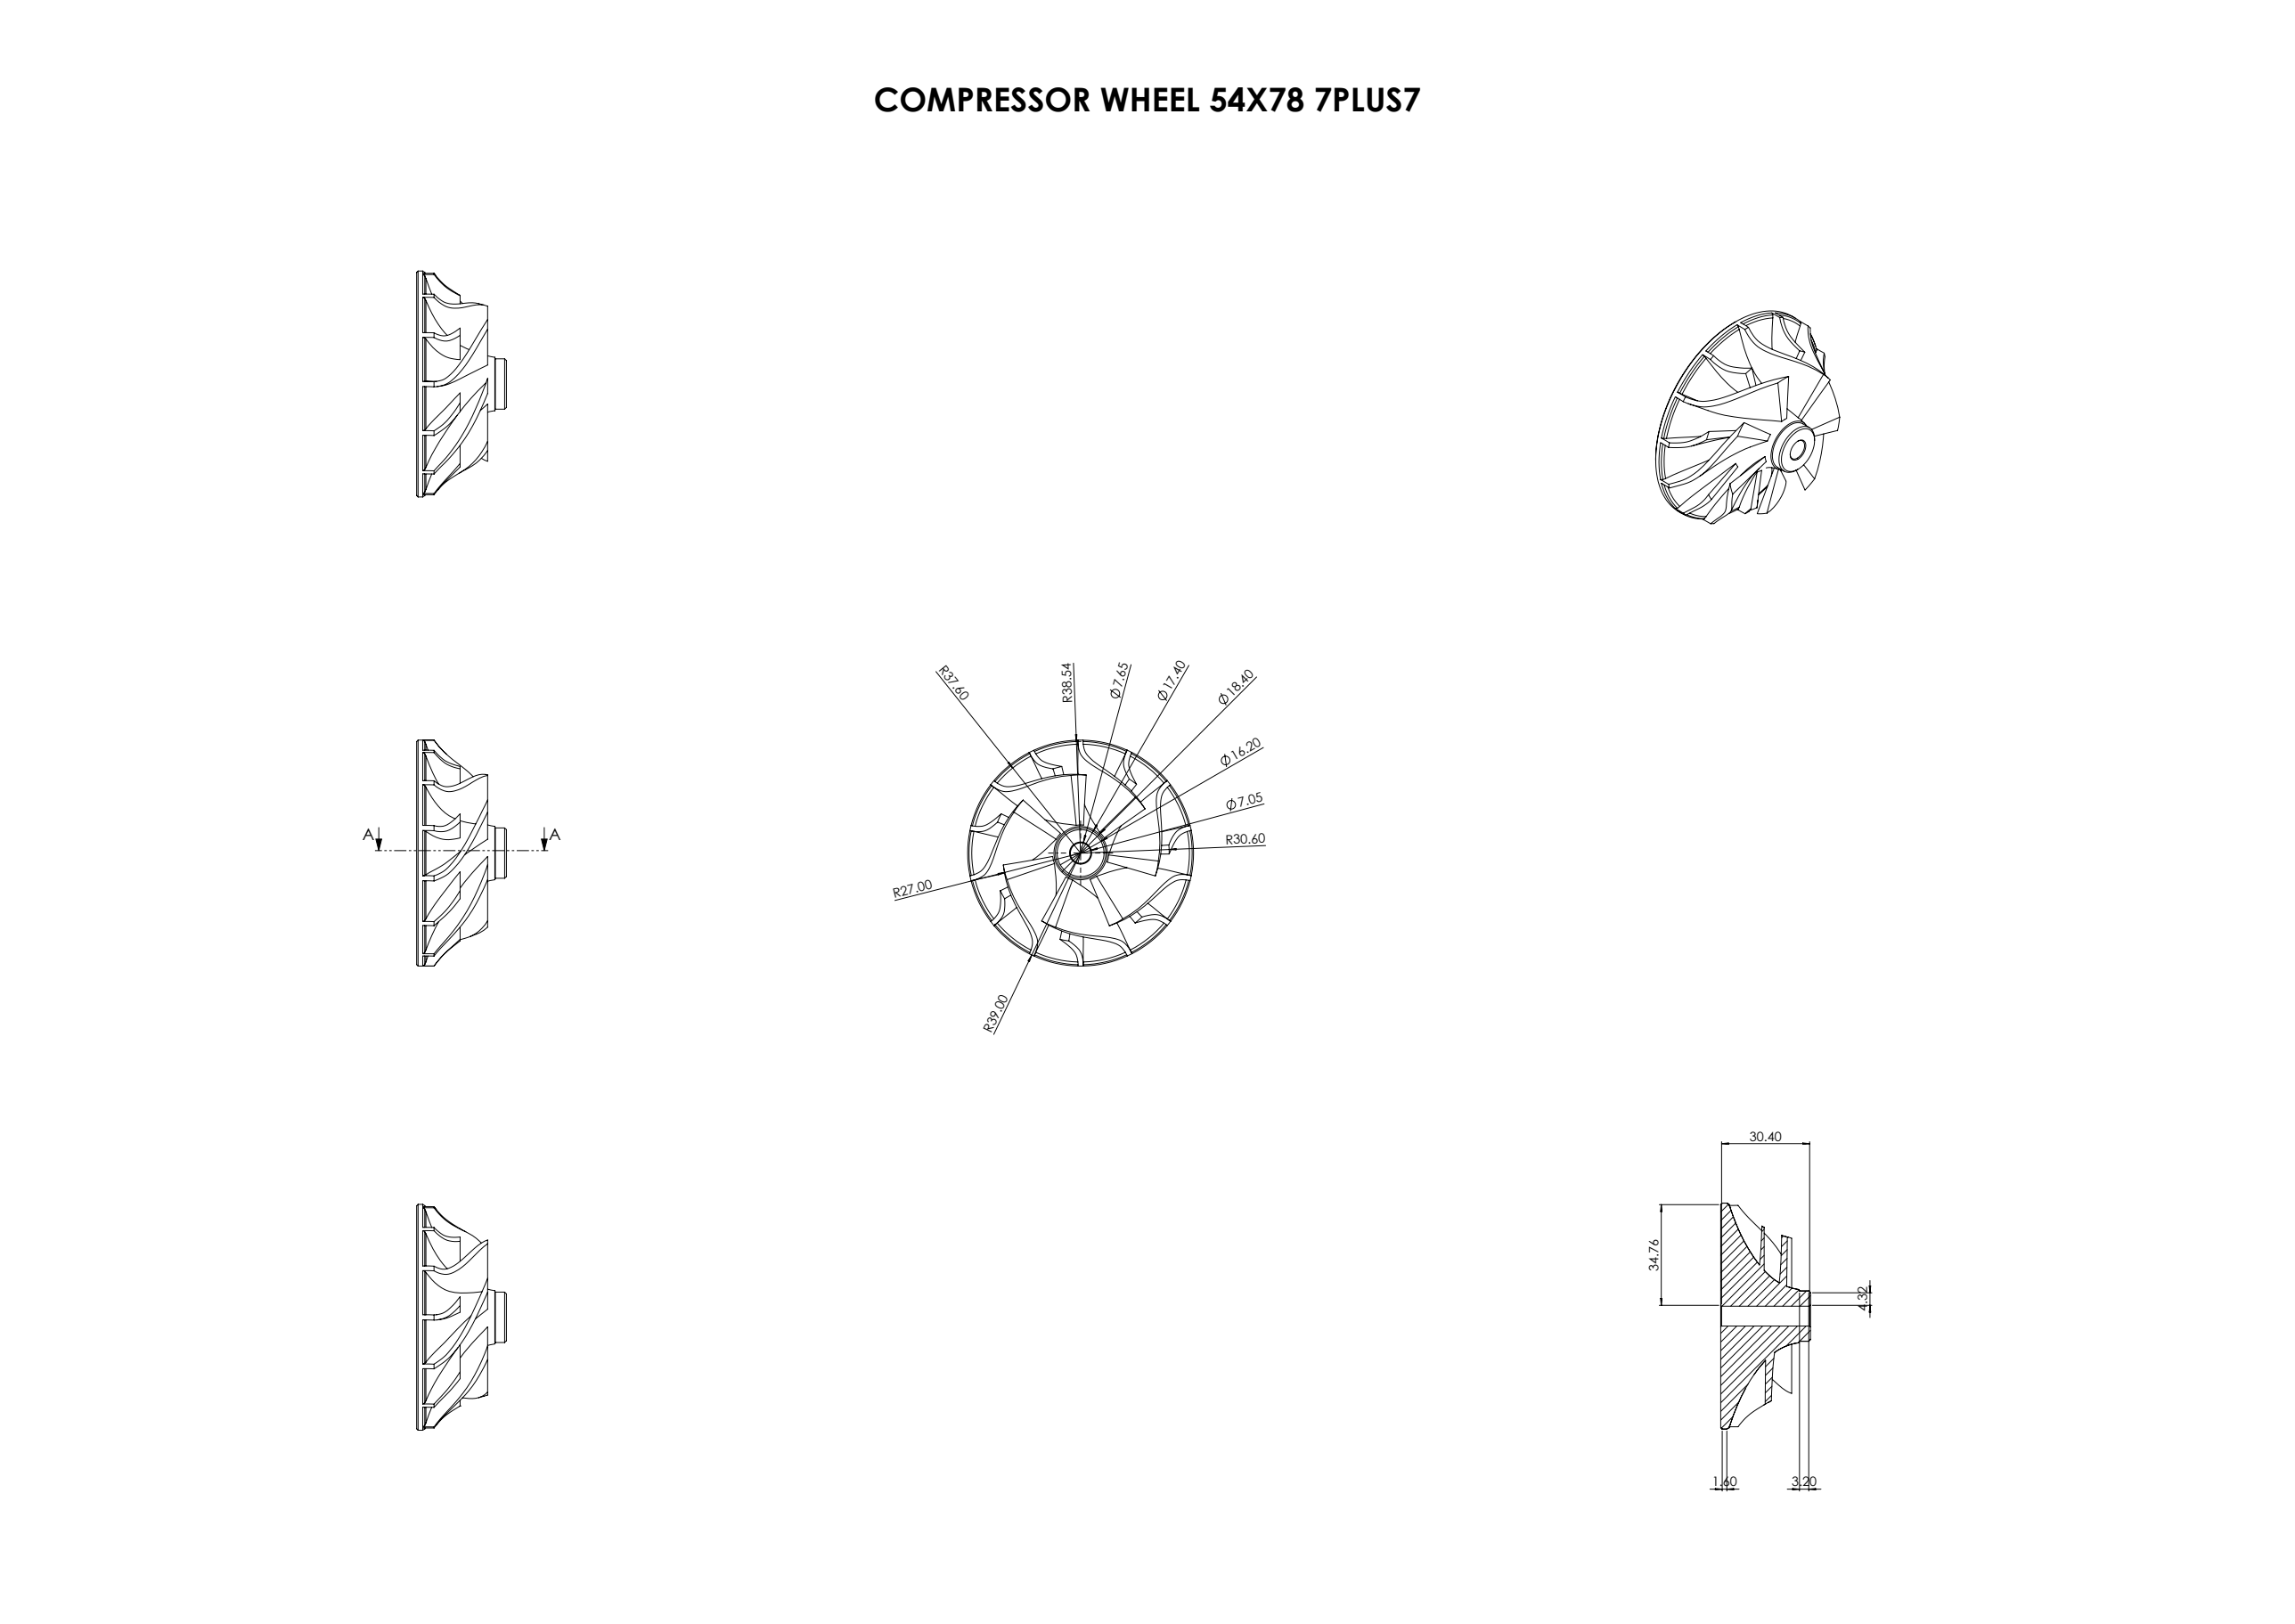
ISO-10303-21;
HEADER;
/* Generated by software containing ST-Developer
 * from STEP Tools, Inc. (www.steptools.com) 
 */

FILE_DESCRIPTION(
/* description */ (''),
/* implementation_level */ '2;1');

FILE_NAME(
/* name */ '09_Compressor_Wheel_54x78_7plus7.step',
/* time_stamp */ '2026-10-25T01:10:36-07:00',
/* author */ (''),
/* organization */ (''),
/* preprocessor_version */ 'ST-DEVELOPER v20.2',
/* originating_system */ 'Autodesk Translation Framework v15.15.0.0',
/* authorisation */ '');

FILE_SCHEMA (('AUTOMOTIVE_DESIGN { 1 0 10303 214 3 1 1 }'));
ENDSEC;

DATA;
#10=MECHANICAL_DESIGN_GEOMETRIC_PRESENTATION_REPRESENTATION('',(#1301),#60365);
#73=SHAPE_REPRESENTATION_RELATIONSHIP('SRR','None',#60413,#83);
#83=ADVANCED_BREP_SHAPE_REPRESENTATION('',(#93),#60361);
#93=MANIFOLD_SOLID_BREP('Body1',#18303);
#131=B_SPLINE_SURFACE_WITH_KNOTS('',3,3,((#48070,#48071,#48072,#48073,#48074,
#48075,#48076,#48077,#48078,#48079,#48080,#48081,#48082,#48083,#48084,#48085,
#48086,#48087,#48088,#48089,#48090,#48091,#48092,#48093,#48094,#48095,#48096),
(#48097,#48098,#48099,#48100,#48101,#48102,#48103,#48104,#48105,#48106,
#48107,#48108,#48109,#48110,#48111,#48112,#48113,#48114,#48115,#48116,#48117,
#48118,#48119,#48120,#48121,#48122,#48123),(#48124,#48125,#48126,#48127,
#48128,#48129,#48130,#48131,#48132,#48133,#48134,#48135,#48136,#48137,#48138,
#48139,#48140,#48141,#48142,#48143,#48144,#48145,#48146,#48147,#48148,#48149,
#48150),(#48151,#48152,#48153,#48154,#48155,#48156,#48157,#48158,#48159,
#48160,#48161,#48162,#48163,#48164,#48165,#48166,#48167,#48168,#48169,#48170,
#48171,#48172,#48173,#48174,#48175,#48176,#48177)),.UNSPECIFIED.,.F.,.F.,
 .F.,(4,4),(4,2,1,1,1,2,1,1,1,1,1,1,2,1,1,1,1,1,2,1,4),(0.266176291422809,
0.969386396335851),(0.0275328340336186,0.114720141806747,0.131928163077759,
0.149136184348771,0.183552226890795,0.252384311974843,0.26119115197838,
0.269997991981918,0.287611671988993,0.305225351996068,0.322839032003143,
0.358066392017293,0.393293752031443,0.516081621889917,0.536546266866329,
0.546778589354535,0.551894750598638,0.55445283122069,0.557010911842741,
0.604124367076873,0.651237822311005),.UNSPECIFIED.);
#132=B_SPLINE_SURFACE_WITH_KNOTS('',3,3,((#48414,#48415,#48416,#48417,#48418,
#48419,#48420,#48421,#48422,#48423,#48424,#48425,#48426,#48427,#48428,#48429,
#48430,#48431,#48432,#48433,#48434,#48435,#48436,#48437,#48438),(#48439,
#48440,#48441,#48442,#48443,#48444,#48445,#48446,#48447,#48448,#48449,#48450,
#48451,#48452,#48453,#48454,#48455,#48456,#48457,#48458,#48459,#48460,#48461,
#48462,#48463),(#48464,#48465,#48466,#48467,#48468,#48469,#48470,#48471,
#48472,#48473,#48474,#48475,#48476,#48477,#48478,#48479,#48480,#48481,#48482,
#48483,#48484,#48485,#48486,#48487,#48488),(#48489,#48490,#48491,#48492,
#48493,#48494,#48495,#48496,#48497,#48498,#48499,#48500,#48501,#48502,#48503,
#48504,#48505,#48506,#48507,#48508,#48509,#48510,#48511,#48512,#48513)),
 .UNSPECIFIED.,.F.,.F.,.F.,(4,4),(4,2,1,1,2,1,1,1,1,1,1,2,1,1,1,2,1,1,4),
(0.266100373933286,0.969385828517312),(0.0275328340336185,0.114720141806747,
0.149136184348771,0.183552226890795,0.252384311974843,0.26119115197838,
0.269997991981918,0.287611671988993,0.305225351996068,0.322839032003143,
0.340452712010218,0.393293752031443,0.475152331937092,0.516081621889917,
0.536546266866329,0.557010911842741,0.602472788890741,0.647934665938741,
0.738858420034741),.UNSPECIFIED.);
#133=B_SPLINE_SURFACE_WITH_KNOTS('',3,3,((#48540,#48541,#48542,#48543,#48544,
#48545,#48546,#48547,#48548,#48549,#48550,#48551,#48552,#48553,#48554,#48555,
#48556,#48557,#48558,#48559,#48560,#48561,#48562,#48563,#48564,#48565,#48566),
(#48567,#48568,#48569,#48570,#48571,#48572,#48573,#48574,#48575,#48576,
#48577,#48578,#48579,#48580,#48581,#48582,#48583,#48584,#48585,#48586,#48587,
#48588,#48589,#48590,#48591,#48592,#48593),(#48594,#48595,#48596,#48597,
#48598,#48599,#48600,#48601,#48602,#48603,#48604,#48605,#48606,#48607,#48608,
#48609,#48610,#48611,#48612,#48613,#48614,#48615,#48616,#48617,#48618,#48619,
#48620),(#48621,#48622,#48623,#48624,#48625,#48626,#48627,#48628,#48629,
#48630,#48631,#48632,#48633,#48634,#48635,#48636,#48637,#48638,#48639,#48640,
#48641,#48642,#48643,#48644,#48645,#48646,#48647)),.UNSPECIFIED.,.F.,.F.,
 .F.,(4,4),(4,2,1,1,1,2,1,1,1,1,1,1,2,1,1,1,1,1,2,1,4),(0.266176291422809,
0.969386396335851),(0.0275328340336186,0.114720141806747,0.131928163077759,
0.149136184348771,0.183552226890795,0.252384311974843,0.26119115197838,
0.269997991981918,0.287611671988993,0.305225351996068,0.322839032003143,
0.358066392017293,0.393293752031443,0.516081621889917,0.536546266866329,
0.546778589354535,0.551894750598638,0.55445283122069,0.557010911842741,
0.604124367076873,0.651237822311005),.UNSPECIFIED.);
#134=B_SPLINE_SURFACE_WITH_KNOTS('',3,3,((#48884,#48885,#48886,#48887,#48888,
#48889,#48890,#48891,#48892,#48893,#48894,#48895,#48896,#48897,#48898,#48899,
#48900,#48901,#48902,#48903,#48904,#48905,#48906,#48907,#48908),(#48909,
#48910,#48911,#48912,#48913,#48914,#48915,#48916,#48917,#48918,#48919,#48920,
#48921,#48922,#48923,#48924,#48925,#48926,#48927,#48928,#48929,#48930,#48931,
#48932,#48933),(#48934,#48935,#48936,#48937,#48938,#48939,#48940,#48941,
#48942,#48943,#48944,#48945,#48946,#48947,#48948,#48949,#48950,#48951,#48952,
#48953,#48954,#48955,#48956,#48957,#48958),(#48959,#48960,#48961,#48962,
#48963,#48964,#48965,#48966,#48967,#48968,#48969,#48970,#48971,#48972,#48973,
#48974,#48975,#48976,#48977,#48978,#48979,#48980,#48981,#48982,#48983)),
 .UNSPECIFIED.,.F.,.F.,.F.,(4,4),(4,2,1,1,2,1,1,1,1,1,1,2,1,1,1,2,1,1,4),
(0.266100373933286,0.969385828517312),(0.0275328340336192,0.114720141806747,
0.149136184348771,0.183552226890795,0.252384311974843,0.26119115197838,
0.269997991981918,0.287611671988993,0.305225351996068,0.322839032003143,
0.340452712010218,0.393293752031443,0.475152331937092,0.516081621889917,
0.536546266866329,0.557010911842741,0.602472788890741,0.647934665938741,
0.738858420034741),.UNSPECIFIED.);
#135=B_SPLINE_SURFACE_WITH_KNOTS('',3,3,((#49010,#49011,#49012,#49013,#49014,
#49015,#49016,#49017,#49018,#49019,#49020,#49021,#49022,#49023,#49024,#49025,
#49026,#49027,#49028,#49029,#49030,#49031,#49032,#49033,#49034,#49035,#49036),
(#49037,#49038,#49039,#49040,#49041,#49042,#49043,#49044,#49045,#49046,
#49047,#49048,#49049,#49050,#49051,#49052,#49053,#49054,#49055,#49056,#49057,
#49058,#49059,#49060,#49061,#49062,#49063),(#49064,#49065,#49066,#49067,
#49068,#49069,#49070,#49071,#49072,#49073,#49074,#49075,#49076,#49077,#49078,
#49079,#49080,#49081,#49082,#49083,#49084,#49085,#49086,#49087,#49088,#49089,
#49090),(#49091,#49092,#49093,#49094,#49095,#49096,#49097,#49098,#49099,
#49100,#49101,#49102,#49103,#49104,#49105,#49106,#49107,#49108,#49109,#49110,
#49111,#49112,#49113,#49114,#49115,#49116,#49117)),.UNSPECIFIED.,.F.,.F.,
 .F.,(4,4),(4,2,1,1,1,2,1,1,1,1,1,1,2,1,1,1,1,1,2,1,4),(0.266176291422809,
0.969386396335851),(0.0275328340336192,0.114720141806747,0.131928163077759,
0.149136184348771,0.183552226890795,0.252384311974843,0.26119115197838,
0.269997991981918,0.287611671988993,0.305225351996068,0.322839032003143,
0.358066392017293,0.393293752031443,0.516081621889917,0.536546266866329,
0.546778589354535,0.551894750598638,0.55445283122069,0.557010911842741,
0.604124367076873,0.651237822311005),.UNSPECIFIED.);
#136=B_SPLINE_SURFACE_WITH_KNOTS('',3,3,((#49354,#49355,#49356,#49357,#49358,
#49359,#49360,#49361,#49362,#49363,#49364,#49365,#49366,#49367,#49368,#49369,
#49370,#49371,#49372,#49373,#49374,#49375,#49376,#49377,#49378),(#49379,
#49380,#49381,#49382,#49383,#49384,#49385,#49386,#49387,#49388,#49389,#49390,
#49391,#49392,#49393,#49394,#49395,#49396,#49397,#49398,#49399,#49400,#49401,
#49402,#49403),(#49404,#49405,#49406,#49407,#49408,#49409,#49410,#49411,
#49412,#49413,#49414,#49415,#49416,#49417,#49418,#49419,#49420,#49421,#49422,
#49423,#49424,#49425,#49426,#49427,#49428),(#49429,#49430,#49431,#49432,
#49433,#49434,#49435,#49436,#49437,#49438,#49439,#49440,#49441,#49442,#49443,
#49444,#49445,#49446,#49447,#49448,#49449,#49450,#49451,#49452,#49453)),
 .UNSPECIFIED.,.F.,.F.,.F.,(4,4),(4,2,1,1,2,1,1,1,1,1,1,2,1,1,1,2,1,1,4),
(0.266100373933287,0.969385828517312),(0.0275328340336187,0.114720141806747,
0.149136184348771,0.183552226890795,0.252384311974843,0.26119115197838,
0.269997991981918,0.287611671988993,0.305225351996068,0.322839032003143,
0.340452712010218,0.393293752031443,0.475152331937092,0.516081621889917,
0.536546266866329,0.557010911842741,0.602472788890741,0.647934665938741,
0.738858420034741),.UNSPECIFIED.);
#137=B_SPLINE_SURFACE_WITH_KNOTS('',3,3,((#49480,#49481,#49482,#49483,#49484,
#49485,#49486,#49487,#49488,#49489,#49490,#49491,#49492,#49493,#49494,#49495,
#49496,#49497,#49498,#49499,#49500,#49501,#49502,#49503,#49504,#49505,#49506),
(#49507,#49508,#49509,#49510,#49511,#49512,#49513,#49514,#49515,#49516,
#49517,#49518,#49519,#49520,#49521,#49522,#49523,#49524,#49525,#49526,#49527,
#49528,#49529,#49530,#49531,#49532,#49533),(#49534,#49535,#49536,#49537,
#49538,#49539,#49540,#49541,#49542,#49543,#49544,#49545,#49546,#49547,#49548,
#49549,#49550,#49551,#49552,#49553,#49554,#49555,#49556,#49557,#49558,#49559,
#49560),(#49561,#49562,#49563,#49564,#49565,#49566,#49567,#49568,#49569,
#49570,#49571,#49572,#49573,#49574,#49575,#49576,#49577,#49578,#49579,#49580,
#49581,#49582,#49583,#49584,#49585,#49586,#49587)),.UNSPECIFIED.,.F.,.F.,
 .F.,(4,4),(4,2,1,1,1,2,1,1,1,1,1,1,2,1,1,1,1,1,2,1,4),(0.266176291422809,
0.969386396335851),(0.0275328340336192,0.114720141806747,0.131928163077759,
0.149136184348771,0.183552226890795,0.252384311974843,0.26119115197838,
0.269997991981918,0.287611671988993,0.305225351996068,0.322839032003143,
0.358066392017293,0.393293752031443,0.516081621889917,0.536546266866329,
0.546778589354535,0.551894750598638,0.55445283122069,0.557010911842741,
0.604124367076873,0.651237822311005),.UNSPECIFIED.);
#138=B_SPLINE_SURFACE_WITH_KNOTS('',3,3,((#49826,#49827,#49828,#49829,#49830,
#49831,#49832,#49833,#49834,#49835,#49836,#49837,#49838,#49839,#49840,#49841,
#49842,#49843,#49844,#49845,#49846,#49847,#49848,#49849,#49850),(#49851,
#49852,#49853,#49854,#49855,#49856,#49857,#49858,#49859,#49860,#49861,#49862,
#49863,#49864,#49865,#49866,#49867,#49868,#49869,#49870,#49871,#49872,#49873,
#49874,#49875),(#49876,#49877,#49878,#49879,#49880,#49881,#49882,#49883,
#49884,#49885,#49886,#49887,#49888,#49889,#49890,#49891,#49892,#49893,#49894,
#49895,#49896,#49897,#49898,#49899,#49900),(#49901,#49902,#49903,#49904,
#49905,#49906,#49907,#49908,#49909,#49910,#49911,#49912,#49913,#49914,#49915,
#49916,#49917,#49918,#49919,#49920,#49921,#49922,#49923,#49924,#49925)),
 .UNSPECIFIED.,.F.,.F.,.F.,(4,4),(4,2,1,1,2,1,1,1,1,1,1,2,1,1,1,2,1,1,4),
(0.266100373933287,0.969385828517312),(0.0275328340336186,0.114720141806747,
0.149136184348771,0.183552226890795,0.252384311974843,0.26119115197838,
0.269997991981918,0.287611671988993,0.305225351996068,0.322839032003143,
0.340452712010218,0.393293752031443,0.475152331937092,0.516081621889917,
0.536546266866329,0.557010911842741,0.602472788890741,0.647934665938741,
0.738858420034741),.UNSPECIFIED.);
#139=B_SPLINE_SURFACE_WITH_KNOTS('',3,3,((#49952,#49953,#49954,#49955,#49956,
#49957,#49958,#49959,#49960,#49961,#49962,#49963,#49964,#49965,#49966,#49967,
#49968,#49969,#49970,#49971,#49972,#49973,#49974,#49975,#49976,#49977,#49978),
(#49979,#49980,#49981,#49982,#49983,#49984,#49985,#49986,#49987,#49988,
#49989,#49990,#49991,#49992,#49993,#49994,#49995,#49996,#49997,#49998,#49999,
#50000,#50001,#50002,#50003,#50004,#50005),(#50006,#50007,#50008,#50009,
#50010,#50011,#50012,#50013,#50014,#50015,#50016,#50017,#50018,#50019,#50020,
#50021,#50022,#50023,#50024,#50025,#50026,#50027,#50028,#50029,#50030,#50031,
#50032),(#50033,#50034,#50035,#50036,#50037,#50038,#50039,#50040,#50041,
#50042,#50043,#50044,#50045,#50046,#50047,#50048,#50049,#50050,#50051,#50052,
#50053,#50054,#50055,#50056,#50057,#50058,#50059)),.UNSPECIFIED.,.F.,.F.,
 .F.,(4,4),(4,2,1,1,1,2,1,1,1,1,1,1,2,1,1,1,1,1,2,1,4),(0.266176291422809,
0.969386396335851),(0.0275328340336195,0.114720141806747,0.131928163077759,
0.149136184348771,0.183552226890795,0.252384311974843,0.26119115197838,
0.269997991981918,0.287611671988993,0.305225351996068,0.322839032003143,
0.358066392017293,0.393293752031443,0.516081621889917,0.536546266866329,
0.546778589354535,0.551894750598638,0.55445283122069,0.557010911842741,
0.604124367076873,0.651237822311005),.UNSPECIFIED.);
#140=B_SPLINE_SURFACE_WITH_KNOTS('',3,3,((#50298,#50299,#50300,#50301,#50302,
#50303,#50304,#50305,#50306,#50307,#50308,#50309,#50310,#50311,#50312,#50313,
#50314,#50315,#50316,#50317,#50318,#50319,#50320,#50321,#50322),(#50323,
#50324,#50325,#50326,#50327,#50328,#50329,#50330,#50331,#50332,#50333,#50334,
#50335,#50336,#50337,#50338,#50339,#50340,#50341,#50342,#50343,#50344,#50345,
#50346,#50347),(#50348,#50349,#50350,#50351,#50352,#50353,#50354,#50355,
#50356,#50357,#50358,#50359,#50360,#50361,#50362,#50363,#50364,#50365,#50366,
#50367,#50368,#50369,#50370,#50371,#50372),(#50373,#50374,#50375,#50376,
#50377,#50378,#50379,#50380,#50381,#50382,#50383,#50384,#50385,#50386,#50387,
#50388,#50389,#50390,#50391,#50392,#50393,#50394,#50395,#50396,#50397)),
 .UNSPECIFIED.,.F.,.F.,.F.,(4,4),(4,2,1,1,2,1,1,1,1,1,1,2,1,1,1,2,1,1,4),
(0.266100373933287,0.969385828517312),(0.0275328340336187,0.114720141806747,
0.149136184348771,0.183552226890795,0.252384311974843,0.26119115197838,
0.269997991981918,0.287611671988993,0.305225351996068,0.322839032003143,
0.340452712010218,0.393293752031443,0.475152331937092,0.516081621889917,
0.536546266866329,0.557010911842741,0.602472788890741,0.647934665938741,
0.738858420034741),.UNSPECIFIED.);
#141=B_SPLINE_SURFACE_WITH_KNOTS('',3,3,((#50424,#50425,#50426,#50427,#50428,
#50429,#50430,#50431,#50432,#50433,#50434,#50435,#50436,#50437,#50438,#50439,
#50440,#50441,#50442,#50443,#50444,#50445,#50446,#50447,#50448,#50449,#50450),
(#50451,#50452,#50453,#50454,#50455,#50456,#50457,#50458,#50459,#50460,
#50461,#50462,#50463,#50464,#50465,#50466,#50467,#50468,#50469,#50470,#50471,
#50472,#50473,#50474,#50475,#50476,#50477),(#50478,#50479,#50480,#50481,
#50482,#50483,#50484,#50485,#50486,#50487,#50488,#50489,#50490,#50491,#50492,
#50493,#50494,#50495,#50496,#50497,#50498,#50499,#50500,#50501,#50502,#50503,
#50504),(#50505,#50506,#50507,#50508,#50509,#50510,#50511,#50512,#50513,
#50514,#50515,#50516,#50517,#50518,#50519,#50520,#50521,#50522,#50523,#50524,
#50525,#50526,#50527,#50528,#50529,#50530,#50531)),.UNSPECIFIED.,.F.,.F.,
 .F.,(4,4),(4,2,1,1,1,2,1,1,1,1,1,1,2,1,1,1,1,1,2,1,4),(0.266176291422809,
0.969386396335851),(0.0275328340336193,0.114720141806747,0.131928163077759,
0.149136184348771,0.183552226890795,0.252384311974843,0.26119115197838,
0.269997991981918,0.287611671988993,0.305225351996068,0.322839032003143,
0.358066392017293,0.393293752031443,0.516081621889917,0.536546266866329,
0.546778589354535,0.551894750598638,0.55445283122069,0.557010911842741,
0.604124367076873,0.651237822311005),.UNSPECIFIED.);
#142=B_SPLINE_SURFACE_WITH_KNOTS('',3,3,((#50768,#50769,#50770,#50771,#50772,
#50773,#50774,#50775,#50776,#50777,#50778,#50779,#50780,#50781,#50782,#50783,
#50784,#50785,#50786,#50787,#50788,#50789,#50790,#50791,#50792),(#50793,
#50794,#50795,#50796,#50797,#50798,#50799,#50800,#50801,#50802,#50803,#50804,
#50805,#50806,#50807,#50808,#50809,#50810,#50811,#50812,#50813,#50814,#50815,
#50816,#50817),(#50818,#50819,#50820,#50821,#50822,#50823,#50824,#50825,
#50826,#50827,#50828,#50829,#50830,#50831,#50832,#50833,#50834,#50835,#50836,
#50837,#50838,#50839,#50840,#50841,#50842),(#50843,#50844,#50845,#50846,
#50847,#50848,#50849,#50850,#50851,#50852,#50853,#50854,#50855,#50856,#50857,
#50858,#50859,#50860,#50861,#50862,#50863,#50864,#50865,#50866,#50867)),
 .UNSPECIFIED.,.F.,.F.,.F.,(4,4),(4,2,1,1,2,1,1,1,1,1,1,2,1,1,1,2,1,1,4),
(0.266100373933286,0.969385828517312),(0.0275328340336187,0.114720141806747,
0.149136184348771,0.183552226890795,0.252384311974843,0.26119115197838,
0.269997991981918,0.287611671988993,0.305225351996068,0.322839032003143,
0.340452712010218,0.393293752031443,0.475152331937092,0.516081621889917,
0.536546266866329,0.557010911842741,0.602472788890741,0.647934665938741,
0.738858420034741),.UNSPECIFIED.);
#143=B_SPLINE_SURFACE_WITH_KNOTS('',3,3,((#50894,#50895,#50896,#50897,#50898,
#50899,#50900,#50901,#50902,#50903,#50904,#50905,#50906,#50907,#50908,#50909,
#50910,#50911,#50912,#50913,#50914,#50915,#50916,#50917,#50918,#50919,#50920),
(#50921,#50922,#50923,#50924,#50925,#50926,#50927,#50928,#50929,#50930,
#50931,#50932,#50933,#50934,#50935,#50936,#50937,#50938,#50939,#50940,#50941,
#50942,#50943,#50944,#50945,#50946,#50947),(#50948,#50949,#50950,#50951,
#50952,#50953,#50954,#50955,#50956,#50957,#50958,#50959,#50960,#50961,#50962,
#50963,#50964,#50965,#50966,#50967,#50968,#50969,#50970,#50971,#50972,#50973,
#50974),(#50975,#50976,#50977,#50978,#50979,#50980,#50981,#50982,#50983,
#50984,#50985,#50986,#50987,#50988,#50989,#50990,#50991,#50992,#50993,#50994,
#50995,#50996,#50997,#50998,#50999,#51000,#51001)),.UNSPECIFIED.,.F.,.F.,
 .F.,(4,4),(4,2,1,1,1,2,1,1,1,1,1,1,2,1,1,1,1,1,2,1,4),(0.266176291422809,
0.969386396335851),(0.0275328340336186,0.114720141806747,0.131928163077759,
0.149136184348771,0.183552226890795,0.252384311974843,0.26119115197838,
0.269997991981918,0.287611671988993,0.305225351996068,0.322839032003143,
0.358066392017293,0.393293752031443,0.516081621889917,0.536546266866329,
0.546778589354535,0.551894750598638,0.55445283122069,0.557010911842741,
0.604124367076873,0.651237822311005),.UNSPECIFIED.);
#144=B_SPLINE_SURFACE_WITH_KNOTS('',3,3,((#51203,#51204,#51205,#51206,#51207,
#51208,#51209,#51210,#51211,#51212,#51213,#51214,#51215,#51216,#51217,#51218,
#51219,#51220,#51221,#51222,#51223,#51224,#51225,#51226,#51227),(#51228,
#51229,#51230,#51231,#51232,#51233,#51234,#51235,#51236,#51237,#51238,#51239,
#51240,#51241,#51242,#51243,#51244,#51245,#51246,#51247,#51248,#51249,#51250,
#51251,#51252),(#51253,#51254,#51255,#51256,#51257,#51258,#51259,#51260,
#51261,#51262,#51263,#51264,#51265,#51266,#51267,#51268,#51269,#51270,#51271,
#51272,#51273,#51274,#51275,#51276,#51277),(#51278,#51279,#51280,#51281,
#51282,#51283,#51284,#51285,#51286,#51287,#51288,#51289,#51290,#51291,#51292,
#51293,#51294,#51295,#51296,#51297,#51298,#51299,#51300,#51301,#51302)),
 .UNSPECIFIED.,.F.,.F.,.F.,(4,4),(4,2,1,1,2,1,1,1,1,1,1,2,1,1,1,2,1,1,4),
(0.266100373933287,0.969385828517312),(0.0275328340336187,0.114720141806747,
0.149136184348771,0.183552226890795,0.252384311974843,0.26119115197838,
0.269997991981918,0.287611671988993,0.305225351996068,0.322839032003143,
0.340452712010218,0.393293752031443,0.475152331937092,0.516081621889917,
0.536546266866329,0.557010911842741,0.602472788890741,0.647934665938741,
0.738858420034741),.UNSPECIFIED.);
#145=B_SPLINE_SURFACE_WITH_KNOTS('',3,3,((#51312,#51313,#51314,#51315,#51316,
#51317,#51318,#51319,#51320,#51321,#51322,#51323,#51324,#51325,#51326,#51327,
#51328,#51329,#51330,#51331,#51332,#51333,#51334,#51335,#51336,#51337,#51338,
#51339,#51340,#51341,#51342,#51343,#51344,#51345,#51346),(#51347,#51348,
#51349,#51350,#51351,#51352,#51353,#51354,#51355,#51356,#51357,#51358,#51359,
#51360,#51361,#51362,#51363,#51364,#51365,#51366,#51367,#51368,#51369,#51370,
#51371,#51372,#51373,#51374,#51375,#51376,#51377,#51378,#51379,#51380,#51381),
(#51382,#51383,#51384,#51385,#51386,#51387,#51388,#51389,#51390,#51391,
#51392,#51393,#51394,#51395,#51396,#51397,#51398,#51399,#51400,#51401,#51402,
#51403,#51404,#51405,#51406,#51407,#51408,#51409,#51410,#51411,#51412,#51413,
#51414,#51415,#51416),(#51417,#51418,#51419,#51420,#51421,#51422,#51423,
#51424,#51425,#51426,#51427,#51428,#51429,#51430,#51431,#51432,#51433,#51434,
#51435,#51436,#51437,#51438,#51439,#51440,#51441,#51442,#51443,#51444,#51445,
#51446,#51447,#51448,#51449,#51450,#51451),(#51452,#51453,#51454,#51455,
#51456,#51457,#51458,#51459,#51460,#51461,#51462,#51463,#51464,#51465,#51466,
#51467,#51468,#51469,#51470,#51471,#51472,#51473,#51474,#51475,#51476,#51477,
#51478,#51479,#51480,#51481,#51482,#51483,#51484,#51485,#51486)),
 .UNSPECIFIED.,.F.,.F.,.F.,(4,1,4),(4,2,1,1,1,2,1,1,1,1,1,1,1,2,1,2,1,1,
2,1,1,2,1,1,2,4),(0.081890721945263,0.462246010974744,0.969386396347385),
(0.0162979902041911,0.0679082925174644,0.0780945363950841,0.0882807802727037,
0.108653268027943,0.149398243538422,0.154611429799316,0.159824616060209,
0.165037802321103,0.170250988581997,0.191103733625573,0.211956478669149,
0.222382851190937,0.232809223712724,0.281265199287278,0.329721174861832,
0.35931187583389,0.388902576805948,0.448083978750065,0.484049840267495,
0.520015701784926,0.591947424819786,0.634833203943942,0.677718983068097,
0.763490541316409,0.884888589856318),.UNSPECIFIED.);
#146=B_SPLINE_SURFACE_WITH_KNOTS('',3,3,((#51895,#51896,#51897,#51898,#51899,
#51900,#51901,#51902,#51903,#51904,#51905,#51906,#51907,#51908,#51909,#51910,
#51911,#51912,#51913,#51914,#51915,#51916,#51917,#51918,#51919,#51920,#51921,
#51922,#51923,#51924,#51925,#51926,#51927,#51928,#51929,#51930),(#51931,
#51932,#51933,#51934,#51935,#51936,#51937,#51938,#51939,#51940,#51941,#51942,
#51943,#51944,#51945,#51946,#51947,#51948,#51949,#51950,#51951,#51952,#51953,
#51954,#51955,#51956,#51957,#51958,#51959,#51960,#51961,#51962,#51963,#51964,
#51965,#51966),(#51967,#51968,#51969,#51970,#51971,#51972,#51973,#51974,
#51975,#51976,#51977,#51978,#51979,#51980,#51981,#51982,#51983,#51984,#51985,
#51986,#51987,#51988,#51989,#51990,#51991,#51992,#51993,#51994,#51995,#51996,
#51997,#51998,#51999,#52000,#52001,#52002),(#52003,#52004,#52005,#52006,
#52007,#52008,#52009,#52010,#52011,#52012,#52013,#52014,#52015,#52016,#52017,
#52018,#52019,#52020,#52021,#52022,#52023,#52024,#52025,#52026,#52027,#52028,
#52029,#52030,#52031,#52032,#52033,#52034,#52035,#52036,#52037,#52038),
(#52039,#52040,#52041,#52042,#52043,#52044,#52045,#52046,#52047,#52048,
#52049,#52050,#52051,#52052,#52053,#52054,#52055,#52056,#52057,#52058,#52059,
#52060,#52061,#52062,#52063,#52064,#52065,#52066,#52067,#52068,#52069,#52070,
#52071,#52072,#52073,#52074)),.UNSPECIFIED.,.F.,.F.,.F.,(4,1,4),(4,2,1,
1,1,2,1,1,1,1,1,1,1,2,1,2,1,1,2,1,1,1,2,1,1,2,4),(0.081835747691657,0.462214353759979,
0.969385828517743),(0.0162979902041911,0.0679082925174644,0.0780945363950841,
0.0882807802727037,0.108653268027943,0.149398243538422,0.154611429799316,
0.159824616060209,0.165037802321103,0.170250988581997,0.191103733625573,
0.211956478669149,0.222382851190937,0.232809223712724,0.281265199287278,
0.329721174861832,0.35931187583389,0.388902576805948,0.448083978750065,
0.46606690950878,0.484049840267495,0.520015701784926,0.591947424819786,
0.634833203943942,0.677718983068097,0.763490541316409,0.988990749040375),
 .UNSPECIFIED.);
#147=B_SPLINE_SURFACE_WITH_KNOTS('',3,3,((#52134,#52135,#52136,#52137,#52138,
#52139,#52140,#52141,#52142,#52143,#52144,#52145,#52146,#52147,#52148,#52149,
#52150,#52151,#52152,#52153,#52154,#52155,#52156,#52157,#52158,#52159,#52160,
#52161,#52162,#52163,#52164,#52165,#52166,#52167,#52168),(#52169,#52170,
#52171,#52172,#52173,#52174,#52175,#52176,#52177,#52178,#52179,#52180,#52181,
#52182,#52183,#52184,#52185,#52186,#52187,#52188,#52189,#52190,#52191,#52192,
#52193,#52194,#52195,#52196,#52197,#52198,#52199,#52200,#52201,#52202,#52203),
(#52204,#52205,#52206,#52207,#52208,#52209,#52210,#52211,#52212,#52213,
#52214,#52215,#52216,#52217,#52218,#52219,#52220,#52221,#52222,#52223,#52224,
#52225,#52226,#52227,#52228,#52229,#52230,#52231,#52232,#52233,#52234,#52235,
#52236,#52237,#52238),(#52239,#52240,#52241,#52242,#52243,#52244,#52245,
#52246,#52247,#52248,#52249,#52250,#52251,#52252,#52253,#52254,#52255,#52256,
#52257,#52258,#52259,#52260,#52261,#52262,#52263,#52264,#52265,#52266,#52267,
#52268,#52269,#52270,#52271,#52272,#52273),(#52274,#52275,#52276,#52277,
#52278,#52279,#52280,#52281,#52282,#52283,#52284,#52285,#52286,#52287,#52288,
#52289,#52290,#52291,#52292,#52293,#52294,#52295,#52296,#52297,#52298,#52299,
#52300,#52301,#52302,#52303,#52304,#52305,#52306,#52307,#52308)),
 .UNSPECIFIED.,.F.,.F.,.F.,(4,1,4),(4,2,1,1,1,2,1,1,1,1,1,1,1,2,1,2,1,1,
2,1,1,2,1,1,2,4),(0.0818907219452629,0.462246010974744,0.969386396347385),
(0.0162979902041915,0.0679082925174644,0.0780945363950841,0.0882807802727037,
0.108653268027943,0.149398243538422,0.154611429799316,0.159824616060209,
0.165037802321103,0.170250988581997,0.191103733625573,0.211956478669149,
0.222382851190937,0.232809223712724,0.281265199287278,0.329721174861832,
0.35931187583389,0.388902576805948,0.448083978750065,0.484049840267495,
0.520015701784926,0.591947424819786,0.634833203943942,0.677718983068097,
0.763490541316409,0.884888589856318),.UNSPECIFIED.);
#148=B_SPLINE_SURFACE_WITH_KNOTS('',3,3,((#52717,#52718,#52719,#52720,#52721,
#52722,#52723,#52724,#52725,#52726,#52727,#52728,#52729,#52730,#52731,#52732,
#52733,#52734,#52735,#52736,#52737,#52738,#52739,#52740,#52741,#52742,#52743,
#52744,#52745,#52746,#52747,#52748,#52749,#52750,#52751),(#52752,#52753,
#52754,#52755,#52756,#52757,#52758,#52759,#52760,#52761,#52762,#52763,#52764,
#52765,#52766,#52767,#52768,#52769,#52770,#52771,#52772,#52773,#52774,#52775,
#52776,#52777,#52778,#52779,#52780,#52781,#52782,#52783,#52784,#52785,#52786),
(#52787,#52788,#52789,#52790,#52791,#52792,#52793,#52794,#52795,#52796,
#52797,#52798,#52799,#52800,#52801,#52802,#52803,#52804,#52805,#52806,#52807,
#52808,#52809,#52810,#52811,#52812,#52813,#52814,#52815,#52816,#52817,#52818,
#52819,#52820,#52821),(#52822,#52823,#52824,#52825,#52826,#52827,#52828,
#52829,#52830,#52831,#52832,#52833,#52834,#52835,#52836,#52837,#52838,#52839,
#52840,#52841,#52842,#52843,#52844,#52845,#52846,#52847,#52848,#52849,#52850,
#52851,#52852,#52853,#52854,#52855,#52856),(#52857,#52858,#52859,#52860,
#52861,#52862,#52863,#52864,#52865,#52866,#52867,#52868,#52869,#52870,#52871,
#52872,#52873,#52874,#52875,#52876,#52877,#52878,#52879,#52880,#52881,#52882,
#52883,#52884,#52885,#52886,#52887,#52888,#52889,#52890,#52891),(#52892,
#52893,#52894,#52895,#52896,#52897,#52898,#52899,#52900,#52901,#52902,#52903,
#52904,#52905,#52906,#52907,#52908,#52909,#52910,#52911,#52912,#52913,#52914,
#52915,#52916,#52917,#52918,#52919,#52920,#52921,#52922,#52923,#52924,#52925,
#52926)),.UNSPECIFIED.,.F.,.F.,.F.,(4,1,1,4),(4,2,1,1,1,2,1,1,1,1,1,1,2,
1,1,2,1,1,2,1,1,2,1,1,2,4),(0.0818357476916571,0.335421485070539,0.58900722244942,
0.969385828517743),(0.016297990204191,0.0679082925174644,0.0780945363950841,
0.0882807802727037,0.108653268027943,0.149398243538422,0.154611429799316,
0.159824616060209,0.170250988581997,0.180677361103785,0.191103733625573,
0.211956478669149,0.232809223712724,0.281265199287278,0.305493187074555,
0.329721174861832,0.35931187583389,0.388902576805948,0.448083978750065,
0.484049840267495,0.520015701784926,0.591947424819786,0.634833203943942,
0.677718983068097,0.763490541316409,0.988990749040375),.UNSPECIFIED.);
#149=B_SPLINE_SURFACE_WITH_KNOTS('',3,3,((#52986,#52987,#52988,#52989,#52990,
#52991,#52992,#52993,#52994,#52995,#52996,#52997,#52998,#52999,#53000,#53001,
#53002,#53003,#53004,#53005,#53006,#53007,#53008,#53009,#53010,#53011,#53012,
#53013,#53014,#53015,#53016,#53017,#53018,#53019,#53020,#53021),(#53022,
#53023,#53024,#53025,#53026,#53027,#53028,#53029,#53030,#53031,#53032,#53033,
#53034,#53035,#53036,#53037,#53038,#53039,#53040,#53041,#53042,#53043,#53044,
#53045,#53046,#53047,#53048,#53049,#53050,#53051,#53052,#53053,#53054,#53055,
#53056,#53057),(#53058,#53059,#53060,#53061,#53062,#53063,#53064,#53065,
#53066,#53067,#53068,#53069,#53070,#53071,#53072,#53073,#53074,#53075,#53076,
#53077,#53078,#53079,#53080,#53081,#53082,#53083,#53084,#53085,#53086,#53087,
#53088,#53089,#53090,#53091,#53092,#53093),(#53094,#53095,#53096,#53097,
#53098,#53099,#53100,#53101,#53102,#53103,#53104,#53105,#53106,#53107,#53108,
#53109,#53110,#53111,#53112,#53113,#53114,#53115,#53116,#53117,#53118,#53119,
#53120,#53121,#53122,#53123,#53124,#53125,#53126,#53127,#53128,#53129),
(#53130,#53131,#53132,#53133,#53134,#53135,#53136,#53137,#53138,#53139,
#53140,#53141,#53142,#53143,#53144,#53145,#53146,#53147,#53148,#53149,#53150,
#53151,#53152,#53153,#53154,#53155,#53156,#53157,#53158,#53159,#53160,#53161,
#53162,#53163,#53164,#53165)),.UNSPECIFIED.,.F.,.F.,.F.,(4,1,4),(4,2,1,
1,1,2,1,1,1,1,1,1,1,2,1,2,1,1,2,1,1,1,2,1,1,2,4),(0.0818907219452629,0.462246010974744,
0.969386396347385),(0.0162979902041916,0.0679082925174644,0.0780945363950841,
0.0882807802727037,0.108653268027943,0.149398243538422,0.154611429799316,
0.159824616060209,0.165037802321103,0.170250988581997,0.191103733625573,
0.211956478669149,0.222382851190937,0.232809223712724,0.281265199287278,
0.329721174861832,0.35931187583389,0.388902576805948,0.448083978750065,
0.46606690950878,0.484049840267495,0.520015701784926,0.591947424819786,
0.634833203943942,0.677718983068097,0.763490541316409,0.884888589856318),
 .UNSPECIFIED.);
#150=B_SPLINE_SURFACE_WITH_KNOTS('',3,3,((#53574,#53575,#53576,#53577,#53578,
#53579,#53580,#53581,#53582,#53583,#53584,#53585,#53586,#53587,#53588,#53589,
#53590,#53591,#53592,#53593,#53594,#53595,#53596,#53597,#53598,#53599,#53600,
#53601,#53602,#53603,#53604,#53605,#53606,#53607,#53608),(#53609,#53610,
#53611,#53612,#53613,#53614,#53615,#53616,#53617,#53618,#53619,#53620,#53621,
#53622,#53623,#53624,#53625,#53626,#53627,#53628,#53629,#53630,#53631,#53632,
#53633,#53634,#53635,#53636,#53637,#53638,#53639,#53640,#53641,#53642,#53643),
(#53644,#53645,#53646,#53647,#53648,#53649,#53650,#53651,#53652,#53653,
#53654,#53655,#53656,#53657,#53658,#53659,#53660,#53661,#53662,#53663,#53664,
#53665,#53666,#53667,#53668,#53669,#53670,#53671,#53672,#53673,#53674,#53675,
#53676,#53677,#53678),(#53679,#53680,#53681,#53682,#53683,#53684,#53685,
#53686,#53687,#53688,#53689,#53690,#53691,#53692,#53693,#53694,#53695,#53696,
#53697,#53698,#53699,#53700,#53701,#53702,#53703,#53704,#53705,#53706,#53707,
#53708,#53709,#53710,#53711,#53712,#53713),(#53714,#53715,#53716,#53717,
#53718,#53719,#53720,#53721,#53722,#53723,#53724,#53725,#53726,#53727,#53728,
#53729,#53730,#53731,#53732,#53733,#53734,#53735,#53736,#53737,#53738,#53739,
#53740,#53741,#53742,#53743,#53744,#53745,#53746,#53747,#53748)),
 .UNSPECIFIED.,.F.,.F.,.F.,(4,1,4),(4,2,1,1,1,2,1,1,1,1,1,1,1,2,1,2,1,1,
2,1,1,2,1,1,2,4),(0.0818357476916571,0.462214353759979,0.969385828517743),
(0.0162979902041911,0.0679082925174644,0.0780945363950841,0.0882807802727037,
0.108653268027943,0.149398243538422,0.154611429799316,0.159824616060209,
0.165037802321103,0.170250988581997,0.191103733625573,0.211956478669149,
0.222382851190937,0.232809223712724,0.281265199287278,0.329721174861832,
0.35931187583389,0.388902576805948,0.448083978750065,0.484049840267495,
0.520015701784926,0.591947424819786,0.634833203943942,0.677718983068097,
0.763490541316409,0.988990749040375),.UNSPECIFIED.);
#151=B_SPLINE_SURFACE_WITH_KNOTS('',3,3,((#53808,#53809,#53810,#53811,#53812,
#53813,#53814,#53815,#53816,#53817,#53818,#53819,#53820,#53821,#53822,#53823,
#53824,#53825,#53826,#53827,#53828,#53829,#53830,#53831,#53832,#53833,#53834,
#53835,#53836,#53837,#53838,#53839,#53840,#53841,#53842),(#53843,#53844,
#53845,#53846,#53847,#53848,#53849,#53850,#53851,#53852,#53853,#53854,#53855,
#53856,#53857,#53858,#53859,#53860,#53861,#53862,#53863,#53864,#53865,#53866,
#53867,#53868,#53869,#53870,#53871,#53872,#53873,#53874,#53875,#53876,#53877),
(#53878,#53879,#53880,#53881,#53882,#53883,#53884,#53885,#53886,#53887,
#53888,#53889,#53890,#53891,#53892,#53893,#53894,#53895,#53896,#53897,#53898,
#53899,#53900,#53901,#53902,#53903,#53904,#53905,#53906,#53907,#53908,#53909,
#53910,#53911,#53912),(#53913,#53914,#53915,#53916,#53917,#53918,#53919,
#53920,#53921,#53922,#53923,#53924,#53925,#53926,#53927,#53928,#53929,#53930,
#53931,#53932,#53933,#53934,#53935,#53936,#53937,#53938,#53939,#53940,#53941,
#53942,#53943,#53944,#53945,#53946,#53947),(#53948,#53949,#53950,#53951,
#53952,#53953,#53954,#53955,#53956,#53957,#53958,#53959,#53960,#53961,#53962,
#53963,#53964,#53965,#53966,#53967,#53968,#53969,#53970,#53971,#53972,#53973,
#53974,#53975,#53976,#53977,#53978,#53979,#53980,#53981,#53982)),
 .UNSPECIFIED.,.F.,.F.,.F.,(4,1,4),(4,2,1,1,1,2,1,1,1,1,1,1,1,2,1,2,1,1,
2,1,1,2,1,1,2,4),(0.0818907219452629,0.462246010974744,0.969386396347385),
(0.0162979902041915,0.0679082925174644,0.0780945363950841,0.0882807802727037,
0.108653268027943,0.149398243538422,0.154611429799316,0.159824616060209,
0.165037802321103,0.170250988581997,0.191103733625573,0.211956478669149,
0.222382851190937,0.232809223712724,0.281265199287278,0.329721174861832,
0.35931187583389,0.388902576805948,0.448083978750065,0.484049840267495,
0.520015701784926,0.591947424819786,0.634833203943942,0.677718983068097,
0.763490541316409,0.884888589856318),.UNSPECIFIED.);
#152=B_SPLINE_SURFACE_WITH_KNOTS('',3,3,((#54391,#54392,#54393,#54394,#54395,
#54396,#54397,#54398,#54399,#54400,#54401,#54402,#54403,#54404,#54405,#54406,
#54407,#54408,#54409,#54410,#54411,#54412,#54413,#54414,#54415,#54416,#54417,
#54418,#54419,#54420,#54421,#54422,#54423,#54424,#54425),(#54426,#54427,
#54428,#54429,#54430,#54431,#54432,#54433,#54434,#54435,#54436,#54437,#54438,
#54439,#54440,#54441,#54442,#54443,#54444,#54445,#54446,#54447,#54448,#54449,
#54450,#54451,#54452,#54453,#54454,#54455,#54456,#54457,#54458,#54459,#54460),
(#54461,#54462,#54463,#54464,#54465,#54466,#54467,#54468,#54469,#54470,
#54471,#54472,#54473,#54474,#54475,#54476,#54477,#54478,#54479,#54480,#54481,
#54482,#54483,#54484,#54485,#54486,#54487,#54488,#54489,#54490,#54491,#54492,
#54493,#54494,#54495),(#54496,#54497,#54498,#54499,#54500,#54501,#54502,
#54503,#54504,#54505,#54506,#54507,#54508,#54509,#54510,#54511,#54512,#54513,
#54514,#54515,#54516,#54517,#54518,#54519,#54520,#54521,#54522,#54523,#54524,
#54525,#54526,#54527,#54528,#54529,#54530),(#54531,#54532,#54533,#54534,
#54535,#54536,#54537,#54538,#54539,#54540,#54541,#54542,#54543,#54544,#54545,
#54546,#54547,#54548,#54549,#54550,#54551,#54552,#54553,#54554,#54555,#54556,
#54557,#54558,#54559,#54560,#54561,#54562,#54563,#54564,#54565),(#54566,
#54567,#54568,#54569,#54570,#54571,#54572,#54573,#54574,#54575,#54576,#54577,
#54578,#54579,#54580,#54581,#54582,#54583,#54584,#54585,#54586,#54587,#54588,
#54589,#54590,#54591,#54592,#54593,#54594,#54595,#54596,#54597,#54598,#54599,
#54600)),.UNSPECIFIED.,.F.,.F.,.F.,(4,1,1,4),(4,2,1,1,1,2,1,1,1,1,1,1,2,
1,1,2,1,1,2,1,1,2,1,1,2,4),(0.0818357476916571,0.335421485070539,0.58900722244942,
0.969385828517743),(0.0162979902041912,0.0679082925174644,0.0780945363950841,
0.0882807802727037,0.108653268027943,0.149398243538422,0.154611429799316,
0.159824616060209,0.170250988581997,0.180677361103785,0.191103733625573,
0.211956478669149,0.232809223712724,0.281265199287278,0.305493187074555,
0.329721174861832,0.35931187583389,0.388902576805948,0.448083978750065,
0.484049840267495,0.520015701784926,0.591947424819786,0.634833203943942,
0.677718983068097,0.763490541316409,0.988990749040375),.UNSPECIFIED.);
#153=B_SPLINE_SURFACE_WITH_KNOTS('',3,3,((#54660,#54661,#54662,#54663,#54664,
#54665,#54666,#54667,#54668,#54669,#54670,#54671,#54672,#54673,#54674,#54675,
#54676,#54677,#54678,#54679,#54680,#54681,#54682,#54683,#54684,#54685,#54686,
#54687,#54688,#54689,#54690,#54691,#54692,#54693,#54694),(#54695,#54696,
#54697,#54698,#54699,#54700,#54701,#54702,#54703,#54704,#54705,#54706,#54707,
#54708,#54709,#54710,#54711,#54712,#54713,#54714,#54715,#54716,#54717,#54718,
#54719,#54720,#54721,#54722,#54723,#54724,#54725,#54726,#54727,#54728,#54729),
(#54730,#54731,#54732,#54733,#54734,#54735,#54736,#54737,#54738,#54739,
#54740,#54741,#54742,#54743,#54744,#54745,#54746,#54747,#54748,#54749,#54750,
#54751,#54752,#54753,#54754,#54755,#54756,#54757,#54758,#54759,#54760,#54761,
#54762,#54763,#54764),(#54765,#54766,#54767,#54768,#54769,#54770,#54771,
#54772,#54773,#54774,#54775,#54776,#54777,#54778,#54779,#54780,#54781,#54782,
#54783,#54784,#54785,#54786,#54787,#54788,#54789,#54790,#54791,#54792,#54793,
#54794,#54795,#54796,#54797,#54798,#54799),(#54800,#54801,#54802,#54803,
#54804,#54805,#54806,#54807,#54808,#54809,#54810,#54811,#54812,#54813,#54814,
#54815,#54816,#54817,#54818,#54819,#54820,#54821,#54822,#54823,#54824,#54825,
#54826,#54827,#54828,#54829,#54830,#54831,#54832,#54833,#54834)),
 .UNSPECIFIED.,.F.,.F.,.F.,(4,1,4),(4,2,1,1,1,2,1,1,1,1,1,1,1,2,1,2,1,1,
2,1,1,2,1,1,2,4),(0.0818907219452629,0.462246010974744,0.969386396347385),
(0.0162979902041915,0.0679082925174644,0.0780945363950841,0.0882807802727037,
0.108653268027943,0.149398243538422,0.154611429799316,0.159824616060209,
0.165037802321103,0.170250988581997,0.191103733625573,0.211956478669149,
0.222382851190937,0.232809223712724,0.281265199287278,0.329721174861832,
0.35931187583389,0.388902576805948,0.448083978750065,0.484049840267495,
0.520015701784926,0.591947424819786,0.634833203943942,0.677718983068097,
0.763490541316409,0.884888589856319),.UNSPECIFIED.);
#154=B_SPLINE_SURFACE_WITH_KNOTS('',3,3,((#55243,#55244,#55245,#55246,#55247,
#55248,#55249,#55250,#55251,#55252,#55253,#55254,#55255,#55256,#55257,#55258,
#55259,#55260,#55261,#55262,#55263,#55264,#55265,#55266,#55267,#55268,#55269,
#55270,#55271,#55272,#55273,#55274,#55275,#55276,#55277),(#55278,#55279,
#55280,#55281,#55282,#55283,#55284,#55285,#55286,#55287,#55288,#55289,#55290,
#55291,#55292,#55293,#55294,#55295,#55296,#55297,#55298,#55299,#55300,#55301,
#55302,#55303,#55304,#55305,#55306,#55307,#55308,#55309,#55310,#55311,#55312),
(#55313,#55314,#55315,#55316,#55317,#55318,#55319,#55320,#55321,#55322,
#55323,#55324,#55325,#55326,#55327,#55328,#55329,#55330,#55331,#55332,#55333,
#55334,#55335,#55336,#55337,#55338,#55339,#55340,#55341,#55342,#55343,#55344,
#55345,#55346,#55347),(#55348,#55349,#55350,#55351,#55352,#55353,#55354,
#55355,#55356,#55357,#55358,#55359,#55360,#55361,#55362,#55363,#55364,#55365,
#55366,#55367,#55368,#55369,#55370,#55371,#55372,#55373,#55374,#55375,#55376,
#55377,#55378,#55379,#55380,#55381,#55382),(#55383,#55384,#55385,#55386,
#55387,#55388,#55389,#55390,#55391,#55392,#55393,#55394,#55395,#55396,#55397,
#55398,#55399,#55400,#55401,#55402,#55403,#55404,#55405,#55406,#55407,#55408,
#55409,#55410,#55411,#55412,#55413,#55414,#55415,#55416,#55417)),
 .UNSPECIFIED.,.F.,.F.,.F.,(4,1,4),(4,2,1,1,1,2,1,1,1,1,1,1,1,2,1,2,1,1,
2,1,1,2,1,1,2,4),(0.081835747691657,0.462214353759979,0.969385828517743),
(0.0162979902041914,0.0679082925174644,0.0780945363950841,0.0882807802727037,
0.108653268027943,0.149398243538422,0.154611429799316,0.159824616060209,
0.165037802321103,0.170250988581997,0.191103733625573,0.211956478669149,
0.222382851190937,0.232809223712724,0.281265199287278,0.329721174861832,
0.35931187583389,0.388902576805948,0.448083978750065,0.484049840267495,
0.520015701784926,0.591947424819786,0.634833203943942,0.677718983068097,
0.763490541316409,0.988990749040375),.UNSPECIFIED.);
#155=B_SPLINE_SURFACE_WITH_KNOTS('',3,3,((#55477,#55478,#55479,#55480,#55481,
#55482,#55483,#55484,#55485,#55486,#55487,#55488,#55489,#55490,#55491,#55492,
#55493,#55494,#55495,#55496,#55497,#55498,#55499,#55500,#55501,#55502,#55503,
#55504,#55505,#55506,#55507,#55508,#55509,#55510,#55511),(#55512,#55513,
#55514,#55515,#55516,#55517,#55518,#55519,#55520,#55521,#55522,#55523,#55524,
#55525,#55526,#55527,#55528,#55529,#55530,#55531,#55532,#55533,#55534,#55535,
#55536,#55537,#55538,#55539,#55540,#55541,#55542,#55543,#55544,#55545,#55546),
(#55547,#55548,#55549,#55550,#55551,#55552,#55553,#55554,#55555,#55556,
#55557,#55558,#55559,#55560,#55561,#55562,#55563,#55564,#55565,#55566,#55567,
#55568,#55569,#55570,#55571,#55572,#55573,#55574,#55575,#55576,#55577,#55578,
#55579,#55580,#55581),(#55582,#55583,#55584,#55585,#55586,#55587,#55588,
#55589,#55590,#55591,#55592,#55593,#55594,#55595,#55596,#55597,#55598,#55599,
#55600,#55601,#55602,#55603,#55604,#55605,#55606,#55607,#55608,#55609,#55610,
#55611,#55612,#55613,#55614,#55615,#55616),(#55617,#55618,#55619,#55620,
#55621,#55622,#55623,#55624,#55625,#55626,#55627,#55628,#55629,#55630,#55631,
#55632,#55633,#55634,#55635,#55636,#55637,#55638,#55639,#55640,#55641,#55642,
#55643,#55644,#55645,#55646,#55647,#55648,#55649,#55650,#55651)),
 .UNSPECIFIED.,.F.,.F.,.F.,(4,1,4),(4,2,1,1,1,2,1,1,1,1,1,1,1,2,1,2,1,1,
2,1,1,2,1,1,2,4),(0.0818907219452629,0.462246010974744,0.969386396347385),
(0.0162979902041911,0.0679082925174644,0.0780945363950841,0.0882807802727037,
0.108653268027943,0.149398243538422,0.154611429799316,0.159824616060209,
0.165037802321103,0.170250988581997,0.191103733625573,0.211956478669149,
0.222382851190937,0.232809223712724,0.281265199287278,0.329721174861832,
0.35931187583389,0.388902576805948,0.448083978750065,0.484049840267495,
0.520015701784926,0.591947424819786,0.634833203943942,0.677718983068097,
0.763490541316409,0.884888589856318),.UNSPECIFIED.);
#156=B_SPLINE_SURFACE_WITH_KNOTS('',3,3,((#56065,#56066,#56067,#56068,#56069,
#56070,#56071,#56072,#56073,#56074,#56075,#56076,#56077,#56078,#56079,#56080,
#56081,#56082,#56083,#56084,#56085,#56086,#56087,#56088,#56089,#56090,#56091,
#56092,#56093,#56094,#56095,#56096,#56097,#56098,#56099,#56100),(#56101,
#56102,#56103,#56104,#56105,#56106,#56107,#56108,#56109,#56110,#56111,#56112,
#56113,#56114,#56115,#56116,#56117,#56118,#56119,#56120,#56121,#56122,#56123,
#56124,#56125,#56126,#56127,#56128,#56129,#56130,#56131,#56132,#56133,#56134,
#56135,#56136),(#56137,#56138,#56139,#56140,#56141,#56142,#56143,#56144,
#56145,#56146,#56147,#56148,#56149,#56150,#56151,#56152,#56153,#56154,#56155,
#56156,#56157,#56158,#56159,#56160,#56161,#56162,#56163,#56164,#56165,#56166,
#56167,#56168,#56169,#56170,#56171,#56172),(#56173,#56174,#56175,#56176,
#56177,#56178,#56179,#56180,#56181,#56182,#56183,#56184,#56185,#56186,#56187,
#56188,#56189,#56190,#56191,#56192,#56193,#56194,#56195,#56196,#56197,#56198,
#56199,#56200,#56201,#56202,#56203,#56204,#56205,#56206,#56207,#56208),
(#56209,#56210,#56211,#56212,#56213,#56214,#56215,#56216,#56217,#56218,
#56219,#56220,#56221,#56222,#56223,#56224,#56225,#56226,#56227,#56228,#56229,
#56230,#56231,#56232,#56233,#56234,#56235,#56236,#56237,#56238,#56239,#56240,
#56241,#56242,#56243,#56244)),.UNSPECIFIED.,.F.,.F.,.F.,(4,1,4),(4,2,1,
1,2,1,1,1,1,1,1,1,2,1,1,2,1,1,2,1,1,2,1,1,1,2,4),(0.0818357476933141,0.462214353760926,
0.969385828517743),(0.0162979902041911,0.0679082925174644,0.0882807802727037,
0.108653268027943,0.149398243538422,0.154611429799316,0.159824616060209,
0.165037802321103,0.170250988581997,0.191103733625573,0.211956478669149,
0.222382851190937,0.232809223712724,0.281265199287278,0.305493187074555,
0.329721174861832,0.35931187583389,0.388902576805948,0.448083978750065,
0.484049840267495,0.520015701784926,0.591947424819786,0.613390314381864,
0.634833203943942,0.677718983068097,0.763490541316409,0.988990749040375),
 .UNSPECIFIED.);
#157=B_SPLINE_SURFACE_WITH_KNOTS('',3,3,((#56626,#56627,#56628,#56629,#56630,
#56631,#56632,#56633,#56634,#56635,#56636,#56637,#56638,#56639,#56640,#56641,
#56642,#56643,#56644,#56645,#56646,#56647,#56648,#56649,#56650,#56651,#56652,
#56653,#56654,#56655,#56656,#56657,#56658,#56659,#56660),(#56661,#56662,
#56663,#56664,#56665,#56666,#56667,#56668,#56669,#56670,#56671,#56672,#56673,
#56674,#56675,#56676,#56677,#56678,#56679,#56680,#56681,#56682,#56683,#56684,
#56685,#56686,#56687,#56688,#56689,#56690,#56691,#56692,#56693,#56694,#56695),
(#56696,#56697,#56698,#56699,#56700,#56701,#56702,#56703,#56704,#56705,
#56706,#56707,#56708,#56709,#56710,#56711,#56712,#56713,#56714,#56715,#56716,
#56717,#56718,#56719,#56720,#56721,#56722,#56723,#56724,#56725,#56726,#56727,
#56728,#56729,#56730),(#56731,#56732,#56733,#56734,#56735,#56736,#56737,
#56738,#56739,#56740,#56741,#56742,#56743,#56744,#56745,#56746,#56747,#56748,
#56749,#56750,#56751,#56752,#56753,#56754,#56755,#56756,#56757,#56758,#56759,
#56760,#56761,#56762,#56763,#56764,#56765),(#56766,#56767,#56768,#56769,
#56770,#56771,#56772,#56773,#56774,#56775,#56776,#56777,#56778,#56779,#56780,
#56781,#56782,#56783,#56784,#56785,#56786,#56787,#56788,#56789,#56790,#56791,
#56792,#56793,#56794,#56795,#56796,#56797,#56798,#56799,#56800)),
 .UNSPECIFIED.,.F.,.F.,.F.,(4,1,4),(4,2,1,1,1,2,1,1,1,1,1,1,1,2,1,2,1,1,
2,1,1,2,1,1,2,4),(0.081890721945263,0.462246010974744,0.969386396347385),
(0.0162979902041911,0.0679082925174644,0.0780945363950841,0.0882807802727037,
0.108653268027943,0.149398243538422,0.154611429799316,0.159824616060209,
0.165037802321103,0.170250988581997,0.191103733625573,0.211956478669149,
0.222382851190937,0.232809223712724,0.281265199287278,0.329721174861832,
0.35931187583389,0.388902576805948,0.448083978750065,0.484049840267495,
0.520015701784926,0.591947424819786,0.634833203943942,0.677718983068097,
0.763490541316409,0.884888589856318),.UNSPECIFIED.);
#158=B_SPLINE_SURFACE_WITH_KNOTS('',3,3,((#57155,#57156,#57157,#57158,#57159,
#57160,#57161,#57162,#57163,#57164,#57165,#57166,#57167,#57168,#57169,#57170,
#57171,#57172,#57173,#57174,#57175,#57176,#57177,#57178,#57179,#57180,#57181,
#57182,#57183,#57184,#57185,#57186,#57187,#57188,#57189),(#57190,#57191,
#57192,#57193,#57194,#57195,#57196,#57197,#57198,#57199,#57200,#57201,#57202,
#57203,#57204,#57205,#57206,#57207,#57208,#57209,#57210,#57211,#57212,#57213,
#57214,#57215,#57216,#57217,#57218,#57219,#57220,#57221,#57222,#57223,#57224),
(#57225,#57226,#57227,#57228,#57229,#57230,#57231,#57232,#57233,#57234,
#57235,#57236,#57237,#57238,#57239,#57240,#57241,#57242,#57243,#57244,#57245,
#57246,#57247,#57248,#57249,#57250,#57251,#57252,#57253,#57254,#57255,#57256,
#57257,#57258,#57259),(#57260,#57261,#57262,#57263,#57264,#57265,#57266,
#57267,#57268,#57269,#57270,#57271,#57272,#57273,#57274,#57275,#57276,#57277,
#57278,#57279,#57280,#57281,#57282,#57283,#57284,#57285,#57286,#57287,#57288,
#57289,#57290,#57291,#57292,#57293,#57294),(#57295,#57296,#57297,#57298,
#57299,#57300,#57301,#57302,#57303,#57304,#57305,#57306,#57307,#57308,#57309,
#57310,#57311,#57312,#57313,#57314,#57315,#57316,#57317,#57318,#57319,#57320,
#57321,#57322,#57323,#57324,#57325,#57326,#57327,#57328,#57329),(#57330,
#57331,#57332,#57333,#57334,#57335,#57336,#57337,#57338,#57339,#57340,#57341,
#57342,#57343,#57344,#57345,#57346,#57347,#57348,#57349,#57350,#57351,#57352,
#57353,#57354,#57355,#57356,#57357,#57358,#57359,#57360,#57361,#57362,#57363,
#57364)),.UNSPECIFIED.,.F.,.F.,.F.,(4,1,1,4),(4,2,1,1,1,2,1,1,1,1,1,1,2,
1,1,2,1,1,2,1,1,2,1,1,2,4),(0.0818357476916571,0.335421485070539,0.58900722244942,
0.969385828517743),(0.0162979902041911,0.0679082925174644,0.0780945363950841,
0.0882807802727037,0.108653268027943,0.149398243538422,0.154611429799316,
0.159824616060209,0.170250988581997,0.180677361103785,0.191103733625573,
0.211956478669149,0.232809223712724,0.281265199287278,0.305493187074555,
0.329721174861832,0.35931187583389,0.388902576805948,0.448083978750065,
0.484049840267495,0.520015701784926,0.591947424819786,0.634833203943942,
0.677718983068097,0.763490541316409,0.988990749040375),.UNSPECIFIED.);
#241=FACE_BOUND('',#2922,.T.);
#242=FACE_BOUND('',#2925,.T.);
#608=PLANE('',#19300);
#609=PLANE('',#19304);
#610=PLANE('',#19306);
#611=PLANE('',#19310);
#612=PLANE('',#19314);
#613=PLANE('',#19318);
#614=PLANE('',#19322);
#615=PLANE('',#19326);
#616=PLANE('',#19330);
#617=PLANE('',#19333);
#618=PLANE('',#19337);
#619=PLANE('',#19341);
#620=PLANE('',#19345);
#621=PLANE('',#19349);
#622=PLANE('',#19353);
#623=PLANE('',#19359);
#922=CONICAL_SURFACE('',#19234,38.7702137424955,0.582952270254907);
#923=CONICAL_SURFACE('',#19267,38.7702137424955,0.582952270254903);
#924=CONICAL_SURFACE('',#19269,38.7702137424955,0.582952270254907);
#925=CONICAL_SURFACE('',#19271,38.7702137424955,0.582952270254917);
#926=CONICAL_SURFACE('',#19273,38.7702137424955,0.582952270254906);
#927=CONICAL_SURFACE('',#19275,38.7702137424955,0.582952270254903);
#928=CONICAL_SURFACE('',#19277,38.7702137424955,0.582952270254906);
#929=CONICAL_SURFACE('',#19279,38.7702137424955,0.582952270254907);
#930=CONICAL_SURFACE('',#19281,38.7702137424955,0.582952270254906);
#931=CONICAL_SURFACE('',#19283,38.7702137424955,0.582952270254906);
#932=CONICAL_SURFACE('',#19285,38.7702137424955,0.582952270254902);
#933=CONICAL_SURFACE('',#19287,38.7702137424955,0.582952270254911);
#934=CONICAL_SURFACE('',#19289,38.7702137424955,0.582952270254907);
#935=CONICAL_SURFACE('',#19291,38.7702137424955,0.582952270254902);
#936=CONICAL_SURFACE('',#19293,3.675,0.785398163397447);
#937=CONICAL_SURFACE('',#19302,3.675,0.785398163397451);
#938=CONICAL_SURFACE('',#19308,38.3,1.16590454050981);
#939=CONICAL_SURFACE('',#19312,38.3,1.16590454050981);
#940=CONICAL_SURFACE('',#19316,38.3,1.16590454050981);
#941=CONICAL_SURFACE('',#19320,38.3,1.16590454050981);
#942=CONICAL_SURFACE('',#19324,38.3,1.16590454050981);
#943=CONICAL_SURFACE('',#19328,38.3,1.16590454050981);
#944=CONICAL_SURFACE('',#19332,38.3,1.16590454050981);
#945=CONICAL_SURFACE('',#19335,38.3,1.16590454050981);
#946=CONICAL_SURFACE('',#19339,38.3,1.16590454050981);
#947=CONICAL_SURFACE('',#19343,38.3,1.16590454050981);
#948=CONICAL_SURFACE('',#19347,38.3,1.16590454050981);
#949=CONICAL_SURFACE('',#19351,38.3,1.16590454050981);
#950=CONICAL_SURFACE('',#19355,38.3,1.16590454050981);
#951=CONICAL_SURFACE('',#19361,38.75,0.785398163397447);
#952=CONICAL_SURFACE('',#19362,38.3,1.16590454050981);
#953=CONICAL_SURFACE('',#19363,8.95,1.19028994968254);
#954=CONICAL_SURFACE('',#19367,8.4,0.785398163397447);
#1054=(
BOUNDED_CURVE()
B_SPLINE_CURVE(5,(#47338,#47339,#47340,#47341,#47342,#47343,#47344,#47345,
#47346,#47347,#47348,#47349,#47350,#47351,#47352,#47353,#47354),
 .UNSPECIFIED.,.F.,.F.)
B_SPLINE_CURVE_WITH_KNOTS((6,1,1,1,1,1,1,1,1,1,1,1,6),(0.422875935222759,
0.44,0.48,0.52,0.56,0.6,0.64,0.68,0.72,0.76,0.8,0.84,0.867889296212967),
 .UNSPECIFIED.)
CURVE()
GEOMETRIC_REPRESENTATION_ITEM()
RATIONAL_B_SPLINE_CURVE((1.,1.,1.,1.,1.,1.,1.,1.,1.,1.,1.,1.,1.,1.,1.,1.,
1.))
REPRESENTATION_ITEM('')
);
#1055=(
BOUNDED_CURVE()
B_SPLINE_CURVE(5,(#56525,#56526,#56527,#56528,#56529,#56530,#56531,#56532),
 .UNSPECIFIED.,.F.,.F.)
B_SPLINE_CURVE_WITH_KNOTS((6,1,1,6),(0.904281576377558,0.92,0.96,1.),
 .UNSPECIFIED.)
CURVE()
GEOMETRIC_REPRESENTATION_ITEM()
RATIONAL_B_SPLINE_CURVE((1.,1.,1.,1.,1.,1.,1.,1.))
REPRESENTATION_ITEM('')
);
#1082=(
BOUNDED_SURFACE()
B_SPLINE_SURFACE(5,2,((#47066,#47067,#47068,#47069,#47070,#47071,#47072,
#47073,#47074),(#47075,#47076,#47077,#47078,#47079,#47080,#47081,#47082,
#47083),(#47084,#47085,#47086,#47087,#47088,#47089,#47090,#47091,#47092),
(#47093,#47094,#47095,#47096,#47097,#47098,#47099,#47100,#47101),(#47102,
#47103,#47104,#47105,#47106,#47107,#47108,#47109,#47110),(#47111,#47112,
#47113,#47114,#47115,#47116,#47117,#47118,#47119),(#47120,#47121,#47122,
#47123,#47124,#47125,#47126,#47127,#47128),(#47129,#47130,#47131,#47132,
#47133,#47134,#47135,#47136,#47137),(#47138,#47139,#47140,#47141,#47142,
#47143,#47144,#47145,#47146),(#47147,#47148,#47149,#47150,#47151,#47152,
#47153,#47154,#47155),(#47156,#47157,#47158,#47159,#47160,#47161,#47162,
#47163,#47164),(#47165,#47166,#47167,#47168,#47169,#47170,#47171,#47172,
#47173),(#47174,#47175,#47176,#47177,#47178,#47179,#47180,#47181,#47182),
(#47183,#47184,#47185,#47186,#47187,#47188,#47189,#47190,#47191),(#47192,
#47193,#47194,#47195,#47196,#47197,#47198,#47199,#47200),(#47201,#47202,
#47203,#47204,#47205,#47206,#47207,#47208,#47209),(#47210,#47211,#47212,
#47213,#47214,#47215,#47216,#47217,#47218),(#47219,#47220,#47221,#47222,
#47223,#47224,#47225,#47226,#47227),(#47228,#47229,#47230,#47231,#47232,
#47233,#47234,#47235,#47236),(#47237,#47238,#47239,#47240,#47241,#47242,
#47243,#47244,#47245),(#47246,#47247,#47248,#47249,#47250,#47251,#47252,
#47253,#47254),(#47255,#47256,#47257,#47258,#47259,#47260,#47261,#47262,
#47263),(#47264,#47265,#47266,#47267,#47268,#47269,#47270,#47271,#47272),
(#47273,#47274,#47275,#47276,#47277,#47278,#47279,#47280,#47281),(#47282,
#47283,#47284,#47285,#47286,#47287,#47288,#47289,#47290),(#47291,#47292,
#47293,#47294,#47295,#47296,#47297,#47298,#47299),(#47300,#47301,#47302,
#47303,#47304,#47305,#47306,#47307,#47308),(#47309,#47310,#47311,#47312,
#47313,#47314,#47315,#47316,#47317),(#47318,#47319,#47320,#47321,#47322,
#47323,#47324,#47325,#47326),(#47327,#47328,#47329,#47330,#47331,#47332,
#47333,#47334,#47335)),.UNSPECIFIED.,.F.,.T.,.F.)
B_SPLINE_SURFACE_WITH_KNOTS((6,1,1,1,1,1,1,1,1,1,1,1,1,1,1,1,1,1,1,1,1,
1,1,1,1,6),(3,2,2,2,3),(-1.,-0.96,-0.92,-0.88,-0.84,-0.8,-0.76,-0.72,-0.68,
-0.64,-0.6,-0.56,-0.52,-0.48,-0.44,-0.4,-0.36,-0.32,-0.28,-0.24,-0.2,-0.16,
-0.12,-0.08,-0.04,0.),(0.,1.5707963267949,3.14159265358979,4.71238898038469,
6.28318530717959),.UNSPECIFIED.)
GEOMETRIC_REPRESENTATION_ITEM()
RATIONAL_B_SPLINE_SURFACE(((1.,0.707106781186548,1.,0.707106781186548,1.,
0.707106781186548,1.,0.707106781186548,1.),(1.,0.707106781186548,1.,0.707106781186548,
1.,0.707106781186548,1.,0.707106781186548,1.),(1.,0.707106781186548,1.,
0.707106781186548,1.,0.707106781186548,1.,0.707106781186548,1.),(1.,0.707106781186548,
1.,0.707106781186548,1.,0.707106781186548,1.,0.707106781186548,1.),(1.,
0.707106781186548,1.,0.707106781186548,1.,0.707106781186548,1.,0.707106781186548,
1.),(1.,0.707106781186548,1.,0.707106781186548,1.,0.707106781186548,1.,
0.707106781186548,1.),(1.,0.707106781186548,1.,0.707106781186548,1.,0.707106781186548,
1.,0.707106781186548,1.),(1.,0.707106781186548,1.,0.707106781186548,1.,
0.707106781186548,1.,0.707106781186548,1.),(1.,0.707106781186548,1.,0.707106781186548,
1.,0.707106781186548,1.,0.707106781186548,1.),(1.,0.707106781186548,1.,
0.707106781186548,1.,0.707106781186548,1.,0.707106781186548,1.),(1.,0.707106781186548,
1.,0.707106781186548,1.,0.707106781186548,1.,0.707106781186548,1.),(1.,
0.707106781186548,1.,0.707106781186548,1.,0.707106781186548,1.,0.707106781186548,
1.),(1.,0.707106781186548,1.,0.707106781186548,1.,0.707106781186548,1.,
0.707106781186548,1.),(1.,0.707106781186548,1.,0.707106781186548,1.,0.707106781186548,
1.,0.707106781186548,1.),(1.,0.707106781186548,1.,0.707106781186548,1.,
0.707106781186548,1.,0.707106781186548,1.),(1.,0.707106781186548,1.,0.707106781186548,
1.,0.707106781186548,1.,0.707106781186548,1.),(1.,0.707106781186548,1.,
0.707106781186548,1.,0.707106781186548,1.,0.707106781186548,1.),(1.,0.707106781186548,
1.,0.707106781186548,1.,0.707106781186548,1.,0.707106781186548,1.),(1.,
0.707106781186548,1.,0.707106781186548,1.,0.707106781186548,1.,0.707106781186548,
1.),(1.,0.707106781186548,1.,0.707106781186548,1.,0.707106781186548,1.,
0.707106781186548,1.),(1.,0.707106781186548,1.,0.707106781186548,1.,0.707106781186548,
1.,0.707106781186548,1.),(1.,0.707106781186548,1.,0.707106781186548,1.,
0.707106781186548,1.,0.707106781186548,1.),(1.,0.707106781186548,1.,0.707106781186548,
1.,0.707106781186548,1.,0.707106781186548,1.),(1.,0.707106781186548,1.,
0.707106781186548,1.,0.707106781186548,1.,0.707106781186548,1.),(1.,0.707106781186548,
1.,0.707106781186548,1.,0.707106781186548,1.,0.707106781186548,1.),(1.,
0.707106781186548,1.,0.707106781186548,1.,0.707106781186548,1.,0.707106781186548,
1.),(1.,0.707106781186548,1.,0.707106781186548,1.,0.707106781186548,1.,
0.707106781186548,1.),(1.,0.707106781186548,1.,0.707106781186548,1.,0.707106781186548,
1.,0.707106781186548,1.),(1.,0.707106781186548,1.,0.707106781186548,1.,
0.707106781186548,1.,0.707106781186548,1.),(1.,0.707106781186548,1.,0.707106781186548,
1.,0.707106781186548,1.,0.707106781186548,1.)))
REPRESENTATION_ITEM('')
SURFACE()
);
#1083=(
BOUNDED_SURFACE()
B_SPLINE_SURFACE(5,2,((#48257,#48258,#48259,#48260,#48261,#48262,#48263,
#48264,#48265),(#48266,#48267,#48268,#48269,#48270,#48271,#48272,#48273,
#48274),(#48275,#48276,#48277,#48278,#48279,#48280,#48281,#48282,#48283),
(#48284,#48285,#48286,#48287,#48288,#48289,#48290,#48291,#48292),(#48293,
#48294,#48295,#48296,#48297,#48298,#48299,#48300,#48301),(#48302,#48303,
#48304,#48305,#48306,#48307,#48308,#48309,#48310),(#48311,#48312,#48313,
#48314,#48315,#48316,#48317,#48318,#48319),(#48320,#48321,#48322,#48323,
#48324,#48325,#48326,#48327,#48328),(#48329,#48330,#48331,#48332,#48333,
#48334,#48335,#48336,#48337),(#48338,#48339,#48340,#48341,#48342,#48343,
#48344,#48345,#48346),(#48347,#48348,#48349,#48350,#48351,#48352,#48353,
#48354,#48355),(#48356,#48357,#48358,#48359,#48360,#48361,#48362,#48363,
#48364),(#48365,#48366,#48367,#48368,#48369,#48370,#48371,#48372,#48373),
(#48374,#48375,#48376,#48377,#48378,#48379,#48380,#48381,#48382),(#48383,
#48384,#48385,#48386,#48387,#48388,#48389,#48390,#48391)),.UNSPECIFIED.,
 .F.,.T.,.F.)
B_SPLINE_SURFACE_WITH_KNOTS((6,1,1,1,1,1,1,1,1,1,6),(3,2,2,2,3),(-1.,-0.9,
-0.8,-0.7,-0.6,-0.5,-0.4,-0.3,-0.2,-0.1,0.),(0.,1.5707963267949,3.14159265358979,
4.71238898038469,6.28318530717959),.UNSPECIFIED.)
GEOMETRIC_REPRESENTATION_ITEM()
RATIONAL_B_SPLINE_SURFACE(((1.,0.707106781186548,1.,0.707106781186548,1.,
0.707106781186548,1.,0.707106781186548,1.),(1.,0.707106781186548,1.,0.707106781186548,
1.,0.707106781186548,1.,0.707106781186548,1.),(1.,0.707106781186548,1.,
0.707106781186548,1.,0.707106781186548,1.,0.707106781186548,1.),(1.,0.707106781186548,
1.,0.707106781186548,1.,0.707106781186548,1.,0.707106781186548,1.),(1.,
0.707106781186548,1.,0.707106781186548,1.,0.707106781186548,1.,0.707106781186548,
1.),(1.,0.707106781186548,1.,0.707106781186548,1.,0.707106781186548,1.,
0.707106781186548,1.),(1.,0.707106781186548,1.,0.707106781186548,1.,0.707106781186548,
1.,0.707106781186548,1.),(1.,0.707106781186548,1.,0.707106781186548,1.,
0.707106781186548,1.,0.707106781186548,1.),(1.,0.707106781186548,1.,0.707106781186548,
1.,0.707106781186548,1.,0.707106781186548,1.),(1.,0.707106781186548,1.,
0.707106781186548,1.,0.707106781186548,1.,0.707106781186548,1.),(1.,0.707106781186548,
1.,0.707106781186548,1.,0.707106781186548,1.,0.707106781186548,1.),(1.,
0.707106781186548,1.,0.707106781186548,1.,0.707106781186548,1.,0.707106781186548,
1.),(1.,0.707106781186548,1.,0.707106781186548,1.,0.707106781186548,1.,
0.707106781186548,1.),(1.,0.707106781186548,1.,0.707106781186548,1.,0.707106781186548,
1.,0.707106781186548,1.),(1.,0.707106781186548,1.,0.707106781186548,1.,
0.707106781186548,1.,0.707106781186548,1.)))
REPRESENTATION_ITEM('')
SURFACE()
);
#1084=(
BOUNDED_SURFACE()
B_SPLINE_SURFACE(5,2,((#48727,#48728,#48729,#48730,#48731,#48732,#48733,
#48734,#48735),(#48736,#48737,#48738,#48739,#48740,#48741,#48742,#48743,
#48744),(#48745,#48746,#48747,#48748,#48749,#48750,#48751,#48752,#48753),
(#48754,#48755,#48756,#48757,#48758,#48759,#48760,#48761,#48762),(#48763,
#48764,#48765,#48766,#48767,#48768,#48769,#48770,#48771),(#48772,#48773,
#48774,#48775,#48776,#48777,#48778,#48779,#48780),(#48781,#48782,#48783,
#48784,#48785,#48786,#48787,#48788,#48789),(#48790,#48791,#48792,#48793,
#48794,#48795,#48796,#48797,#48798),(#48799,#48800,#48801,#48802,#48803,
#48804,#48805,#48806,#48807),(#48808,#48809,#48810,#48811,#48812,#48813,
#48814,#48815,#48816),(#48817,#48818,#48819,#48820,#48821,#48822,#48823,
#48824,#48825),(#48826,#48827,#48828,#48829,#48830,#48831,#48832,#48833,
#48834),(#48835,#48836,#48837,#48838,#48839,#48840,#48841,#48842,#48843),
(#48844,#48845,#48846,#48847,#48848,#48849,#48850,#48851,#48852),(#48853,
#48854,#48855,#48856,#48857,#48858,#48859,#48860,#48861)),.UNSPECIFIED.,
 .F.,.T.,.F.)
B_SPLINE_SURFACE_WITH_KNOTS((6,1,1,1,1,1,1,1,1,1,6),(3,2,2,2,3),(-1.,-0.9,
-0.8,-0.7,-0.6,-0.5,-0.4,-0.3,-0.2,-0.1,0.),(0.,1.5707963267949,3.14159265358979,
4.71238898038469,6.28318530717959),.UNSPECIFIED.)
GEOMETRIC_REPRESENTATION_ITEM()
RATIONAL_B_SPLINE_SURFACE(((1.,0.707106781186548,1.,0.707106781186548,1.,
0.707106781186548,1.,0.707106781186548,1.),(1.,0.707106781186548,1.,0.707106781186548,
1.,0.707106781186548,1.,0.707106781186548,1.),(1.,0.707106781186548,1.,
0.707106781186548,1.,0.707106781186548,1.,0.707106781186548,1.),(1.,0.707106781186548,
1.,0.707106781186548,1.,0.707106781186548,1.,0.707106781186548,1.),(1.,
0.707106781186548,1.,0.707106781186548,1.,0.707106781186548,1.,0.707106781186548,
1.),(1.,0.707106781186548,1.,0.707106781186548,1.,0.707106781186548,1.,
0.707106781186548,1.),(1.,0.707106781186548,1.,0.707106781186548,1.,0.707106781186548,
1.,0.707106781186548,1.),(1.,0.707106781186548,1.,0.707106781186548,1.,
0.707106781186548,1.,0.707106781186548,1.),(1.,0.707106781186548,1.,0.707106781186548,
1.,0.707106781186548,1.,0.707106781186548,1.),(1.,0.707106781186548,1.,
0.707106781186548,1.,0.707106781186548,1.,0.707106781186548,1.),(1.,0.707106781186548,
1.,0.707106781186548,1.,0.707106781186548,1.,0.707106781186548,1.),(1.,
0.707106781186548,1.,0.707106781186548,1.,0.707106781186548,1.,0.707106781186548,
1.),(1.,0.707106781186548,1.,0.707106781186548,1.,0.707106781186548,1.,
0.707106781186548,1.),(1.,0.707106781186548,1.,0.707106781186548,1.,0.707106781186548,
1.,0.707106781186548,1.),(1.,0.707106781186548,1.,0.707106781186548,1.,
0.707106781186548,1.,0.707106781186548,1.)))
REPRESENTATION_ITEM('')
SURFACE()
);
#1085=(
BOUNDED_SURFACE()
B_SPLINE_SURFACE(5,2,((#49197,#49198,#49199,#49200,#49201,#49202,#49203,
#49204,#49205),(#49206,#49207,#49208,#49209,#49210,#49211,#49212,#49213,
#49214),(#49215,#49216,#49217,#49218,#49219,#49220,#49221,#49222,#49223),
(#49224,#49225,#49226,#49227,#49228,#49229,#49230,#49231,#49232),(#49233,
#49234,#49235,#49236,#49237,#49238,#49239,#49240,#49241),(#49242,#49243,
#49244,#49245,#49246,#49247,#49248,#49249,#49250),(#49251,#49252,#49253,
#49254,#49255,#49256,#49257,#49258,#49259),(#49260,#49261,#49262,#49263,
#49264,#49265,#49266,#49267,#49268),(#49269,#49270,#49271,#49272,#49273,
#49274,#49275,#49276,#49277),(#49278,#49279,#49280,#49281,#49282,#49283,
#49284,#49285,#49286),(#49287,#49288,#49289,#49290,#49291,#49292,#49293,
#49294,#49295),(#49296,#49297,#49298,#49299,#49300,#49301,#49302,#49303,
#49304),(#49305,#49306,#49307,#49308,#49309,#49310,#49311,#49312,#49313),
(#49314,#49315,#49316,#49317,#49318,#49319,#49320,#49321,#49322),(#49323,
#49324,#49325,#49326,#49327,#49328,#49329,#49330,#49331)),.UNSPECIFIED.,
 .F.,.T.,.F.)
B_SPLINE_SURFACE_WITH_KNOTS((6,1,1,1,1,1,1,1,1,1,6),(3,2,2,2,3),(-1.,-0.9,
-0.8,-0.7,-0.6,-0.5,-0.4,-0.3,-0.2,-0.1,0.),(0.,1.5707963267949,3.14159265358979,
4.71238898038469,6.28318530717959),.UNSPECIFIED.)
GEOMETRIC_REPRESENTATION_ITEM()
RATIONAL_B_SPLINE_SURFACE(((1.,0.707106781186548,1.,0.707106781186548,1.,
0.707106781186548,1.,0.707106781186548,1.),(1.,0.707106781186548,1.,0.707106781186548,
1.,0.707106781186548,1.,0.707106781186548,1.),(1.,0.707106781186548,1.,
0.707106781186548,1.,0.707106781186548,1.,0.707106781186548,1.),(1.,0.707106781186548,
1.,0.707106781186548,1.,0.707106781186548,1.,0.707106781186548,1.),(1.,
0.707106781186548,1.,0.707106781186548,1.,0.707106781186548,1.,0.707106781186548,
1.),(1.,0.707106781186548,1.,0.707106781186548,1.,0.707106781186548,1.,
0.707106781186548,1.),(1.,0.707106781186548,1.,0.707106781186548,1.,0.707106781186548,
1.,0.707106781186548,1.),(1.,0.707106781186548,1.,0.707106781186548,1.,
0.707106781186548,1.,0.707106781186548,1.),(1.,0.707106781186548,1.,0.707106781186548,
1.,0.707106781186548,1.,0.707106781186548,1.),(1.,0.707106781186548,1.,
0.707106781186548,1.,0.707106781186548,1.,0.707106781186548,1.),(1.,0.707106781186548,
1.,0.707106781186548,1.,0.707106781186548,1.,0.707106781186548,1.),(1.,
0.707106781186548,1.,0.707106781186548,1.,0.707106781186548,1.,0.707106781186548,
1.),(1.,0.707106781186548,1.,0.707106781186548,1.,0.707106781186548,1.,
0.707106781186548,1.),(1.,0.707106781186548,1.,0.707106781186548,1.,0.707106781186548,
1.,0.707106781186548,1.),(1.,0.707106781186548,1.,0.707106781186548,1.,
0.707106781186548,1.,0.707106781186548,1.)))
REPRESENTATION_ITEM('')
SURFACE()
);
#1086=(
BOUNDED_SURFACE()
B_SPLINE_SURFACE(5,2,((#49669,#49670,#49671,#49672,#49673,#49674,#49675,
#49676,#49677),(#49678,#49679,#49680,#49681,#49682,#49683,#49684,#49685,
#49686),(#49687,#49688,#49689,#49690,#49691,#49692,#49693,#49694,#49695),
(#49696,#49697,#49698,#49699,#49700,#49701,#49702,#49703,#49704),(#49705,
#49706,#49707,#49708,#49709,#49710,#49711,#49712,#49713),(#49714,#49715,
#49716,#49717,#49718,#49719,#49720,#49721,#49722),(#49723,#49724,#49725,
#49726,#49727,#49728,#49729,#49730,#49731),(#49732,#49733,#49734,#49735,
#49736,#49737,#49738,#49739,#49740),(#49741,#49742,#49743,#49744,#49745,
#49746,#49747,#49748,#49749),(#49750,#49751,#49752,#49753,#49754,#49755,
#49756,#49757,#49758),(#49759,#49760,#49761,#49762,#49763,#49764,#49765,
#49766,#49767),(#49768,#49769,#49770,#49771,#49772,#49773,#49774,#49775,
#49776),(#49777,#49778,#49779,#49780,#49781,#49782,#49783,#49784,#49785),
(#49786,#49787,#49788,#49789,#49790,#49791,#49792,#49793,#49794),(#49795,
#49796,#49797,#49798,#49799,#49800,#49801,#49802,#49803)),.UNSPECIFIED.,
 .F.,.T.,.F.)
B_SPLINE_SURFACE_WITH_KNOTS((6,1,1,1,1,1,1,1,1,1,6),(3,2,2,2,3),(-1.,-0.9,
-0.8,-0.7,-0.6,-0.5,-0.4,-0.3,-0.2,-0.1,0.),(0.,1.5707963267949,3.14159265358979,
4.71238898038469,6.28318530717959),.UNSPECIFIED.)
GEOMETRIC_REPRESENTATION_ITEM()
RATIONAL_B_SPLINE_SURFACE(((1.,0.707106781186548,1.,0.707106781186548,1.,
0.707106781186548,1.,0.707106781186548,1.),(1.,0.707106781186548,1.,0.707106781186548,
1.,0.707106781186548,1.,0.707106781186548,1.),(1.,0.707106781186548,1.,
0.707106781186548,1.,0.707106781186548,1.,0.707106781186548,1.),(1.,0.707106781186548,
1.,0.707106781186548,1.,0.707106781186548,1.,0.707106781186548,1.),(1.,
0.707106781186548,1.,0.707106781186548,1.,0.707106781186548,1.,0.707106781186548,
1.),(1.,0.707106781186548,1.,0.707106781186548,1.,0.707106781186548,1.,
0.707106781186548,1.),(1.,0.707106781186548,1.,0.707106781186548,1.,0.707106781186548,
1.,0.707106781186548,1.),(1.,0.707106781186548,1.,0.707106781186548,1.,
0.707106781186548,1.,0.707106781186548,1.),(1.,0.707106781186548,1.,0.707106781186548,
1.,0.707106781186548,1.,0.707106781186548,1.),(1.,0.707106781186548,1.,
0.707106781186548,1.,0.707106781186548,1.,0.707106781186548,1.),(1.,0.707106781186548,
1.,0.707106781186548,1.,0.707106781186548,1.,0.707106781186548,1.),(1.,
0.707106781186548,1.,0.707106781186548,1.,0.707106781186548,1.,0.707106781186548,
1.),(1.,0.707106781186548,1.,0.707106781186548,1.,0.707106781186548,1.,
0.707106781186548,1.),(1.,0.707106781186548,1.,0.707106781186548,1.,0.707106781186548,
1.,0.707106781186548,1.),(1.,0.707106781186548,1.,0.707106781186548,1.,
0.707106781186548,1.,0.707106781186548,1.)))
REPRESENTATION_ITEM('')
SURFACE()
);
#1087=(
BOUNDED_SURFACE()
B_SPLINE_SURFACE(5,2,((#50141,#50142,#50143,#50144,#50145,#50146,#50147,
#50148,#50149),(#50150,#50151,#50152,#50153,#50154,#50155,#50156,#50157,
#50158),(#50159,#50160,#50161,#50162,#50163,#50164,#50165,#50166,#50167),
(#50168,#50169,#50170,#50171,#50172,#50173,#50174,#50175,#50176),(#50177,
#50178,#50179,#50180,#50181,#50182,#50183,#50184,#50185),(#50186,#50187,
#50188,#50189,#50190,#50191,#50192,#50193,#50194),(#50195,#50196,#50197,
#50198,#50199,#50200,#50201,#50202,#50203),(#50204,#50205,#50206,#50207,
#50208,#50209,#50210,#50211,#50212),(#50213,#50214,#50215,#50216,#50217,
#50218,#50219,#50220,#50221),(#50222,#50223,#50224,#50225,#50226,#50227,
#50228,#50229,#50230),(#50231,#50232,#50233,#50234,#50235,#50236,#50237,
#50238,#50239),(#50240,#50241,#50242,#50243,#50244,#50245,#50246,#50247,
#50248),(#50249,#50250,#50251,#50252,#50253,#50254,#50255,#50256,#50257),
(#50258,#50259,#50260,#50261,#50262,#50263,#50264,#50265,#50266),(#50267,
#50268,#50269,#50270,#50271,#50272,#50273,#50274,#50275)),.UNSPECIFIED.,
 .F.,.T.,.F.)
B_SPLINE_SURFACE_WITH_KNOTS((6,1,1,1,1,1,1,1,1,1,6),(3,2,2,2,3),(-1.,-0.9,
-0.8,-0.7,-0.6,-0.5,-0.4,-0.3,-0.2,-0.1,0.),(0.,1.5707963267949,3.14159265358979,
4.71238898038469,6.28318530717959),.UNSPECIFIED.)
GEOMETRIC_REPRESENTATION_ITEM()
RATIONAL_B_SPLINE_SURFACE(((1.,0.707106781186548,1.,0.707106781186548,1.,
0.707106781186548,1.,0.707106781186548,1.),(1.,0.707106781186548,1.,0.707106781186548,
1.,0.707106781186548,1.,0.707106781186548,1.),(1.,0.707106781186548,1.,
0.707106781186548,1.,0.707106781186548,1.,0.707106781186548,1.),(1.,0.707106781186548,
1.,0.707106781186548,1.,0.707106781186548,1.,0.707106781186548,1.),(1.,
0.707106781186548,1.,0.707106781186548,1.,0.707106781186548,1.,0.707106781186548,
1.),(1.,0.707106781186548,1.,0.707106781186548,1.,0.707106781186548,1.,
0.707106781186548,1.),(1.,0.707106781186548,1.,0.707106781186548,1.,0.707106781186548,
1.,0.707106781186548,1.),(1.,0.707106781186548,1.,0.707106781186548,1.,
0.707106781186548,1.,0.707106781186548,1.),(1.,0.707106781186548,1.,0.707106781186548,
1.,0.707106781186548,1.,0.707106781186548,1.),(1.,0.707106781186548,1.,
0.707106781186548,1.,0.707106781186548,1.,0.707106781186548,1.),(1.,0.707106781186548,
1.,0.707106781186548,1.,0.707106781186548,1.,0.707106781186548,1.),(1.,
0.707106781186548,1.,0.707106781186548,1.,0.707106781186548,1.,0.707106781186548,
1.),(1.,0.707106781186548,1.,0.707106781186548,1.,0.707106781186548,1.,
0.707106781186548,1.),(1.,0.707106781186548,1.,0.707106781186548,1.,0.707106781186548,
1.,0.707106781186548,1.),(1.,0.707106781186548,1.,0.707106781186548,1.,
0.707106781186548,1.,0.707106781186548,1.)))
REPRESENTATION_ITEM('')
SURFACE()
);
#1088=(
BOUNDED_SURFACE()
B_SPLINE_SURFACE(5,2,((#50611,#50612,#50613,#50614,#50615,#50616,#50617,
#50618,#50619),(#50620,#50621,#50622,#50623,#50624,#50625,#50626,#50627,
#50628),(#50629,#50630,#50631,#50632,#50633,#50634,#50635,#50636,#50637),
(#50638,#50639,#50640,#50641,#50642,#50643,#50644,#50645,#50646),(#50647,
#50648,#50649,#50650,#50651,#50652,#50653,#50654,#50655),(#50656,#50657,
#50658,#50659,#50660,#50661,#50662,#50663,#50664),(#50665,#50666,#50667,
#50668,#50669,#50670,#50671,#50672,#50673),(#50674,#50675,#50676,#50677,
#50678,#50679,#50680,#50681,#50682),(#50683,#50684,#50685,#50686,#50687,
#50688,#50689,#50690,#50691),(#50692,#50693,#50694,#50695,#50696,#50697,
#50698,#50699,#50700),(#50701,#50702,#50703,#50704,#50705,#50706,#50707,
#50708,#50709),(#50710,#50711,#50712,#50713,#50714,#50715,#50716,#50717,
#50718),(#50719,#50720,#50721,#50722,#50723,#50724,#50725,#50726,#50727),
(#50728,#50729,#50730,#50731,#50732,#50733,#50734,#50735,#50736),(#50737,
#50738,#50739,#50740,#50741,#50742,#50743,#50744,#50745)),.UNSPECIFIED.,
 .F.,.T.,.F.)
B_SPLINE_SURFACE_WITH_KNOTS((6,1,1,1,1,1,1,1,1,1,6),(3,2,2,2,3),(-1.,-0.9,
-0.8,-0.7,-0.6,-0.5,-0.4,-0.3,-0.2,-0.1,0.),(0.,1.5707963267949,3.14159265358979,
4.71238898038469,6.28318530717959),.UNSPECIFIED.)
GEOMETRIC_REPRESENTATION_ITEM()
RATIONAL_B_SPLINE_SURFACE(((1.,0.707106781186548,1.,0.707106781186548,1.,
0.707106781186548,1.,0.707106781186548,1.),(1.,0.707106781186548,1.,0.707106781186548,
1.,0.707106781186548,1.,0.707106781186548,1.),(1.,0.707106781186548,1.,
0.707106781186548,1.,0.707106781186548,1.,0.707106781186548,1.),(1.,0.707106781186548,
1.,0.707106781186548,1.,0.707106781186548,1.,0.707106781186548,1.),(1.,
0.707106781186548,1.,0.707106781186548,1.,0.707106781186548,1.,0.707106781186548,
1.),(1.,0.707106781186548,1.,0.707106781186548,1.,0.707106781186548,1.,
0.707106781186548,1.),(1.,0.707106781186548,1.,0.707106781186548,1.,0.707106781186548,
1.,0.707106781186548,1.),(1.,0.707106781186548,1.,0.707106781186548,1.,
0.707106781186548,1.,0.707106781186548,1.),(1.,0.707106781186548,1.,0.707106781186548,
1.,0.707106781186548,1.,0.707106781186548,1.),(1.,0.707106781186548,1.,
0.707106781186548,1.,0.707106781186548,1.,0.707106781186548,1.),(1.,0.707106781186548,
1.,0.707106781186548,1.,0.707106781186548,1.,0.707106781186548,1.),(1.,
0.707106781186548,1.,0.707106781186548,1.,0.707106781186548,1.,0.707106781186548,
1.),(1.,0.707106781186548,1.,0.707106781186548,1.,0.707106781186548,1.,
0.707106781186548,1.),(1.,0.707106781186548,1.,0.707106781186548,1.,0.707106781186548,
1.,0.707106781186548,1.),(1.,0.707106781186548,1.,0.707106781186548,1.,
0.707106781186548,1.,0.707106781186548,1.)))
REPRESENTATION_ITEM('')
SURFACE()
);
#1089=(
BOUNDED_SURFACE()
B_SPLINE_SURFACE(5,2,((#51046,#51047,#51048,#51049,#51050,#51051,#51052,
#51053,#51054),(#51055,#51056,#51057,#51058,#51059,#51060,#51061,#51062,
#51063),(#51064,#51065,#51066,#51067,#51068,#51069,#51070,#51071,#51072),
(#51073,#51074,#51075,#51076,#51077,#51078,#51079,#51080,#51081),(#51082,
#51083,#51084,#51085,#51086,#51087,#51088,#51089,#51090),(#51091,#51092,
#51093,#51094,#51095,#51096,#51097,#51098,#51099),(#51100,#51101,#51102,
#51103,#51104,#51105,#51106,#51107,#51108),(#51109,#51110,#51111,#51112,
#51113,#51114,#51115,#51116,#51117),(#51118,#51119,#51120,#51121,#51122,
#51123,#51124,#51125,#51126),(#51127,#51128,#51129,#51130,#51131,#51132,
#51133,#51134,#51135),(#51136,#51137,#51138,#51139,#51140,#51141,#51142,
#51143,#51144),(#51145,#51146,#51147,#51148,#51149,#51150,#51151,#51152,
#51153),(#51154,#51155,#51156,#51157,#51158,#51159,#51160,#51161,#51162),
(#51163,#51164,#51165,#51166,#51167,#51168,#51169,#51170,#51171),(#51172,
#51173,#51174,#51175,#51176,#51177,#51178,#51179,#51180)),.UNSPECIFIED.,
 .F.,.T.,.F.)
B_SPLINE_SURFACE_WITH_KNOTS((6,1,1,1,1,1,1,1,1,1,6),(3,2,2,2,3),(-1.,-0.9,
-0.8,-0.7,-0.6,-0.5,-0.4,-0.3,-0.2,-0.1,0.),(0.,1.5707963267949,3.14159265358979,
4.71238898038469,6.28318530717959),.UNSPECIFIED.)
GEOMETRIC_REPRESENTATION_ITEM()
RATIONAL_B_SPLINE_SURFACE(((1.,0.707106781186548,1.,0.707106781186548,1.,
0.707106781186548,1.,0.707106781186548,1.),(1.,0.707106781186548,1.,0.707106781186548,
1.,0.707106781186548,1.,0.707106781186548,1.),(1.,0.707106781186548,1.,
0.707106781186548,1.,0.707106781186548,1.,0.707106781186548,1.),(1.,0.707106781186548,
1.,0.707106781186548,1.,0.707106781186548,1.,0.707106781186548,1.),(1.,
0.707106781186548,1.,0.707106781186548,1.,0.707106781186548,1.,0.707106781186548,
1.),(1.,0.707106781186548,1.,0.707106781186548,1.,0.707106781186548,1.,
0.707106781186548,1.),(1.,0.707106781186548,1.,0.707106781186548,1.,0.707106781186548,
1.,0.707106781186548,1.),(1.,0.707106781186548,1.,0.707106781186548,1.,
0.707106781186548,1.,0.707106781186548,1.),(1.,0.707106781186548,1.,0.707106781186548,
1.,0.707106781186548,1.,0.707106781186548,1.),(1.,0.707106781186548,1.,
0.707106781186548,1.,0.707106781186548,1.,0.707106781186548,1.),(1.,0.707106781186548,
1.,0.707106781186548,1.,0.707106781186548,1.,0.707106781186548,1.),(1.,
0.707106781186548,1.,0.707106781186548,1.,0.707106781186548,1.,0.707106781186548,
1.),(1.,0.707106781186548,1.,0.707106781186548,1.,0.707106781186548,1.,
0.707106781186548,1.),(1.,0.707106781186548,1.,0.707106781186548,1.,0.707106781186548,
1.,0.707106781186548,1.),(1.,0.707106781186548,1.,0.707106781186548,1.,
0.707106781186548,1.,0.707106781186548,1.)))
REPRESENTATION_ITEM('')
SURFACE()
);
#1090=(
BOUNDED_SURFACE()
B_SPLINE_SURFACE(5,2,((#51574,#51575,#51576,#51577,#51578,#51579,#51580,
#51581,#51582,#51583,#51584),(#51585,#51586,#51587,#51588,#51589,#51590,
#51591,#51592,#51593,#51594,#51595),(#51596,#51597,#51598,#51599,#51600,
#51601,#51602,#51603,#51604,#51605,#51606),(#51607,#51608,#51609,#51610,
#51611,#51612,#51613,#51614,#51615,#51616,#51617),(#51618,#51619,#51620,
#51621,#51622,#51623,#51624,#51625,#51626,#51627,#51628),(#51629,#51630,
#51631,#51632,#51633,#51634,#51635,#51636,#51637,#51638,#51639),(#51640,
#51641,#51642,#51643,#51644,#51645,#51646,#51647,#51648,#51649,#51650),
(#51651,#51652,#51653,#51654,#51655,#51656,#51657,#51658,#51659,#51660,
#51661),(#51662,#51663,#51664,#51665,#51666,#51667,#51668,#51669,#51670,
#51671,#51672),(#51673,#51674,#51675,#51676,#51677,#51678,#51679,#51680,
#51681,#51682,#51683),(#51684,#51685,#51686,#51687,#51688,#51689,#51690,
#51691,#51692,#51693,#51694),(#51695,#51696,#51697,#51698,#51699,#51700,
#51701,#51702,#51703,#51704,#51705),(#51706,#51707,#51708,#51709,#51710,
#51711,#51712,#51713,#51714,#51715,#51716),(#51717,#51718,#51719,#51720,
#51721,#51722,#51723,#51724,#51725,#51726,#51727),(#51728,#51729,#51730,
#51731,#51732,#51733,#51734,#51735,#51736,#51737,#51738),(#51739,#51740,
#51741,#51742,#51743,#51744,#51745,#51746,#51747,#51748,#51749),(#51750,
#51751,#51752,#51753,#51754,#51755,#51756,#51757,#51758,#51759,#51760),
(#51761,#51762,#51763,#51764,#51765,#51766,#51767,#51768,#51769,#51770,
#51771),(#51772,#51773,#51774,#51775,#51776,#51777,#51778,#51779,#51780,
#51781,#51782),(#51783,#51784,#51785,#51786,#51787,#51788,#51789,#51790,
#51791,#51792,#51793),(#51794,#51795,#51796,#51797,#51798,#51799,#51800,
#51801,#51802,#51803,#51804),(#51805,#51806,#51807,#51808,#51809,#51810,
#51811,#51812,#51813,#51814,#51815),(#51816,#51817,#51818,#51819,#51820,
#51821,#51822,#51823,#51824,#51825,#51826),(#51827,#51828,#51829,#51830,
#51831,#51832,#51833,#51834,#51835,#51836,#51837),(#51838,#51839,#51840,
#51841,#51842,#51843,#51844,#51845,#51846,#51847,#51848)),.UNSPECIFIED.,
 .F.,.T.,.F.)
B_SPLINE_SURFACE_WITH_KNOTS((6,1,1,1,1,1,1,1,1,1,1,1,1,1,1,1,1,1,1,1,6),
(3,2,2,2,2,3),(-1.,-0.95,-0.9,-0.85,-0.8,-0.75,-0.7,-0.65,-0.6,-0.55,-0.5,
-0.45,-0.4,-0.35,-0.3,-0.25,-0.2,-0.15,-0.1,-0.05,0.),(-0.960413254722853,
0.,1.5707963267949,3.14159265358979,4.71238898038469,5.32277205245673),
 .UNSPECIFIED.)
GEOMETRIC_REPRESENTATION_ITEM()
RATIONAL_B_SPLINE_SURFACE(((0.860825335104674,0.820919794139797,1.,0.707106781186548,
1.,0.707106781186548,1.,0.707106781186548,1.,0.88618698704675,0.860825335104674),
(0.860825335104674,0.820919794139797,1.,0.707106781186548,1.,0.707106781186548,
1.,0.707106781186548,1.,0.88618698704675,0.860825335104674),(0.860825335104674,
0.820919794139797,1.,0.707106781186548,1.,0.707106781186548,1.,0.707106781186548,
1.,0.88618698704675,0.860825335104674),(0.860825335104674,0.820919794139797,
1.,0.707106781186548,1.,0.707106781186548,1.,0.707106781186548,1.,0.88618698704675,
0.860825335104674),(0.860825335104674,0.820919794139797,1.,0.707106781186548,
1.,0.707106781186548,1.,0.707106781186548,1.,0.88618698704675,0.860825335104674),
(0.860825335104674,0.820919794139797,1.,0.707106781186548,1.,0.707106781186548,
1.,0.707106781186548,1.,0.88618698704675,0.860825335104674),(0.860825335104674,
0.820919794139797,1.,0.707106781186548,1.,0.707106781186548,1.,0.707106781186548,
1.,0.88618698704675,0.860825335104674),(0.860825335104674,0.820919794139797,
1.,0.707106781186548,1.,0.707106781186548,1.,0.707106781186548,1.,0.88618698704675,
0.860825335104674),(0.860825335104674,0.820919794139797,1.,0.707106781186548,
1.,0.707106781186548,1.,0.707106781186548,1.,0.88618698704675,0.860825335104674),
(0.860825335104674,0.820919794139797,1.,0.707106781186548,1.,0.707106781186548,
1.,0.707106781186548,1.,0.88618698704675,0.860825335104674),(0.860825335104674,
0.820919794139797,1.,0.707106781186548,1.,0.707106781186548,1.,0.707106781186548,
1.,0.88618698704675,0.860825335104674),(0.860825335104674,0.820919794139797,
1.,0.707106781186548,1.,0.707106781186548,1.,0.707106781186548,1.,0.88618698704675,
0.860825335104674),(0.860825335104674,0.820919794139797,1.,0.707106781186548,
1.,0.707106781186548,1.,0.707106781186548,1.,0.88618698704675,0.860825335104674),
(0.860825335104674,0.820919794139797,1.,0.707106781186548,1.,0.707106781186548,
1.,0.707106781186548,1.,0.88618698704675,0.860825335104674),(0.860825335104674,
0.820919794139797,1.,0.707106781186548,1.,0.707106781186548,1.,0.707106781186548,
1.,0.88618698704675,0.860825335104674),(0.860825335104674,0.820919794139797,
1.,0.707106781186548,1.,0.707106781186548,1.,0.707106781186548,1.,0.88618698704675,
0.860825335104674),(0.860825335104674,0.820919794139797,1.,0.707106781186548,
1.,0.707106781186548,1.,0.707106781186548,1.,0.88618698704675,0.860825335104674),
(0.860825335104674,0.820919794139797,1.,0.707106781186548,1.,0.707106781186548,
1.,0.707106781186548,1.,0.88618698704675,0.860825335104674),(0.860825335104674,
0.820919794139797,1.,0.707106781186548,1.,0.707106781186548,1.,0.707106781186548,
1.,0.88618698704675,0.860825335104674),(0.860825335104674,0.820919794139797,
1.,0.707106781186548,1.,0.707106781186548,1.,0.707106781186548,1.,0.88618698704675,
0.860825335104674),(0.860825335104674,0.820919794139797,1.,0.707106781186548,
1.,0.707106781186548,1.,0.707106781186548,1.,0.88618698704675,0.860825335104674),
(0.860825335104674,0.820919794139797,1.,0.707106781186548,1.,0.707106781186548,
1.,0.707106781186548,1.,0.88618698704675,0.860825335104674),(0.860825335104674,
0.820919794139797,1.,0.707106781186548,1.,0.707106781186548,1.,0.707106781186548,
1.,0.88618698704675,0.860825335104674),(0.860825335104674,0.820919794139797,
1.,0.707106781186548,1.,0.707106781186548,1.,0.707106781186548,1.,0.88618698704675,
0.860825335104674),(0.860825335104674,0.820919794139797,1.,0.707106781186548,
1.,0.707106781186548,1.,0.707106781186548,1.,0.88618698704675,0.860825335104674)))
REPRESENTATION_ITEM('')
SURFACE()
);
#1091=(
BOUNDED_SURFACE()
B_SPLINE_SURFACE(5,2,((#52396,#52397,#52398,#52399,#52400,#52401,#52402,
#52403,#52404,#52405,#52406),(#52407,#52408,#52409,#52410,#52411,#52412,
#52413,#52414,#52415,#52416,#52417),(#52418,#52419,#52420,#52421,#52422,
#52423,#52424,#52425,#52426,#52427,#52428),(#52429,#52430,#52431,#52432,
#52433,#52434,#52435,#52436,#52437,#52438,#52439),(#52440,#52441,#52442,
#52443,#52444,#52445,#52446,#52447,#52448,#52449,#52450),(#52451,#52452,
#52453,#52454,#52455,#52456,#52457,#52458,#52459,#52460,#52461),(#52462,
#52463,#52464,#52465,#52466,#52467,#52468,#52469,#52470,#52471,#52472),
(#52473,#52474,#52475,#52476,#52477,#52478,#52479,#52480,#52481,#52482,
#52483),(#52484,#52485,#52486,#52487,#52488,#52489,#52490,#52491,#52492,
#52493,#52494),(#52495,#52496,#52497,#52498,#52499,#52500,#52501,#52502,
#52503,#52504,#52505),(#52506,#52507,#52508,#52509,#52510,#52511,#52512,
#52513,#52514,#52515,#52516),(#52517,#52518,#52519,#52520,#52521,#52522,
#52523,#52524,#52525,#52526,#52527),(#52528,#52529,#52530,#52531,#52532,
#52533,#52534,#52535,#52536,#52537,#52538),(#52539,#52540,#52541,#52542,
#52543,#52544,#52545,#52546,#52547,#52548,#52549),(#52550,#52551,#52552,
#52553,#52554,#52555,#52556,#52557,#52558,#52559,#52560),(#52561,#52562,
#52563,#52564,#52565,#52566,#52567,#52568,#52569,#52570,#52571),(#52572,
#52573,#52574,#52575,#52576,#52577,#52578,#52579,#52580,#52581,#52582),
(#52583,#52584,#52585,#52586,#52587,#52588,#52589,#52590,#52591,#52592,
#52593),(#52594,#52595,#52596,#52597,#52598,#52599,#52600,#52601,#52602,
#52603,#52604),(#52605,#52606,#52607,#52608,#52609,#52610,#52611,#52612,
#52613,#52614,#52615),(#52616,#52617,#52618,#52619,#52620,#52621,#52622,
#52623,#52624,#52625,#52626),(#52627,#52628,#52629,#52630,#52631,#52632,
#52633,#52634,#52635,#52636,#52637),(#52638,#52639,#52640,#52641,#52642,
#52643,#52644,#52645,#52646,#52647,#52648),(#52649,#52650,#52651,#52652,
#52653,#52654,#52655,#52656,#52657,#52658,#52659),(#52660,#52661,#52662,
#52663,#52664,#52665,#52666,#52667,#52668,#52669,#52670)),.UNSPECIFIED.,
 .F.,.T.,.F.)
B_SPLINE_SURFACE_WITH_KNOTS((6,1,1,1,1,1,1,1,1,1,1,1,1,1,1,1,1,1,1,1,6),
(3,2,2,2,2,3),(-1.,-0.95,-0.9,-0.85,-0.8,-0.75,-0.7,-0.65,-0.6,-0.55,-0.5,
-0.45,-0.4,-0.35,-0.3,-0.25,-0.2,-0.15,-0.1,-0.05,0.),(-0.960413254722853,
0.,1.5707963267949,3.14159265358979,4.71238898038469,5.32277205245673),
 .UNSPECIFIED.)
GEOMETRIC_REPRESENTATION_ITEM()
RATIONAL_B_SPLINE_SURFACE(((0.860825335104674,0.820919794139797,1.,0.707106781186548,
1.,0.707106781186548,1.,0.707106781186548,1.,0.88618698704675,0.860825335104674),
(0.860825335104674,0.820919794139797,1.,0.707106781186548,1.,0.707106781186548,
1.,0.707106781186548,1.,0.88618698704675,0.860825335104674),(0.860825335104674,
0.820919794139797,1.,0.707106781186548,1.,0.707106781186548,1.,0.707106781186548,
1.,0.88618698704675,0.860825335104674),(0.860825335104674,0.820919794139797,
1.,0.707106781186548,1.,0.707106781186548,1.,0.707106781186548,1.,0.88618698704675,
0.860825335104674),(0.860825335104674,0.820919794139797,1.,0.707106781186548,
1.,0.707106781186548,1.,0.707106781186548,1.,0.88618698704675,0.860825335104674),
(0.860825335104674,0.820919794139797,1.,0.707106781186548,1.,0.707106781186548,
1.,0.707106781186548,1.,0.88618698704675,0.860825335104674),(0.860825335104674,
0.820919794139797,1.,0.707106781186548,1.,0.707106781186548,1.,0.707106781186548,
1.,0.88618698704675,0.860825335104674),(0.860825335104674,0.820919794139797,
1.,0.707106781186548,1.,0.707106781186548,1.,0.707106781186548,1.,0.88618698704675,
0.860825335104674),(0.860825335104674,0.820919794139797,1.,0.707106781186548,
1.,0.707106781186548,1.,0.707106781186548,1.,0.88618698704675,0.860825335104674),
(0.860825335104674,0.820919794139797,1.,0.707106781186548,1.,0.707106781186548,
1.,0.707106781186548,1.,0.88618698704675,0.860825335104674),(0.860825335104674,
0.820919794139797,1.,0.707106781186548,1.,0.707106781186548,1.,0.707106781186548,
1.,0.88618698704675,0.860825335104674),(0.860825335104674,0.820919794139797,
1.,0.707106781186548,1.,0.707106781186548,1.,0.707106781186548,1.,0.88618698704675,
0.860825335104674),(0.860825335104674,0.820919794139797,1.,0.707106781186548,
1.,0.707106781186548,1.,0.707106781186548,1.,0.88618698704675,0.860825335104674),
(0.860825335104674,0.820919794139797,1.,0.707106781186548,1.,0.707106781186548,
1.,0.707106781186548,1.,0.88618698704675,0.860825335104674),(0.860825335104674,
0.820919794139797,1.,0.707106781186548,1.,0.707106781186548,1.,0.707106781186548,
1.,0.88618698704675,0.860825335104674),(0.860825335104674,0.820919794139797,
1.,0.707106781186548,1.,0.707106781186548,1.,0.707106781186548,1.,0.88618698704675,
0.860825335104674),(0.860825335104674,0.820919794139797,1.,0.707106781186548,
1.,0.707106781186548,1.,0.707106781186548,1.,0.88618698704675,0.860825335104674),
(0.860825335104674,0.820919794139797,1.,0.707106781186548,1.,0.707106781186548,
1.,0.707106781186548,1.,0.88618698704675,0.860825335104674),(0.860825335104674,
0.820919794139797,1.,0.707106781186548,1.,0.707106781186548,1.,0.707106781186548,
1.,0.88618698704675,0.860825335104674),(0.860825335104674,0.820919794139797,
1.,0.707106781186548,1.,0.707106781186548,1.,0.707106781186548,1.,0.88618698704675,
0.860825335104674),(0.860825335104674,0.820919794139797,1.,0.707106781186548,
1.,0.707106781186548,1.,0.707106781186548,1.,0.88618698704675,0.860825335104674),
(0.860825335104674,0.820919794139797,1.,0.707106781186548,1.,0.707106781186548,
1.,0.707106781186548,1.,0.88618698704675,0.860825335104674),(0.860825335104674,
0.820919794139797,1.,0.707106781186548,1.,0.707106781186548,1.,0.707106781186548,
1.,0.88618698704675,0.860825335104674),(0.860825335104674,0.820919794139797,
1.,0.707106781186548,1.,0.707106781186548,1.,0.707106781186548,1.,0.88618698704675,
0.860825335104674),(0.860825335104674,0.820919794139797,1.,0.707106781186548,
1.,0.707106781186548,1.,0.707106781186548,1.,0.88618698704675,0.860825335104674)))
REPRESENTATION_ITEM('')
SURFACE()
);
#1092=(
BOUNDED_SURFACE()
B_SPLINE_SURFACE(5,2,((#53253,#53254,#53255,#53256,#53257,#53258,#53259,
#53260,#53261,#53262,#53263),(#53264,#53265,#53266,#53267,#53268,#53269,
#53270,#53271,#53272,#53273,#53274),(#53275,#53276,#53277,#53278,#53279,
#53280,#53281,#53282,#53283,#53284,#53285),(#53286,#53287,#53288,#53289,
#53290,#53291,#53292,#53293,#53294,#53295,#53296),(#53297,#53298,#53299,
#53300,#53301,#53302,#53303,#53304,#53305,#53306,#53307),(#53308,#53309,
#53310,#53311,#53312,#53313,#53314,#53315,#53316,#53317,#53318),(#53319,
#53320,#53321,#53322,#53323,#53324,#53325,#53326,#53327,#53328,#53329),
(#53330,#53331,#53332,#53333,#53334,#53335,#53336,#53337,#53338,#53339,
#53340),(#53341,#53342,#53343,#53344,#53345,#53346,#53347,#53348,#53349,
#53350,#53351),(#53352,#53353,#53354,#53355,#53356,#53357,#53358,#53359,
#53360,#53361,#53362),(#53363,#53364,#53365,#53366,#53367,#53368,#53369,
#53370,#53371,#53372,#53373),(#53374,#53375,#53376,#53377,#53378,#53379,
#53380,#53381,#53382,#53383,#53384),(#53385,#53386,#53387,#53388,#53389,
#53390,#53391,#53392,#53393,#53394,#53395),(#53396,#53397,#53398,#53399,
#53400,#53401,#53402,#53403,#53404,#53405,#53406),(#53407,#53408,#53409,
#53410,#53411,#53412,#53413,#53414,#53415,#53416,#53417),(#53418,#53419,
#53420,#53421,#53422,#53423,#53424,#53425,#53426,#53427,#53428),(#53429,
#53430,#53431,#53432,#53433,#53434,#53435,#53436,#53437,#53438,#53439),
(#53440,#53441,#53442,#53443,#53444,#53445,#53446,#53447,#53448,#53449,
#53450),(#53451,#53452,#53453,#53454,#53455,#53456,#53457,#53458,#53459,
#53460,#53461),(#53462,#53463,#53464,#53465,#53466,#53467,#53468,#53469,
#53470,#53471,#53472),(#53473,#53474,#53475,#53476,#53477,#53478,#53479,
#53480,#53481,#53482,#53483),(#53484,#53485,#53486,#53487,#53488,#53489,
#53490,#53491,#53492,#53493,#53494),(#53495,#53496,#53497,#53498,#53499,
#53500,#53501,#53502,#53503,#53504,#53505),(#53506,#53507,#53508,#53509,
#53510,#53511,#53512,#53513,#53514,#53515,#53516),(#53517,#53518,#53519,
#53520,#53521,#53522,#53523,#53524,#53525,#53526,#53527)),.UNSPECIFIED.,
 .F.,.T.,.F.)
B_SPLINE_SURFACE_WITH_KNOTS((6,1,1,1,1,1,1,1,1,1,1,1,1,1,1,1,1,1,1,1,6),
(3,2,2,2,2,3),(-1.,-0.95,-0.9,-0.85,-0.8,-0.75,-0.7,-0.65,-0.6,-0.55,-0.5,
-0.45,-0.4,-0.35,-0.3,-0.25,-0.2,-0.15,-0.1,-0.05,0.),(-0.960413254722853,
0.,1.5707963267949,3.14159265358979,4.71238898038469,5.32277205245673),
 .UNSPECIFIED.)
GEOMETRIC_REPRESENTATION_ITEM()
RATIONAL_B_SPLINE_SURFACE(((0.860825335104674,0.820919794139797,1.,0.707106781186548,
1.,0.707106781186548,1.,0.707106781186548,1.,0.88618698704675,0.860825335104674),
(0.860825335104674,0.820919794139797,1.,0.707106781186548,1.,0.707106781186548,
1.,0.707106781186548,1.,0.88618698704675,0.860825335104674),(0.860825335104674,
0.820919794139797,1.,0.707106781186548,1.,0.707106781186548,1.,0.707106781186548,
1.,0.88618698704675,0.860825335104674),(0.860825335104674,0.820919794139797,
1.,0.707106781186548,1.,0.707106781186548,1.,0.707106781186548,1.,0.88618698704675,
0.860825335104674),(0.860825335104674,0.820919794139797,1.,0.707106781186548,
1.,0.707106781186548,1.,0.707106781186548,1.,0.88618698704675,0.860825335104674),
(0.860825335104674,0.820919794139797,1.,0.707106781186548,1.,0.707106781186548,
1.,0.707106781186548,1.,0.88618698704675,0.860825335104674),(0.860825335104674,
0.820919794139797,1.,0.707106781186548,1.,0.707106781186548,1.,0.707106781186548,
1.,0.88618698704675,0.860825335104674),(0.860825335104674,0.820919794139797,
1.,0.707106781186548,1.,0.707106781186548,1.,0.707106781186548,1.,0.88618698704675,
0.860825335104674),(0.860825335104674,0.820919794139797,1.,0.707106781186548,
1.,0.707106781186548,1.,0.707106781186548,1.,0.88618698704675,0.860825335104674),
(0.860825335104674,0.820919794139797,1.,0.707106781186548,1.,0.707106781186548,
1.,0.707106781186548,1.,0.88618698704675,0.860825335104674),(0.860825335104674,
0.820919794139797,1.,0.707106781186548,1.,0.707106781186548,1.,0.707106781186548,
1.,0.88618698704675,0.860825335104674),(0.860825335104674,0.820919794139797,
1.,0.707106781186548,1.,0.707106781186548,1.,0.707106781186548,1.,0.88618698704675,
0.860825335104674),(0.860825335104674,0.820919794139797,1.,0.707106781186548,
1.,0.707106781186548,1.,0.707106781186548,1.,0.88618698704675,0.860825335104674),
(0.860825335104674,0.820919794139797,1.,0.707106781186548,1.,0.707106781186548,
1.,0.707106781186548,1.,0.88618698704675,0.860825335104674),(0.860825335104674,
0.820919794139797,1.,0.707106781186548,1.,0.707106781186548,1.,0.707106781186548,
1.,0.88618698704675,0.860825335104674),(0.860825335104674,0.820919794139797,
1.,0.707106781186548,1.,0.707106781186548,1.,0.707106781186548,1.,0.88618698704675,
0.860825335104674),(0.860825335104674,0.820919794139797,1.,0.707106781186548,
1.,0.707106781186548,1.,0.707106781186548,1.,0.88618698704675,0.860825335104674),
(0.860825335104674,0.820919794139797,1.,0.707106781186548,1.,0.707106781186548,
1.,0.707106781186548,1.,0.88618698704675,0.860825335104674),(0.860825335104674,
0.820919794139797,1.,0.707106781186548,1.,0.707106781186548,1.,0.707106781186548,
1.,0.88618698704675,0.860825335104674),(0.860825335104674,0.820919794139797,
1.,0.707106781186548,1.,0.707106781186548,1.,0.707106781186548,1.,0.88618698704675,
0.860825335104674),(0.860825335104674,0.820919794139797,1.,0.707106781186548,
1.,0.707106781186548,1.,0.707106781186548,1.,0.88618698704675,0.860825335104674),
(0.860825335104674,0.820919794139797,1.,0.707106781186548,1.,0.707106781186548,
1.,0.707106781186548,1.,0.88618698704675,0.860825335104674),(0.860825335104674,
0.820919794139797,1.,0.707106781186548,1.,0.707106781186548,1.,0.707106781186548,
1.,0.88618698704675,0.860825335104674),(0.860825335104674,0.820919794139797,
1.,0.707106781186548,1.,0.707106781186548,1.,0.707106781186548,1.,0.88618698704675,
0.860825335104674),(0.860825335104674,0.820919794139797,1.,0.707106781186548,
1.,0.707106781186548,1.,0.707106781186548,1.,0.88618698704675,0.860825335104674)))
REPRESENTATION_ITEM('')
SURFACE()
);
#1093=(
BOUNDED_SURFACE()
B_SPLINE_SURFACE(5,2,((#54070,#54071,#54072,#54073,#54074,#54075,#54076,
#54077,#54078,#54079,#54080),(#54081,#54082,#54083,#54084,#54085,#54086,
#54087,#54088,#54089,#54090,#54091),(#54092,#54093,#54094,#54095,#54096,
#54097,#54098,#54099,#54100,#54101,#54102),(#54103,#54104,#54105,#54106,
#54107,#54108,#54109,#54110,#54111,#54112,#54113),(#54114,#54115,#54116,
#54117,#54118,#54119,#54120,#54121,#54122,#54123,#54124),(#54125,#54126,
#54127,#54128,#54129,#54130,#54131,#54132,#54133,#54134,#54135),(#54136,
#54137,#54138,#54139,#54140,#54141,#54142,#54143,#54144,#54145,#54146),
(#54147,#54148,#54149,#54150,#54151,#54152,#54153,#54154,#54155,#54156,
#54157),(#54158,#54159,#54160,#54161,#54162,#54163,#54164,#54165,#54166,
#54167,#54168),(#54169,#54170,#54171,#54172,#54173,#54174,#54175,#54176,
#54177,#54178,#54179),(#54180,#54181,#54182,#54183,#54184,#54185,#54186,
#54187,#54188,#54189,#54190),(#54191,#54192,#54193,#54194,#54195,#54196,
#54197,#54198,#54199,#54200,#54201),(#54202,#54203,#54204,#54205,#54206,
#54207,#54208,#54209,#54210,#54211,#54212),(#54213,#54214,#54215,#54216,
#54217,#54218,#54219,#54220,#54221,#54222,#54223),(#54224,#54225,#54226,
#54227,#54228,#54229,#54230,#54231,#54232,#54233,#54234),(#54235,#54236,
#54237,#54238,#54239,#54240,#54241,#54242,#54243,#54244,#54245),(#54246,
#54247,#54248,#54249,#54250,#54251,#54252,#54253,#54254,#54255,#54256),
(#54257,#54258,#54259,#54260,#54261,#54262,#54263,#54264,#54265,#54266,
#54267),(#54268,#54269,#54270,#54271,#54272,#54273,#54274,#54275,#54276,
#54277,#54278),(#54279,#54280,#54281,#54282,#54283,#54284,#54285,#54286,
#54287,#54288,#54289),(#54290,#54291,#54292,#54293,#54294,#54295,#54296,
#54297,#54298,#54299,#54300),(#54301,#54302,#54303,#54304,#54305,#54306,
#54307,#54308,#54309,#54310,#54311),(#54312,#54313,#54314,#54315,#54316,
#54317,#54318,#54319,#54320,#54321,#54322),(#54323,#54324,#54325,#54326,
#54327,#54328,#54329,#54330,#54331,#54332,#54333),(#54334,#54335,#54336,
#54337,#54338,#54339,#54340,#54341,#54342,#54343,#54344)),.UNSPECIFIED.,
 .F.,.T.,.F.)
B_SPLINE_SURFACE_WITH_KNOTS((6,1,1,1,1,1,1,1,1,1,1,1,1,1,1,1,1,1,1,1,6),
(3,2,2,2,2,3),(-1.,-0.95,-0.9,-0.85,-0.8,-0.75,-0.7,-0.65,-0.6,-0.55,-0.5,
-0.45,-0.4,-0.35,-0.3,-0.25,-0.2,-0.15,-0.1,-0.05,0.),(-0.960413254722853,
0.,1.5707963267949,3.14159265358979,4.71238898038469,5.32277205245673),
 .UNSPECIFIED.)
GEOMETRIC_REPRESENTATION_ITEM()
RATIONAL_B_SPLINE_SURFACE(((0.860825335104674,0.820919794139797,1.,0.707106781186548,
1.,0.707106781186548,1.,0.707106781186548,1.,0.88618698704675,0.860825335104674),
(0.860825335104674,0.820919794139797,1.,0.707106781186548,1.,0.707106781186548,
1.,0.707106781186548,1.,0.88618698704675,0.860825335104674),(0.860825335104674,
0.820919794139797,1.,0.707106781186548,1.,0.707106781186548,1.,0.707106781186548,
1.,0.88618698704675,0.860825335104674),(0.860825335104674,0.820919794139797,
1.,0.707106781186548,1.,0.707106781186548,1.,0.707106781186548,1.,0.88618698704675,
0.860825335104674),(0.860825335104674,0.820919794139797,1.,0.707106781186548,
1.,0.707106781186548,1.,0.707106781186548,1.,0.88618698704675,0.860825335104674),
(0.860825335104674,0.820919794139797,1.,0.707106781186548,1.,0.707106781186548,
1.,0.707106781186548,1.,0.88618698704675,0.860825335104674),(0.860825335104674,
0.820919794139797,1.,0.707106781186548,1.,0.707106781186548,1.,0.707106781186548,
1.,0.88618698704675,0.860825335104674),(0.860825335104674,0.820919794139797,
1.,0.707106781186548,1.,0.707106781186548,1.,0.707106781186548,1.,0.88618698704675,
0.860825335104674),(0.860825335104674,0.820919794139797,1.,0.707106781186548,
1.,0.707106781186548,1.,0.707106781186548,1.,0.88618698704675,0.860825335104674),
(0.860825335104674,0.820919794139797,1.,0.707106781186548,1.,0.707106781186548,
1.,0.707106781186548,1.,0.88618698704675,0.860825335104674),(0.860825335104674,
0.820919794139797,1.,0.707106781186548,1.,0.707106781186548,1.,0.707106781186548,
1.,0.88618698704675,0.860825335104674),(0.860825335104674,0.820919794139797,
1.,0.707106781186548,1.,0.707106781186548,1.,0.707106781186548,1.,0.88618698704675,
0.860825335104674),(0.860825335104674,0.820919794139797,1.,0.707106781186548,
1.,0.707106781186548,1.,0.707106781186548,1.,0.88618698704675,0.860825335104674),
(0.860825335104674,0.820919794139797,1.,0.707106781186548,1.,0.707106781186548,
1.,0.707106781186548,1.,0.88618698704675,0.860825335104674),(0.860825335104674,
0.820919794139797,1.,0.707106781186548,1.,0.707106781186548,1.,0.707106781186548,
1.,0.88618698704675,0.860825335104674),(0.860825335104674,0.820919794139797,
1.,0.707106781186548,1.,0.707106781186548,1.,0.707106781186548,1.,0.88618698704675,
0.860825335104674),(0.860825335104674,0.820919794139797,1.,0.707106781186548,
1.,0.707106781186548,1.,0.707106781186548,1.,0.88618698704675,0.860825335104674),
(0.860825335104674,0.820919794139797,1.,0.707106781186548,1.,0.707106781186548,
1.,0.707106781186548,1.,0.88618698704675,0.860825335104674),(0.860825335104674,
0.820919794139797,1.,0.707106781186548,1.,0.707106781186548,1.,0.707106781186548,
1.,0.88618698704675,0.860825335104674),(0.860825335104674,0.820919794139797,
1.,0.707106781186548,1.,0.707106781186548,1.,0.707106781186548,1.,0.88618698704675,
0.860825335104674),(0.860825335104674,0.820919794139797,1.,0.707106781186548,
1.,0.707106781186548,1.,0.707106781186548,1.,0.88618698704675,0.860825335104674),
(0.860825335104674,0.820919794139797,1.,0.707106781186548,1.,0.707106781186548,
1.,0.707106781186548,1.,0.88618698704675,0.860825335104674),(0.860825335104674,
0.820919794139797,1.,0.707106781186548,1.,0.707106781186548,1.,0.707106781186548,
1.,0.88618698704675,0.860825335104674),(0.860825335104674,0.820919794139797,
1.,0.707106781186548,1.,0.707106781186548,1.,0.707106781186548,1.,0.88618698704675,
0.860825335104674),(0.860825335104674,0.820919794139797,1.,0.707106781186548,
1.,0.707106781186548,1.,0.707106781186548,1.,0.88618698704675,0.860825335104674)))
REPRESENTATION_ITEM('')
SURFACE()
);
#1094=(
BOUNDED_SURFACE()
B_SPLINE_SURFACE(5,2,((#54922,#54923,#54924,#54925,#54926,#54927,#54928,
#54929,#54930,#54931,#54932),(#54933,#54934,#54935,#54936,#54937,#54938,
#54939,#54940,#54941,#54942,#54943),(#54944,#54945,#54946,#54947,#54948,
#54949,#54950,#54951,#54952,#54953,#54954),(#54955,#54956,#54957,#54958,
#54959,#54960,#54961,#54962,#54963,#54964,#54965),(#54966,#54967,#54968,
#54969,#54970,#54971,#54972,#54973,#54974,#54975,#54976),(#54977,#54978,
#54979,#54980,#54981,#54982,#54983,#54984,#54985,#54986,#54987),(#54988,
#54989,#54990,#54991,#54992,#54993,#54994,#54995,#54996,#54997,#54998),
(#54999,#55000,#55001,#55002,#55003,#55004,#55005,#55006,#55007,#55008,
#55009),(#55010,#55011,#55012,#55013,#55014,#55015,#55016,#55017,#55018,
#55019,#55020),(#55021,#55022,#55023,#55024,#55025,#55026,#55027,#55028,
#55029,#55030,#55031),(#55032,#55033,#55034,#55035,#55036,#55037,#55038,
#55039,#55040,#55041,#55042),(#55043,#55044,#55045,#55046,#55047,#55048,
#55049,#55050,#55051,#55052,#55053),(#55054,#55055,#55056,#55057,#55058,
#55059,#55060,#55061,#55062,#55063,#55064),(#55065,#55066,#55067,#55068,
#55069,#55070,#55071,#55072,#55073,#55074,#55075),(#55076,#55077,#55078,
#55079,#55080,#55081,#55082,#55083,#55084,#55085,#55086),(#55087,#55088,
#55089,#55090,#55091,#55092,#55093,#55094,#55095,#55096,#55097),(#55098,
#55099,#55100,#55101,#55102,#55103,#55104,#55105,#55106,#55107,#55108),
(#55109,#55110,#55111,#55112,#55113,#55114,#55115,#55116,#55117,#55118,
#55119),(#55120,#55121,#55122,#55123,#55124,#55125,#55126,#55127,#55128,
#55129,#55130),(#55131,#55132,#55133,#55134,#55135,#55136,#55137,#55138,
#55139,#55140,#55141),(#55142,#55143,#55144,#55145,#55146,#55147,#55148,
#55149,#55150,#55151,#55152),(#55153,#55154,#55155,#55156,#55157,#55158,
#55159,#55160,#55161,#55162,#55163),(#55164,#55165,#55166,#55167,#55168,
#55169,#55170,#55171,#55172,#55173,#55174),(#55175,#55176,#55177,#55178,
#55179,#55180,#55181,#55182,#55183,#55184,#55185),(#55186,#55187,#55188,
#55189,#55190,#55191,#55192,#55193,#55194,#55195,#55196)),.UNSPECIFIED.,
 .F.,.T.,.F.)
B_SPLINE_SURFACE_WITH_KNOTS((6,1,1,1,1,1,1,1,1,1,1,1,1,1,1,1,1,1,1,1,6),
(3,2,2,2,2,3),(-1.,-0.95,-0.9,-0.85,-0.8,-0.75,-0.7,-0.65,-0.6,-0.55,-0.5,
-0.45,-0.4,-0.35,-0.3,-0.25,-0.2,-0.15,-0.1,-0.05,0.),(-0.960413254722853,
0.,1.5707963267949,3.14159265358979,4.71238898038469,5.32277205245673),
 .UNSPECIFIED.)
GEOMETRIC_REPRESENTATION_ITEM()
RATIONAL_B_SPLINE_SURFACE(((0.860825335104674,0.820919794139797,1.,0.707106781186548,
1.,0.707106781186548,1.,0.707106781186548,1.,0.88618698704675,0.860825335104674),
(0.860825335104674,0.820919794139797,1.,0.707106781186548,1.,0.707106781186548,
1.,0.707106781186548,1.,0.88618698704675,0.860825335104674),(0.860825335104674,
0.820919794139797,1.,0.707106781186548,1.,0.707106781186548,1.,0.707106781186548,
1.,0.88618698704675,0.860825335104674),(0.860825335104674,0.820919794139797,
1.,0.707106781186548,1.,0.707106781186548,1.,0.707106781186548,1.,0.88618698704675,
0.860825335104674),(0.860825335104674,0.820919794139797,1.,0.707106781186548,
1.,0.707106781186548,1.,0.707106781186548,1.,0.88618698704675,0.860825335104674),
(0.860825335104674,0.820919794139797,1.,0.707106781186548,1.,0.707106781186548,
1.,0.707106781186548,1.,0.88618698704675,0.860825335104674),(0.860825335104674,
0.820919794139797,1.,0.707106781186548,1.,0.707106781186548,1.,0.707106781186548,
1.,0.88618698704675,0.860825335104674),(0.860825335104674,0.820919794139797,
1.,0.707106781186548,1.,0.707106781186548,1.,0.707106781186548,1.,0.88618698704675,
0.860825335104674),(0.860825335104674,0.820919794139797,1.,0.707106781186548,
1.,0.707106781186548,1.,0.707106781186548,1.,0.88618698704675,0.860825335104674),
(0.860825335104674,0.820919794139797,1.,0.707106781186548,1.,0.707106781186548,
1.,0.707106781186548,1.,0.88618698704675,0.860825335104674),(0.860825335104674,
0.820919794139797,1.,0.707106781186548,1.,0.707106781186548,1.,0.707106781186548,
1.,0.88618698704675,0.860825335104674),(0.860825335104674,0.820919794139797,
1.,0.707106781186548,1.,0.707106781186548,1.,0.707106781186548,1.,0.88618698704675,
0.860825335104674),(0.860825335104674,0.820919794139797,1.,0.707106781186548,
1.,0.707106781186548,1.,0.707106781186548,1.,0.88618698704675,0.860825335104674),
(0.860825335104674,0.820919794139797,1.,0.707106781186548,1.,0.707106781186548,
1.,0.707106781186548,1.,0.88618698704675,0.860825335104674),(0.860825335104674,
0.820919794139797,1.,0.707106781186548,1.,0.707106781186548,1.,0.707106781186548,
1.,0.88618698704675,0.860825335104674),(0.860825335104674,0.820919794139797,
1.,0.707106781186548,1.,0.707106781186548,1.,0.707106781186548,1.,0.88618698704675,
0.860825335104674),(0.860825335104674,0.820919794139797,1.,0.707106781186548,
1.,0.707106781186548,1.,0.707106781186548,1.,0.88618698704675,0.860825335104674),
(0.860825335104674,0.820919794139797,1.,0.707106781186548,1.,0.707106781186548,
1.,0.707106781186548,1.,0.88618698704675,0.860825335104674),(0.860825335104674,
0.820919794139797,1.,0.707106781186548,1.,0.707106781186548,1.,0.707106781186548,
1.,0.88618698704675,0.860825335104674),(0.860825335104674,0.820919794139797,
1.,0.707106781186548,1.,0.707106781186548,1.,0.707106781186548,1.,0.88618698704675,
0.860825335104674),(0.860825335104674,0.820919794139797,1.,0.707106781186548,
1.,0.707106781186548,1.,0.707106781186548,1.,0.88618698704675,0.860825335104674),
(0.860825335104674,0.820919794139797,1.,0.707106781186548,1.,0.707106781186548,
1.,0.707106781186548,1.,0.88618698704675,0.860825335104674),(0.860825335104674,
0.820919794139797,1.,0.707106781186548,1.,0.707106781186548,1.,0.707106781186548,
1.,0.88618698704675,0.860825335104674),(0.860825335104674,0.820919794139797,
1.,0.707106781186548,1.,0.707106781186548,1.,0.707106781186548,1.,0.88618698704675,
0.860825335104674),(0.860825335104674,0.820919794139797,1.,0.707106781186548,
1.,0.707106781186548,1.,0.707106781186548,1.,0.88618698704675,0.860825335104674)))
REPRESENTATION_ITEM('')
SURFACE()
);
#1095=(
BOUNDED_SURFACE()
B_SPLINE_SURFACE(5,2,((#55744,#55745,#55746,#55747,#55748,#55749,#55750,
#55751,#55752,#55753,#55754),(#55755,#55756,#55757,#55758,#55759,#55760,
#55761,#55762,#55763,#55764,#55765),(#55766,#55767,#55768,#55769,#55770,
#55771,#55772,#55773,#55774,#55775,#55776),(#55777,#55778,#55779,#55780,
#55781,#55782,#55783,#55784,#55785,#55786,#55787),(#55788,#55789,#55790,
#55791,#55792,#55793,#55794,#55795,#55796,#55797,#55798),(#55799,#55800,
#55801,#55802,#55803,#55804,#55805,#55806,#55807,#55808,#55809),(#55810,
#55811,#55812,#55813,#55814,#55815,#55816,#55817,#55818,#55819,#55820),
(#55821,#55822,#55823,#55824,#55825,#55826,#55827,#55828,#55829,#55830,
#55831),(#55832,#55833,#55834,#55835,#55836,#55837,#55838,#55839,#55840,
#55841,#55842),(#55843,#55844,#55845,#55846,#55847,#55848,#55849,#55850,
#55851,#55852,#55853),(#55854,#55855,#55856,#55857,#55858,#55859,#55860,
#55861,#55862,#55863,#55864),(#55865,#55866,#55867,#55868,#55869,#55870,
#55871,#55872,#55873,#55874,#55875),(#55876,#55877,#55878,#55879,#55880,
#55881,#55882,#55883,#55884,#55885,#55886),(#55887,#55888,#55889,#55890,
#55891,#55892,#55893,#55894,#55895,#55896,#55897),(#55898,#55899,#55900,
#55901,#55902,#55903,#55904,#55905,#55906,#55907,#55908),(#55909,#55910,
#55911,#55912,#55913,#55914,#55915,#55916,#55917,#55918,#55919),(#55920,
#55921,#55922,#55923,#55924,#55925,#55926,#55927,#55928,#55929,#55930),
(#55931,#55932,#55933,#55934,#55935,#55936,#55937,#55938,#55939,#55940,
#55941),(#55942,#55943,#55944,#55945,#55946,#55947,#55948,#55949,#55950,
#55951,#55952),(#55953,#55954,#55955,#55956,#55957,#55958,#55959,#55960,
#55961,#55962,#55963),(#55964,#55965,#55966,#55967,#55968,#55969,#55970,
#55971,#55972,#55973,#55974),(#55975,#55976,#55977,#55978,#55979,#55980,
#55981,#55982,#55983,#55984,#55985),(#55986,#55987,#55988,#55989,#55990,
#55991,#55992,#55993,#55994,#55995,#55996),(#55997,#55998,#55999,#56000,
#56001,#56002,#56003,#56004,#56005,#56006,#56007),(#56008,#56009,#56010,
#56011,#56012,#56013,#56014,#56015,#56016,#56017,#56018)),.UNSPECIFIED.,
 .F.,.T.,.F.)
B_SPLINE_SURFACE_WITH_KNOTS((6,1,1,1,1,1,1,1,1,1,1,1,1,1,1,1,1,1,1,1,6),
(3,2,2,2,2,3),(-1.,-0.95,-0.9,-0.85,-0.8,-0.75,-0.7,-0.65,-0.6,-0.55,-0.5,
-0.45,-0.4,-0.35,-0.3,-0.25,-0.2,-0.15,-0.1,-0.05,0.),(-0.960413254722853,
0.,1.5707963267949,3.14159265358979,4.71238898038469,5.32277205245673),
 .UNSPECIFIED.)
GEOMETRIC_REPRESENTATION_ITEM()
RATIONAL_B_SPLINE_SURFACE(((0.860825335104674,0.820919794139797,1.,0.707106781186548,
1.,0.707106781186548,1.,0.707106781186548,1.,0.88618698704675,0.860825335104674),
(0.860825335104674,0.820919794139797,1.,0.707106781186548,1.,0.707106781186548,
1.,0.707106781186548,1.,0.88618698704675,0.860825335104674),(0.860825335104674,
0.820919794139797,1.,0.707106781186548,1.,0.707106781186548,1.,0.707106781186548,
1.,0.88618698704675,0.860825335104674),(0.860825335104674,0.820919794139797,
1.,0.707106781186548,1.,0.707106781186548,1.,0.707106781186548,1.,0.88618698704675,
0.860825335104674),(0.860825335104674,0.820919794139797,1.,0.707106781186548,
1.,0.707106781186548,1.,0.707106781186548,1.,0.88618698704675,0.860825335104674),
(0.860825335104674,0.820919794139797,1.,0.707106781186548,1.,0.707106781186548,
1.,0.707106781186548,1.,0.88618698704675,0.860825335104674),(0.860825335104674,
0.820919794139797,1.,0.707106781186548,1.,0.707106781186548,1.,0.707106781186548,
1.,0.88618698704675,0.860825335104674),(0.860825335104674,0.820919794139797,
1.,0.707106781186548,1.,0.707106781186548,1.,0.707106781186548,1.,0.88618698704675,
0.860825335104674),(0.860825335104674,0.820919794139797,1.,0.707106781186548,
1.,0.707106781186548,1.,0.707106781186548,1.,0.88618698704675,0.860825335104674),
(0.860825335104674,0.820919794139797,1.,0.707106781186548,1.,0.707106781186548,
1.,0.707106781186548,1.,0.88618698704675,0.860825335104674),(0.860825335104674,
0.820919794139797,1.,0.707106781186548,1.,0.707106781186548,1.,0.707106781186548,
1.,0.88618698704675,0.860825335104674),(0.860825335104674,0.820919794139797,
1.,0.707106781186548,1.,0.707106781186548,1.,0.707106781186548,1.,0.88618698704675,
0.860825335104674),(0.860825335104674,0.820919794139797,1.,0.707106781186548,
1.,0.707106781186548,1.,0.707106781186548,1.,0.88618698704675,0.860825335104674),
(0.860825335104674,0.820919794139797,1.,0.707106781186548,1.,0.707106781186548,
1.,0.707106781186548,1.,0.88618698704675,0.860825335104674),(0.860825335104674,
0.820919794139797,1.,0.707106781186548,1.,0.707106781186548,1.,0.707106781186548,
1.,0.88618698704675,0.860825335104674),(0.860825335104674,0.820919794139797,
1.,0.707106781186548,1.,0.707106781186548,1.,0.707106781186548,1.,0.88618698704675,
0.860825335104674),(0.860825335104674,0.820919794139797,1.,0.707106781186548,
1.,0.707106781186548,1.,0.707106781186548,1.,0.88618698704675,0.860825335104674),
(0.860825335104674,0.820919794139797,1.,0.707106781186548,1.,0.707106781186548,
1.,0.707106781186548,1.,0.88618698704675,0.860825335104674),(0.860825335104674,
0.820919794139797,1.,0.707106781186548,1.,0.707106781186548,1.,0.707106781186548,
1.,0.88618698704675,0.860825335104674),(0.860825335104674,0.820919794139797,
1.,0.707106781186548,1.,0.707106781186548,1.,0.707106781186548,1.,0.88618698704675,
0.860825335104674),(0.860825335104674,0.820919794139797,1.,0.707106781186548,
1.,0.707106781186548,1.,0.707106781186548,1.,0.88618698704675,0.860825335104674),
(0.860825335104674,0.820919794139797,1.,0.707106781186548,1.,0.707106781186548,
1.,0.707106781186548,1.,0.88618698704675,0.860825335104674),(0.860825335104674,
0.820919794139797,1.,0.707106781186548,1.,0.707106781186548,1.,0.707106781186548,
1.,0.88618698704675,0.860825335104674),(0.860825335104674,0.820919794139797,
1.,0.707106781186548,1.,0.707106781186548,1.,0.707106781186548,1.,0.88618698704675,
0.860825335104674),(0.860825335104674,0.820919794139797,1.,0.707106781186548,
1.,0.707106781186548,1.,0.707106781186548,1.,0.88618698704675,0.860825335104674)))
REPRESENTATION_ITEM('')
SURFACE()
);
#1096=(
BOUNDED_SURFACE()
B_SPLINE_SURFACE(5,2,((#56254,#56255,#56256,#56257,#56258,#56259,#56260,
#56261,#56262),(#56263,#56264,#56265,#56266,#56267,#56268,#56269,#56270,
#56271),(#56272,#56273,#56274,#56275,#56276,#56277,#56278,#56279,#56280),
(#56281,#56282,#56283,#56284,#56285,#56286,#56287,#56288,#56289),(#56290,
#56291,#56292,#56293,#56294,#56295,#56296,#56297,#56298),(#56299,#56300,
#56301,#56302,#56303,#56304,#56305,#56306,#56307),(#56308,#56309,#56310,
#56311,#56312,#56313,#56314,#56315,#56316),(#56317,#56318,#56319,#56320,
#56321,#56322,#56323,#56324,#56325),(#56326,#56327,#56328,#56329,#56330,
#56331,#56332,#56333,#56334),(#56335,#56336,#56337,#56338,#56339,#56340,
#56341,#56342,#56343),(#56344,#56345,#56346,#56347,#56348,#56349,#56350,
#56351,#56352),(#56353,#56354,#56355,#56356,#56357,#56358,#56359,#56360,
#56361),(#56362,#56363,#56364,#56365,#56366,#56367,#56368,#56369,#56370),
(#56371,#56372,#56373,#56374,#56375,#56376,#56377,#56378,#56379),(#56380,
#56381,#56382,#56383,#56384,#56385,#56386,#56387,#56388),(#56389,#56390,
#56391,#56392,#56393,#56394,#56395,#56396,#56397),(#56398,#56399,#56400,
#56401,#56402,#56403,#56404,#56405,#56406),(#56407,#56408,#56409,#56410,
#56411,#56412,#56413,#56414,#56415),(#56416,#56417,#56418,#56419,#56420,
#56421,#56422,#56423,#56424),(#56425,#56426,#56427,#56428,#56429,#56430,
#56431,#56432,#56433),(#56434,#56435,#56436,#56437,#56438,#56439,#56440,
#56441,#56442),(#56443,#56444,#56445,#56446,#56447,#56448,#56449,#56450,
#56451),(#56452,#56453,#56454,#56455,#56456,#56457,#56458,#56459,#56460),
(#56461,#56462,#56463,#56464,#56465,#56466,#56467,#56468,#56469),(#56470,
#56471,#56472,#56473,#56474,#56475,#56476,#56477,#56478),(#56479,#56480,
#56481,#56482,#56483,#56484,#56485,#56486,#56487),(#56488,#56489,#56490,
#56491,#56492,#56493,#56494,#56495,#56496),(#56497,#56498,#56499,#56500,
#56501,#56502,#56503,#56504,#56505),(#56506,#56507,#56508,#56509,#56510,
#56511,#56512,#56513,#56514),(#56515,#56516,#56517,#56518,#56519,#56520,
#56521,#56522,#56523)),.UNSPECIFIED.,.F.,.T.,.F.)
B_SPLINE_SURFACE_WITH_KNOTS((6,1,1,1,1,1,1,1,1,1,1,1,1,1,1,1,1,1,1,1,1,
1,1,1,1,6),(3,2,2,2,3),(-1.,-0.96,-0.92,-0.88,-0.84,-0.8,-0.76,-0.72,-0.68,
-0.64,-0.6,-0.56,-0.52,-0.48,-0.44,-0.4,-0.36,-0.32,-0.28,-0.24,-0.2,-0.16,
-0.12,-0.08,-0.04,0.),(0.,1.5707963267949,3.14159265358979,4.71238898038469,
6.28318530717959),.UNSPECIFIED.)
GEOMETRIC_REPRESENTATION_ITEM()
RATIONAL_B_SPLINE_SURFACE(((1.,0.707106781186548,1.,0.707106781186548,1.,
0.707106781186548,1.,0.707106781186548,1.),(1.,0.707106781186548,1.,0.707106781186548,
1.,0.707106781186548,1.,0.707106781186548,1.),(1.,0.707106781186548,1.,
0.707106781186548,1.,0.707106781186548,1.,0.707106781186548,1.),(1.,0.707106781186548,
1.,0.707106781186548,1.,0.707106781186548,1.,0.707106781186548,1.),(1.,
0.707106781186548,1.,0.707106781186548,1.,0.707106781186548,1.,0.707106781186548,
1.),(1.,0.707106781186548,1.,0.707106781186548,1.,0.707106781186548,1.,
0.707106781186548,1.),(1.,0.707106781186548,1.,0.707106781186548,1.,0.707106781186548,
1.,0.707106781186548,1.),(1.,0.707106781186548,1.,0.707106781186548,1.,
0.707106781186548,1.,0.707106781186548,1.),(1.,0.707106781186548,1.,0.707106781186548,
1.,0.707106781186548,1.,0.707106781186548,1.),(1.,0.707106781186548,1.,
0.707106781186548,1.,0.707106781186548,1.,0.707106781186548,1.),(1.,0.707106781186548,
1.,0.707106781186548,1.,0.707106781186548,1.,0.707106781186548,1.),(1.,
0.707106781186548,1.,0.707106781186548,1.,0.707106781186548,1.,0.707106781186548,
1.),(1.,0.707106781186548,1.,0.707106781186548,1.,0.707106781186548,1.,
0.707106781186548,1.),(1.,0.707106781186548,1.,0.707106781186548,1.,0.707106781186548,
1.,0.707106781186548,1.),(1.,0.707106781186548,1.,0.707106781186548,1.,
0.707106781186548,1.,0.707106781186548,1.),(1.,0.707106781186548,1.,0.707106781186548,
1.,0.707106781186548,1.,0.707106781186548,1.),(1.,0.707106781186548,1.,
0.707106781186548,1.,0.707106781186548,1.,0.707106781186548,1.),(1.,0.707106781186548,
1.,0.707106781186548,1.,0.707106781186548,1.,0.707106781186548,1.),(1.,
0.707106781186548,1.,0.707106781186548,1.,0.707106781186548,1.,0.707106781186548,
1.),(1.,0.707106781186548,1.,0.707106781186548,1.,0.707106781186548,1.,
0.707106781186548,1.),(1.,0.707106781186548,1.,0.707106781186548,1.,0.707106781186548,
1.,0.707106781186548,1.),(1.,0.707106781186548,1.,0.707106781186548,1.,
0.707106781186548,1.,0.707106781186548,1.),(1.,0.707106781186548,1.,0.707106781186548,
1.,0.707106781186548,1.,0.707106781186548,1.),(1.,0.707106781186548,1.,
0.707106781186548,1.,0.707106781186548,1.,0.707106781186548,1.),(1.,0.707106781186548,
1.,0.707106781186548,1.,0.707106781186548,1.,0.707106781186548,1.),(1.,
0.707106781186548,1.,0.707106781186548,1.,0.707106781186548,1.,0.707106781186548,
1.),(1.,0.707106781186548,1.,0.707106781186548,1.,0.707106781186548,1.,
0.707106781186548,1.),(1.,0.707106781186548,1.,0.707106781186548,1.,0.707106781186548,
1.,0.707106781186548,1.),(1.,0.707106781186548,1.,0.707106781186548,1.,
0.707106781186548,1.,0.707106781186548,1.),(1.,0.707106781186548,1.,0.707106781186548,
1.,0.707106781186548,1.,0.707106781186548,1.)))
REPRESENTATION_ITEM('')
SURFACE()
);
#1097=(
BOUNDED_SURFACE()
B_SPLINE_SURFACE(5,2,((#56834,#56835,#56836,#56837,#56838,#56839,#56840,
#56841,#56842,#56843,#56844),(#56845,#56846,#56847,#56848,#56849,#56850,
#56851,#56852,#56853,#56854,#56855),(#56856,#56857,#56858,#56859,#56860,
#56861,#56862,#56863,#56864,#56865,#56866),(#56867,#56868,#56869,#56870,
#56871,#56872,#56873,#56874,#56875,#56876,#56877),(#56878,#56879,#56880,
#56881,#56882,#56883,#56884,#56885,#56886,#56887,#56888),(#56889,#56890,
#56891,#56892,#56893,#56894,#56895,#56896,#56897,#56898,#56899),(#56900,
#56901,#56902,#56903,#56904,#56905,#56906,#56907,#56908,#56909,#56910),
(#56911,#56912,#56913,#56914,#56915,#56916,#56917,#56918,#56919,#56920,
#56921),(#56922,#56923,#56924,#56925,#56926,#56927,#56928,#56929,#56930,
#56931,#56932),(#56933,#56934,#56935,#56936,#56937,#56938,#56939,#56940,
#56941,#56942,#56943),(#56944,#56945,#56946,#56947,#56948,#56949,#56950,
#56951,#56952,#56953,#56954),(#56955,#56956,#56957,#56958,#56959,#56960,
#56961,#56962,#56963,#56964,#56965),(#56966,#56967,#56968,#56969,#56970,
#56971,#56972,#56973,#56974,#56975,#56976),(#56977,#56978,#56979,#56980,
#56981,#56982,#56983,#56984,#56985,#56986,#56987),(#56988,#56989,#56990,
#56991,#56992,#56993,#56994,#56995,#56996,#56997,#56998),(#56999,#57000,
#57001,#57002,#57003,#57004,#57005,#57006,#57007,#57008,#57009),(#57010,
#57011,#57012,#57013,#57014,#57015,#57016,#57017,#57018,#57019,#57020),
(#57021,#57022,#57023,#57024,#57025,#57026,#57027,#57028,#57029,#57030,
#57031),(#57032,#57033,#57034,#57035,#57036,#57037,#57038,#57039,#57040,
#57041,#57042),(#57043,#57044,#57045,#57046,#57047,#57048,#57049,#57050,
#57051,#57052,#57053),(#57054,#57055,#57056,#57057,#57058,#57059,#57060,
#57061,#57062,#57063,#57064),(#57065,#57066,#57067,#57068,#57069,#57070,
#57071,#57072,#57073,#57074,#57075),(#57076,#57077,#57078,#57079,#57080,
#57081,#57082,#57083,#57084,#57085,#57086),(#57087,#57088,#57089,#57090,
#57091,#57092,#57093,#57094,#57095,#57096,#57097),(#57098,#57099,#57100,
#57101,#57102,#57103,#57104,#57105,#57106,#57107,#57108)),.UNSPECIFIED.,
 .F.,.T.,.F.)
B_SPLINE_SURFACE_WITH_KNOTS((6,1,1,1,1,1,1,1,1,1,1,1,1,1,1,1,1,1,1,1,6),
(3,2,2,2,2,3),(-1.,-0.95,-0.9,-0.85,-0.8,-0.75,-0.7,-0.65,-0.6,-0.55,-0.5,
-0.45,-0.4,-0.35,-0.3,-0.25,-0.2,-0.15,-0.1,-0.05,0.),(-0.960413254722853,
0.,1.5707963267949,3.14159265358979,4.71238898038469,5.32277205245673),
 .UNSPECIFIED.)
GEOMETRIC_REPRESENTATION_ITEM()
RATIONAL_B_SPLINE_SURFACE(((0.860825335104674,0.820919794139797,1.,0.707106781186548,
1.,0.707106781186548,1.,0.707106781186548,1.,0.88618698704675,0.860825335104674),
(0.860825335104674,0.820919794139797,1.,0.707106781186548,1.,0.707106781186548,
1.,0.707106781186548,1.,0.88618698704675,0.860825335104674),(0.860825335104674,
0.820919794139797,1.,0.707106781186548,1.,0.707106781186548,1.,0.707106781186548,
1.,0.88618698704675,0.860825335104674),(0.860825335104674,0.820919794139797,
1.,0.707106781186548,1.,0.707106781186548,1.,0.707106781186548,1.,0.88618698704675,
0.860825335104674),(0.860825335104674,0.820919794139797,1.,0.707106781186548,
1.,0.707106781186548,1.,0.707106781186548,1.,0.88618698704675,0.860825335104674),
(0.860825335104674,0.820919794139797,1.,0.707106781186548,1.,0.707106781186548,
1.,0.707106781186548,1.,0.88618698704675,0.860825335104674),(0.860825335104674,
0.820919794139797,1.,0.707106781186548,1.,0.707106781186548,1.,0.707106781186548,
1.,0.88618698704675,0.860825335104674),(0.860825335104674,0.820919794139797,
1.,0.707106781186548,1.,0.707106781186548,1.,0.707106781186548,1.,0.88618698704675,
0.860825335104674),(0.860825335104674,0.820919794139797,1.,0.707106781186548,
1.,0.707106781186548,1.,0.707106781186548,1.,0.88618698704675,0.860825335104674),
(0.860825335104674,0.820919794139797,1.,0.707106781186548,1.,0.707106781186548,
1.,0.707106781186548,1.,0.88618698704675,0.860825335104674),(0.860825335104674,
0.820919794139797,1.,0.707106781186548,1.,0.707106781186548,1.,0.707106781186548,
1.,0.88618698704675,0.860825335104674),(0.860825335104674,0.820919794139797,
1.,0.707106781186548,1.,0.707106781186548,1.,0.707106781186548,1.,0.88618698704675,
0.860825335104674),(0.860825335104674,0.820919794139797,1.,0.707106781186548,
1.,0.707106781186548,1.,0.707106781186548,1.,0.88618698704675,0.860825335104674),
(0.860825335104674,0.820919794139797,1.,0.707106781186548,1.,0.707106781186548,
1.,0.707106781186548,1.,0.88618698704675,0.860825335104674),(0.860825335104674,
0.820919794139797,1.,0.707106781186548,1.,0.707106781186548,1.,0.707106781186548,
1.,0.88618698704675,0.860825335104674),(0.860825335104674,0.820919794139797,
1.,0.707106781186548,1.,0.707106781186548,1.,0.707106781186548,1.,0.88618698704675,
0.860825335104674),(0.860825335104674,0.820919794139797,1.,0.707106781186548,
1.,0.707106781186548,1.,0.707106781186548,1.,0.88618698704675,0.860825335104674),
(0.860825335104674,0.820919794139797,1.,0.707106781186548,1.,0.707106781186548,
1.,0.707106781186548,1.,0.88618698704675,0.860825335104674),(0.860825335104674,
0.820919794139797,1.,0.707106781186548,1.,0.707106781186548,1.,0.707106781186548,
1.,0.88618698704675,0.860825335104674),(0.860825335104674,0.820919794139797,
1.,0.707106781186548,1.,0.707106781186548,1.,0.707106781186548,1.,0.88618698704675,
0.860825335104674),(0.860825335104674,0.820919794139797,1.,0.707106781186548,
1.,0.707106781186548,1.,0.707106781186548,1.,0.88618698704675,0.860825335104674),
(0.860825335104674,0.820919794139797,1.,0.707106781186548,1.,0.707106781186548,
1.,0.707106781186548,1.,0.88618698704675,0.860825335104674),(0.860825335104674,
0.820919794139797,1.,0.707106781186548,1.,0.707106781186548,1.,0.707106781186548,
1.,0.88618698704675,0.860825335104674),(0.860825335104674,0.820919794139797,
1.,0.707106781186548,1.,0.707106781186548,1.,0.707106781186548,1.,0.88618698704675,
0.860825335104674),(0.860825335104674,0.820919794139797,1.,0.707106781186548,
1.,0.707106781186548,1.,0.707106781186548,1.,0.88618698704675,0.860825335104674)))
REPRESENTATION_ITEM('')
SURFACE()
);
#1301=STYLED_ITEM('',(#60520),#93);
#1895=FACE_OUTER_BOUND('',#2903,.T.);
#1896=FACE_OUTER_BOUND('',#2904,.T.);
#1897=FACE_OUTER_BOUND('',#2905,.T.);
#1898=FACE_OUTER_BOUND('',#2906,.T.);
#1899=FACE_OUTER_BOUND('',#2907,.T.);
#1900=FACE_OUTER_BOUND('',#2908,.T.);
#1901=FACE_OUTER_BOUND('',#2909,.T.);
#1902=FACE_OUTER_BOUND('',#2910,.T.);
#1903=FACE_OUTER_BOUND('',#2911,.T.);
#1904=FACE_OUTER_BOUND('',#2912,.T.);
#1905=FACE_OUTER_BOUND('',#2913,.T.);
#1906=FACE_OUTER_BOUND('',#2914,.T.);
#1907=FACE_OUTER_BOUND('',#2915,.T.);
#1908=FACE_OUTER_BOUND('',#2916,.T.);
#1909=FACE_OUTER_BOUND('',#2917,.T.);
#1910=FACE_OUTER_BOUND('',#2918,.T.);
#1911=FACE_OUTER_BOUND('',#2919,.T.);
#1912=FACE_OUTER_BOUND('',#2920,.T.);
#1913=FACE_OUTER_BOUND('',#2921,.T.);
#1914=FACE_OUTER_BOUND('',#2923,.T.);
#1915=FACE_OUTER_BOUND('',#2924,.T.);
#1916=FACE_OUTER_BOUND('',#2926,.T.);
#1917=FACE_OUTER_BOUND('',#2927,.T.);
#1918=FACE_OUTER_BOUND('',#2928,.T.);
#1919=FACE_OUTER_BOUND('',#2929,.T.);
#1920=FACE_OUTER_BOUND('',#2930,.T.);
#1921=FACE_OUTER_BOUND('',#2931,.T.);
#1922=FACE_OUTER_BOUND('',#2932,.T.);
#1923=FACE_OUTER_BOUND('',#2933,.T.);
#1924=FACE_OUTER_BOUND('',#2934,.T.);
#1925=FACE_OUTER_BOUND('',#2935,.T.);
#1926=FACE_OUTER_BOUND('',#2936,.T.);
#1927=FACE_OUTER_BOUND('',#2937,.T.);
#1928=FACE_OUTER_BOUND('',#2938,.T.);
#1929=FACE_OUTER_BOUND('',#2939,.T.);
#1930=FACE_OUTER_BOUND('',#2940,.T.);
#1931=FACE_OUTER_BOUND('',#2941,.T.);
#1932=FACE_OUTER_BOUND('',#2942,.T.);
#1933=FACE_OUTER_BOUND('',#2943,.T.);
#1934=FACE_OUTER_BOUND('',#2944,.T.);
#1935=FACE_OUTER_BOUND('',#2945,.T.);
#1936=FACE_OUTER_BOUND('',#2946,.T.);
#1937=FACE_OUTER_BOUND('',#2947,.T.);
#1938=FACE_OUTER_BOUND('',#2948,.T.);
#1939=FACE_OUTER_BOUND('',#2949,.T.);
#1940=FACE_OUTER_BOUND('',#2950,.T.);
#1941=FACE_OUTER_BOUND('',#2951,.T.);
#1942=FACE_OUTER_BOUND('',#2952,.T.);
#1943=FACE_OUTER_BOUND('',#2953,.T.);
#1944=FACE_OUTER_BOUND('',#2954,.T.);
#1945=FACE_OUTER_BOUND('',#2955,.T.);
#1946=FACE_OUTER_BOUND('',#2956,.T.);
#1947=FACE_OUTER_BOUND('',#2957,.T.);
#1948=FACE_OUTER_BOUND('',#2958,.T.);
#1949=FACE_OUTER_BOUND('',#2959,.T.);
#1950=FACE_OUTER_BOUND('',#2960,.T.);
#1951=FACE_OUTER_BOUND('',#2961,.T.);
#1952=FACE_OUTER_BOUND('',#2962,.T.);
#1953=FACE_OUTER_BOUND('',#2963,.T.);
#1954=FACE_OUTER_BOUND('',#2964,.T.);
#1955=FACE_OUTER_BOUND('',#2965,.T.);
#1956=FACE_OUTER_BOUND('',#2966,.T.);
#1957=FACE_OUTER_BOUND('',#2967,.T.);
#1958=FACE_OUTER_BOUND('',#2968,.T.);
#1959=FACE_OUTER_BOUND('',#2969,.T.);
#1960=FACE_OUTER_BOUND('',#2970,.T.);
#1961=FACE_OUTER_BOUND('',#2971,.T.);
#1962=FACE_OUTER_BOUND('',#2972,.T.);
#1963=FACE_OUTER_BOUND('',#2973,.T.);
#1964=FACE_OUTER_BOUND('',#2974,.T.);
#1965=FACE_OUTER_BOUND('',#2975,.T.);
#1966=FACE_OUTER_BOUND('',#2976,.T.);
#1967=FACE_OUTER_BOUND('',#2977,.T.);
#1968=FACE_OUTER_BOUND('',#2978,.T.);
#1969=FACE_OUTER_BOUND('',#2979,.T.);
#1970=FACE_OUTER_BOUND('',#2980,.T.);
#1971=FACE_OUTER_BOUND('',#2981,.T.);
#1972=FACE_OUTER_BOUND('',#2982,.T.);
#1973=FACE_OUTER_BOUND('',#2983,.T.);
#1974=FACE_OUTER_BOUND('',#2984,.T.);
#1975=FACE_OUTER_BOUND('',#2985,.T.);
#1976=FACE_OUTER_BOUND('',#2986,.T.);
#1977=FACE_OUTER_BOUND('',#2987,.T.);
#1978=FACE_OUTER_BOUND('',#2988,.T.);
#1979=FACE_OUTER_BOUND('',#2989,.T.);
#1980=FACE_OUTER_BOUND('',#2990,.T.);
#1981=FACE_OUTER_BOUND('',#2991,.T.);
#1982=FACE_OUTER_BOUND('',#2992,.T.);
#1983=FACE_OUTER_BOUND('',#2993,.T.);
#1984=FACE_OUTER_BOUND('',#2994,.T.);
#1985=FACE_OUTER_BOUND('',#2995,.T.);
#1986=FACE_OUTER_BOUND('',#2996,.T.);
#1987=FACE_OUTER_BOUND('',#2997,.T.);
#1988=FACE_OUTER_BOUND('',#2998,.T.);
#1989=FACE_OUTER_BOUND('',#2999,.T.);
#1990=FACE_OUTER_BOUND('',#3000,.T.);
#2903=EDGE_LOOP('',(#15031,#15032,#15033,#15034,#15035,#15036,#15037,#15038));
#2904=EDGE_LOOP('',(#15039,#15040,#15041,#15042));
#2905=EDGE_LOOP('',(#15043,#15044,#15045,#15046,#15047,#15048,#15049,#15050,
#15051,#15052,#15053,#15054,#15055,#15056,#15057,#15058,#15059,#15060,#15061,
#15062,#15063,#15064,#15065,#15066,#15067,#15068,#15069,#15070,#15071,#15072,
#15073,#15074,#15075,#15076,#15077,#15078,#15079,#15080,#15081,#15082,#15083,
#15084,#15085,#15086,#15087,#15088,#15089,#15090,#15091,#15092,#15093,#15094,
#15095,#15096,#15097,#15098,#15099,#15100,#15101,#15102,#15103,#15104,#15105,
#15106,#15107,#15108,#15109,#15110,#15111,#15112,#15113,#15114,#15115,#15116,
#15117,#15118,#15119,#15120,#15121,#15122,#15123,#15124,#15125,#15126,#15127,
#15128,#15129,#15130));
#2906=EDGE_LOOP('',(#15131,#15132,#15133,#15134));
#2907=EDGE_LOOP('',(#15135,#15136,#15137,#15138));
#2908=EDGE_LOOP('',(#15139,#15140,#15141,#15142));
#2909=EDGE_LOOP('',(#15143,#15144,#15145,#15146));
#2910=EDGE_LOOP('',(#15147,#15148,#15149,#15150));
#2911=EDGE_LOOP('',(#15151,#15152,#15153,#15154));
#2912=EDGE_LOOP('',(#15155,#15156,#15157,#15158));
#2913=EDGE_LOOP('',(#15159,#15160,#15161,#15162));
#2914=EDGE_LOOP('',(#15163,#15164,#15165,#15166));
#2915=EDGE_LOOP('',(#15167,#15168,#15169,#15170));
#2916=EDGE_LOOP('',(#15171,#15172,#15173,#15174));
#2917=EDGE_LOOP('',(#15175,#15176,#15177,#15178));
#2918=EDGE_LOOP('',(#15179,#15180,#15181,#15182));
#2919=EDGE_LOOP('',(#15183,#15184,#15185,#15186,#15187));
#2920=EDGE_LOOP('',(#15188,#15189,#15190,#15191,#15192,#15193));
#2921=EDGE_LOOP('',(#15194));
#2922=EDGE_LOOP('',(#15195));
#2923=EDGE_LOOP('',(#15196,#15197,#15198,#15199,#15200));
#2924=EDGE_LOOP('',(#15201));
#2925=EDGE_LOOP('',(#15202));
#2926=EDGE_LOOP('',(#15203,#15204,#15205,#15206,#15207,#15208,#15209));
#2927=EDGE_LOOP('',(#15210,#15211,#15212,#15213));
#2928=EDGE_LOOP('',(#15214,#15215,#15216,#15217));
#2929=EDGE_LOOP('',(#15218,#15219,#15220,#15221,#15222,#15223,#15224));
#2930=EDGE_LOOP('',(#15225,#15226,#15227,#15228));
#2931=EDGE_LOOP('',(#15229,#15230,#15231,#15232,#15233,#15234,#15235));
#2932=EDGE_LOOP('',(#15236,#15237,#15238,#15239));
#2933=EDGE_LOOP('',(#15240,#15241,#15242,#15243));
#2934=EDGE_LOOP('',(#15244,#15245,#15246,#15247,#15248,#15249,#15250));
#2935=EDGE_LOOP('',(#15251,#15252,#15253,#15254));
#2936=EDGE_LOOP('',(#15255,#15256,#15257,#15258,#15259,#15260,#15261));
#2937=EDGE_LOOP('',(#15262,#15263,#15264,#15265));
#2938=EDGE_LOOP('',(#15266,#15267,#15268,#15269));
#2939=EDGE_LOOP('',(#15270,#15271,#15272,#15273,#15274,#15275,#15276));
#2940=EDGE_LOOP('',(#15277,#15278,#15279,#15280));
#2941=EDGE_LOOP('',(#15281,#15282,#15283,#15284,#15285,#15286,#15287));
#2942=EDGE_LOOP('',(#15288,#15289,#15290,#15291));
#2943=EDGE_LOOP('',(#15292,#15293,#15294,#15295,#15296));
#2944=EDGE_LOOP('',(#15297,#15298,#15299,#15300,#15301,#15302,#15303));
#2945=EDGE_LOOP('',(#15304,#15305,#15306,#15307));
#2946=EDGE_LOOP('',(#15308,#15309,#15310,#15311,#15312,#15313,#15314));
#2947=EDGE_LOOP('',(#15315,#15316,#15317,#15318));
#2948=EDGE_LOOP('',(#15319,#15320,#15321,#15322));
#2949=EDGE_LOOP('',(#15323,#15324,#15325,#15326,#15327,#15328,#15329));
#2950=EDGE_LOOP('',(#15330,#15331,#15332,#15333));
#2951=EDGE_LOOP('',(#15334,#15335,#15336,#15337,#15338,#15339,#15340));
#2952=EDGE_LOOP('',(#15341,#15342,#15343,#15344));
#2953=EDGE_LOOP('',(#15345,#15346,#15347,#15348));
#2954=EDGE_LOOP('',(#15349,#15350,#15351,#15352,#15353,#15354,#15355));
#2955=EDGE_LOOP('',(#15356,#15357,#15358,#15359));
#2956=EDGE_LOOP('',(#15360,#15361,#15362,#15363,#15364,#15365,#15366));
#2957=EDGE_LOOP('',(#15367,#15368,#15369,#15370));
#2958=EDGE_LOOP('',(#15371,#15372,#15373,#15374));
#2959=EDGE_LOOP('',(#15375,#15376,#15377,#15378,#15379,#15380,#15381));
#2960=EDGE_LOOP('',(#15382,#15383,#15384,#15385));
#2961=EDGE_LOOP('',(#15386,#15387,#15388,#15389,#15390,#15391,#15392,#15393));
#2962=EDGE_LOOP('',(#15394,#15395,#15396,#15397));
#2963=EDGE_LOOP('',(#15398,#15399,#15400,#15401,#15402));
#2964=EDGE_LOOP('',(#15403,#15404,#15405,#15406,#15407,#15408,#15409));
#2965=EDGE_LOOP('',(#15410,#15411,#15412,#15413));
#2966=EDGE_LOOP('',(#15414,#15415,#15416,#15417,#15418,#15419,#15420,#15421));
#2967=EDGE_LOOP('',(#15422,#15423,#15424,#15425));
#2968=EDGE_LOOP('',(#15426,#15427,#15428,#15429,#15430));
#2969=EDGE_LOOP('',(#15431,#15432,#15433,#15434,#15435,#15436,#15437));
#2970=EDGE_LOOP('',(#15438,#15439,#15440,#15441));
#2971=EDGE_LOOP('',(#15442,#15443,#15444,#15445,#15446,#15447,#15448,#15449));
#2972=EDGE_LOOP('',(#15450,#15451,#15452,#15453));
#2973=EDGE_LOOP('',(#15454,#15455,#15456,#15457,#15458));
#2974=EDGE_LOOP('',(#15459,#15460,#15461,#15462,#15463,#15464,#15465));
#2975=EDGE_LOOP('',(#15466,#15467,#15468,#15469));
#2976=EDGE_LOOP('',(#15470,#15471,#15472,#15473,#15474,#15475,#15476,#15477));
#2977=EDGE_LOOP('',(#15478,#15479,#15480,#15481));
#2978=EDGE_LOOP('',(#15482,#15483,#15484,#15485,#15486));
#2979=EDGE_LOOP('',(#15487,#15488,#15489,#15490,#15491,#15492,#15493));
#2980=EDGE_LOOP('',(#15494,#15495,#15496,#15497));
#2981=EDGE_LOOP('',(#15498,#15499,#15500,#15501,#15502,#15503,#15504,#15505));
#2982=EDGE_LOOP('',(#15506,#15507,#15508,#15509));
#2983=EDGE_LOOP('',(#15510,#15511,#15512,#15513,#15514));
#2984=EDGE_LOOP('',(#15515,#15516,#15517,#15518,#15519,#15520,#15521));
#2985=EDGE_LOOP('',(#15522,#15523,#15524,#15525));
#2986=EDGE_LOOP('',(#15526,#15527,#15528,#15529,#15530,#15531,#15532,#15533));
#2987=EDGE_LOOP('',(#15534,#15535,#15536,#15537,#15538));
#2988=EDGE_LOOP('',(#15539,#15540,#15541,#15542,#15543));
#2989=EDGE_LOOP('',(#15544,#15545,#15546,#15547,#15548,#15549,#15550,#15551));
#2990=EDGE_LOOP('',(#15552,#15553,#15554,#15555));
#2991=EDGE_LOOP('',(#15556,#15557,#15558,#15559,#15560,#15561,#15562,#15563,
#15564,#15565,#15566,#15567,#15568,#15569,#15570,#15571,#15572,#15573,#15574,
#15575,#15576,#15577,#15578,#15579,#15580,#15581,#15582,#15583,#15584,#15585,
#15586,#15587,#15588,#15589,#15590,#15591,#15592,#15593,#15594,#15595,#15596,
#15597,#15598,#15599,#15600,#15601,#15602,#15603,#15604,#15605,#15606,#15607,
#15608,#15609,#15610,#15611,#15612));
#2992=EDGE_LOOP('',(#15613,#15614,#15615,#15616,#15617,#15618,#15619,#15620,
#15621));
#2993=EDGE_LOOP('',(#15622,#15623,#15624,#15625));
#2994=EDGE_LOOP('',(#15626,#15627,#15628,#15629,#15630));
#2995=EDGE_LOOP('',(#15631,#15632,#15633,#15634,#15635,#15636,#15637));
#2996=EDGE_LOOP('',(#15638,#15639,#15640,#15641));
#2997=EDGE_LOOP('',(#15642,#15643,#15644,#15645));
#2998=EDGE_LOOP('',(#15646,#15647,#15648,#15649,#15650));
#2999=EDGE_LOOP('',(#15651,#15652,#15653,#15654));
#3000=EDGE_LOOP('',(#15655,#15656,#15657,#15658));
#3568=CIRCLE('',#19232,37.6);
#3569=CIRCLE('',#19233,37.6);
#3570=CIRCLE('',#19235,39.);
#3571=CIRCLE('',#19236,38.540427484991);
#3572=CIRCLE('',#19238,39.);
#3573=CIRCLE('',#19239,39.);
#3574=CIRCLE('',#19240,39.);
#3575=CIRCLE('',#19241,39.);
#3576=CIRCLE('',#19242,39.);
#3577=CIRCLE('',#19243,39.);
#3578=CIRCLE('',#19244,39.);
#3579=CIRCLE('',#19245,39.);
#3580=CIRCLE('',#19246,39.);
#3581=CIRCLE('',#19247,39.);
#3582=CIRCLE('',#19248,39.);
#3583=CIRCLE('',#19249,39.);
#3584=CIRCLE('',#19250,39.);
#3585=CIRCLE('',#19251,39.);
#3586=CIRCLE('',#19252,39.);
#3587=CIRCLE('',#19253,39.);
#3588=CIRCLE('',#19254,39.);
#3589=CIRCLE('',#19255,39.);
#3590=CIRCLE('',#19256,39.);
#3591=CIRCLE('',#19257,39.);
#3592=CIRCLE('',#19258,39.);
#3593=CIRCLE('',#19259,39.);
#3594=CIRCLE('',#19260,39.);
#3595=CIRCLE('',#19261,39.);
#3596=CIRCLE('',#19262,39.);
#3597=CIRCLE('',#19263,39.);
#3598=CIRCLE('',#19264,39.);
#3599=CIRCLE('',#19265,39.);
#3600=CIRCLE('',#19266,39.);
#3601=CIRCLE('',#19268,38.540427484991);
#3602=CIRCLE('',#19270,38.540427484991);
#3603=CIRCLE('',#19272,38.540427484991);
#3604=CIRCLE('',#19274,38.540427484991);
#3605=CIRCLE('',#19276,38.540427484991);
#3606=CIRCLE('',#19278,38.540427484991);
#3607=CIRCLE('',#19280,38.540427484991);
#3608=CIRCLE('',#19282,38.540427484991);
#3609=CIRCLE('',#19284,38.540427484991);
#3610=CIRCLE('',#19286,38.540427484991);
#3611=CIRCLE('',#19288,38.540427484991);
#3612=CIRCLE('',#19290,38.540427484991);
#3613=CIRCLE('',#19292,38.540427484991);
#3614=CIRCLE('',#19294,3.825);
#3615=CIRCLE('',#19295,3.525);
#3616=CIRCLE('',#19296,3.525);
#3617=CIRCLE('',#19298,3.525);
#3618=CIRCLE('',#19299,3.525);
#3619=CIRCLE('',#19301,38.5);
#3620=CIRCLE('',#19303,3.825);
#3621=CIRCLE('',#19305,8.1);
#3622=CIRCLE('',#19307,30.6);
#3623=CIRCLE('',#19309,37.6);
#3624=CIRCLE('',#19311,30.6);
#3625=CIRCLE('',#19313,37.6);
#3626=CIRCLE('',#19315,30.6);
#3627=CIRCLE('',#19317,37.6);
#3628=CIRCLE('',#19319,30.6);
#3629=CIRCLE('',#19321,37.6);
#3630=CIRCLE('',#19323,30.6);
#3631=CIRCLE('',#19325,37.6);
#3632=CIRCLE('',#19327,30.6);
#3633=CIRCLE('',#19329,37.6);
#3634=CIRCLE('',#19331,30.6);
#3635=CIRCLE('',#19334,27.);
#3636=CIRCLE('',#19336,37.6);
#3637=CIRCLE('',#19338,27.);
#3638=CIRCLE('',#19340,37.6);
#3639=CIRCLE('',#19342,27.);
#3640=CIRCLE('',#19344,37.6);
#3641=CIRCLE('',#19346,27.);
#3642=CIRCLE('',#19348,37.6);
#3643=CIRCLE('',#19350,27.);
#3644=CIRCLE('',#19352,37.6);
#3645=CIRCLE('',#19354,27.);
#3646=CIRCLE('',#19356,9.2);
#3647=CIRCLE('',#19357,9.2);
#3648=CIRCLE('',#19358,37.6);
#3649=CIRCLE('',#19360,27.);
#3650=CIRCLE('',#19364,8.7);
#3651=CIRCLE('',#19366,8.7);
#4119=B_SPLINE_CURVE_WITH_KNOTS('',3,(#47356,#47357,#47358,#47359,#47360,
#47361,#47362,#47363,#47364,#47365,#47366,#47367,#47368,#47369,#47370,#47371,
#47372,#47373,#47374),.UNSPECIFIED.,.F.,.F.,(4,3,3,3,3,3,4),(-1.95549230332054,
-1.75875950758926,-1.34349617171388,-1.06103160839237,-0.696688766685516,
-0.248712120243735,0.),.UNSPECIFIED.);
#4120=B_SPLINE_CURVE_WITH_KNOTS('',3,(#47378,#47379,#47380,#47381,#47382,
#47383,#47384,#47385,#47386,#47387,#47388,#47389,#47390,#47391),
 .UNSPECIFIED.,.F.,.F.,(4,2,2,2,2,2,4),(-1.99248695526351,-1.80900909844286,
-1.62729798971959,-1.17075046205492,-0.668721558370408,-0.361288435792572,
-0.0338550864812443),.UNSPECIFIED.);
#4121=B_SPLINE_CURVE_WITH_KNOTS('',3,(#47393,#47394,#47395,#47396),
 .UNSPECIFIED.,.F.,.F.,(4,4),(-0.777523289324711,-0.553838937397288),
 .UNSPECIFIED.);
#4122=B_SPLINE_CURVE_WITH_KNOTS('',3,(#47398,#47399,#47400,#47401,#47402,
#47403,#47404,#47405,#47406,#47407,#47408,#47409,#47410,#47411,#47412,#47413,
#47414,#47415,#47416,#47417,#47418,#47419,#47420,#47421,#47422,#47423,#47424,
#47425),.UNSPECIFIED.,.F.,.F.,(4,3,3,3,3,3,3,3,3,4),(-4.29295029284639,
-3.67766994703909,-2.9703163241262,-2.3742471528823,-2.00020115326112,-1.70071199906103,
-1.1320234547883,-0.387157778255963,-0.249187079614097,0.),
 .UNSPECIFIED.);
#4123=B_SPLINE_CURVE_WITH_KNOTS('',3,(#47428,#47429,#47430,#47431,#47432,
#47433,#47434,#47435,#47436,#47437,#47438,#47439,#47440,#47441,#47442,#47443,
#47444,#47445,#47446,#47447,#47448,#47449,#47450,#47451,#47452,#47453,#47454,
#47455,#47456,#47457,#47458,#47459,#47460,#47461,#47462,#47463,#47464,#47465,
#47466,#47467,#47468,#47469,#47470,#47471,#47472,#47473,#47474,#47475,#47476,
#47477,#47478,#47479),.UNSPECIFIED.,.F.,.F.,(4,3,3,3,3,3,3,3,3,3,3,3,3,
3,3,3,3,4),(-7.1293628449372,-6.73503958122377,-5.85541918839373,-5.49840246457414,
-4.52430913123556,-4.07614123330263,-3.82946470849973,-3.04197748945298,
-2.81695323321067,-2.4773465147895,-2.09725773417371,-1.9043847028781,-1.69190045714872,
-1.20885650102308,-0.931359575039856,-0.504800480040873,-0.274181197077094,
-0.172427513903814),.UNSPECIFIED.);
#4124=B_SPLINE_CURVE_WITH_KNOTS('',3,(#47483,#47484,#47485,#47486),
 .UNSPECIFIED.,.F.,.F.,(4,4),(-0.083488010518486,0.),.UNSPECIFIED.);
#4125=B_SPLINE_CURVE_WITH_KNOTS('',3,(#47490,#47491,#47492,#47493),
 .UNSPECIFIED.,.F.,.F.,(4,4),(-0.0834879590262616,0.),.UNSPECIFIED.);
#4126=B_SPLINE_CURVE_WITH_KNOTS('',3,(#47497,#47498,#47499,#47500),
 .UNSPECIFIED.,.F.,.F.,(4,4),(0.13198468181481,0.18198468181481),
 .UNSPECIFIED.);
#4127=B_SPLINE_CURVE_WITH_KNOTS('',3,(#47502,#47503,#47504,#47505),
 .UNSPECIFIED.,.F.,.F.,(4,4),(0.232761481296011,0.241956189842182),
 .UNSPECIFIED.);
#4128=B_SPLINE_CURVE_WITH_KNOTS('',3,(#47507,#47508,#47509,#47510,#47511,
#47512),.UNSPECIFIED.,.F.,.F.,(4,2,4),(-0.358152343845461,-0.17793853757118,
0.),.UNSPECIFIED.);
#4129=B_SPLINE_CURVE_WITH_KNOTS('',3,(#47516,#47517,#47518,#47519,#47520,
#47521),.UNSPECIFIED.,.F.,.F.,(4,2,4),(-0.346939061794772,-0.172188193249223,
0.),.UNSPECIFIED.);
#4130=B_SPLINE_CURVE_WITH_KNOTS('',3,(#47523,#47524,#47525,#47526),
 .UNSPECIFIED.,.F.,.F.,(4,4),(0.13198468181481,0.18198468181481),
 .UNSPECIFIED.);
#4131=B_SPLINE_CURVE_WITH_KNOTS('',3,(#47530,#47531,#47532,#47533),
 .UNSPECIFIED.,.F.,.F.,(4,4),(0.359141024466699,0.413101541919944),
 .UNSPECIFIED.);
#4132=B_SPLINE_CURVE_WITH_KNOTS('',3,(#47535,#47536,#47537,#47538,#47539,
#47540),.UNSPECIFIED.,.F.,.F.,(4,2,4),(-0.358152325449159,-0.177938418239515,
0.),.UNSPECIFIED.);
#4133=B_SPLINE_CURVE_WITH_KNOTS('',3,(#47544,#47545,#47546,#47547,#47548,
#47549),.UNSPECIFIED.,.F.,.F.,(4,2,4),(-0.346939061574871,-0.172188198132723,
0.),.UNSPECIFIED.);
#4134=B_SPLINE_CURVE_WITH_KNOTS('',3,(#47551,#47552,#47553,#47554),
 .UNSPECIFIED.,.F.,.F.,(4,4),(0.13198468181481,0.181984681814809),
 .UNSPECIFIED.);
#4135=B_SPLINE_CURVE_WITH_KNOTS('',3,(#47558,#47559,#47560,#47561),
 .UNSPECIFIED.,.F.,.F.,(4,4),(0.35914082376606,0.413101294181168),
 .UNSPECIFIED.);
#4136=B_SPLINE_CURVE_WITH_KNOTS('',3,(#47563,#47564,#47565,#47566,#47567,
#47568),.UNSPECIFIED.,.F.,.F.,(4,2,4),(-0.358152343845461,-0.17793853757118,
0.),.UNSPECIFIED.);
#4137=B_SPLINE_CURVE_WITH_KNOTS('',3,(#47572,#47573,#47574,#47575,#47576,
#47577),.UNSPECIFIED.,.F.,.F.,(4,2,4),(-0.346939061794772,-0.172188193249223,
0.),.UNSPECIFIED.);
#4138=B_SPLINE_CURVE_WITH_KNOTS('',3,(#47579,#47580,#47581,#47582),
 .UNSPECIFIED.,.F.,.F.,(4,4),(0.131984681814809,0.181984681814809),
 .UNSPECIFIED.);
#4139=B_SPLINE_CURVE_WITH_KNOTS('',3,(#47586,#47587,#47588,#47589),
 .UNSPECIFIED.,.F.,.F.,(4,4),(0.359141033252547,0.41310155276493),
 .UNSPECIFIED.);
#4140=B_SPLINE_CURVE_WITH_KNOTS('',3,(#47591,#47592,#47593,#47594,#47595,
#47596),.UNSPECIFIED.,.F.,.F.,(4,2,4),(-0.358152325449159,-0.177938418239515,
0.),.UNSPECIFIED.);
#4141=B_SPLINE_CURVE_WITH_KNOTS('',3,(#47600,#47601,#47602,#47603,#47604,
#47605),.UNSPECIFIED.,.F.,.F.,(4,2,4),(-0.346939061574871,-0.172188198132723,
0.),.UNSPECIFIED.);
#4142=B_SPLINE_CURVE_WITH_KNOTS('',3,(#47607,#47608,#47609,#47610),
 .UNSPECIFIED.,.F.,.F.,(4,4),(0.131984681814811,0.18198468181481),
 .UNSPECIFIED.);
#4143=B_SPLINE_CURVE_WITH_KNOTS('',3,(#47614,#47615,#47616,#47617),
 .UNSPECIFIED.,.F.,.F.,(4,4),(0.359140820403378,0.413101290030381),
 .UNSPECIFIED.);
#4144=B_SPLINE_CURVE_WITH_KNOTS('',3,(#47619,#47620,#47621,#47622,#47623,
#47624),.UNSPECIFIED.,.F.,.F.,(4,2,4),(-0.358152343845461,-0.17793853757118,
0.),.UNSPECIFIED.);
#4145=B_SPLINE_CURVE_WITH_KNOTS('',3,(#47628,#47629,#47630,#47631,#47632,
#47633),.UNSPECIFIED.,.F.,.F.,(4,2,4),(-0.346939061794772,-0.172188193249223,
0.),.UNSPECIFIED.);
#4146=B_SPLINE_CURVE_WITH_KNOTS('',3,(#47635,#47636,#47637,#47638),
 .UNSPECIFIED.,.F.,.F.,(4,4),(0.131984681814811,0.181984681814811),
 .UNSPECIFIED.);
#4147=B_SPLINE_CURVE_WITH_KNOTS('',3,(#47642,#47643,#47644,#47645),
 .UNSPECIFIED.,.F.,.F.,(4,4),(0.359141030289299,0.413101549107184),
 .UNSPECIFIED.);
#4148=B_SPLINE_CURVE_WITH_KNOTS('',3,(#47647,#47648,#47649,#47650,#47651,
#47652),.UNSPECIFIED.,.F.,.F.,(4,2,4),(-0.358152325449159,-0.177938418239515,
0.),.UNSPECIFIED.);
#4149=B_SPLINE_CURVE_WITH_KNOTS('',3,(#47656,#47657,#47658,#47659,#47660,
#47661),.UNSPECIFIED.,.F.,.F.,(4,2,4),(-0.346939061574871,-0.172188198132723,
0.),.UNSPECIFIED.);
#4150=B_SPLINE_CURVE_WITH_KNOTS('',3,(#47663,#47664,#47665,#47666),
 .UNSPECIFIED.,.F.,.F.,(4,4),(0.131984681814809,0.181984681814809),
 .UNSPECIFIED.);
#4151=B_SPLINE_CURVE_WITH_KNOTS('',3,(#47670,#47671,#47672,#47673),
 .UNSPECIFIED.,.F.,.F.,(4,4),(0.359140824117849,0.413101294615407),
 .UNSPECIFIED.);
#4152=B_SPLINE_CURVE_WITH_KNOTS('',3,(#47675,#47676,#47677,#47678,#47679,
#47680),.UNSPECIFIED.,.F.,.F.,(4,2,4),(-0.358152343845461,-0.17793853757118,
0.),.UNSPECIFIED.);
#4153=B_SPLINE_CURVE_WITH_KNOTS('',3,(#47689,#47690,#47691,#47692,#47693,
#47694),.UNSPECIFIED.,.F.,.F.,(4,2,4),(-0.346939061794772,-0.172188193249223,
0.),.UNSPECIFIED.);
#4154=B_SPLINE_CURVE_WITH_KNOTS('',3,(#47696,#47697,#47698,#47699),
 .UNSPECIFIED.,.F.,.F.,(4,4),(0.13198468181481,0.18198468181481),
 .UNSPECIFIED.);
#4155=B_SPLINE_CURVE_WITH_KNOTS('',3,(#47703,#47704,#47705,#47706),
 .UNSPECIFIED.,.F.,.F.,(4,4),(0.359141030289304,0.413101549107192),
 .UNSPECIFIED.);
#4156=B_SPLINE_CURVE_WITH_KNOTS('',3,(#47708,#47709,#47710,#47711,#47712,
#47713),.UNSPECIFIED.,.F.,.F.,(4,2,4),(-0.358152325449159,-0.177938418239515,
0.),.UNSPECIFIED.);
#4157=B_SPLINE_CURVE_WITH_KNOTS('',3,(#47717,#47718,#47719,#47720,#47721,
#47722),.UNSPECIFIED.,.F.,.F.,(4,2,4),(-0.346939061574871,-0.172188198132723,
0.),.UNSPECIFIED.);
#4158=B_SPLINE_CURVE_WITH_KNOTS('',3,(#47724,#47725,#47726,#47727),
 .UNSPECIFIED.,.F.,.F.,(4,4),(0.131984681814811,0.18198468181481),
 .UNSPECIFIED.);
#4159=B_SPLINE_CURVE_WITH_KNOTS('',3,(#47731,#47732,#47733,#47734),
 .UNSPECIFIED.,.F.,.F.,(4,4),(0.359140820403392,0.413101290030397),
 .UNSPECIFIED.);
#4160=B_SPLINE_CURVE_WITH_KNOTS('',3,(#47736,#47737,#47738,#47739,#47740,
#47741),.UNSPECIFIED.,.F.,.F.,(4,2,4),(-0.358152343845461,-0.17793853757118,
0.),.UNSPECIFIED.);
#4161=B_SPLINE_CURVE_WITH_KNOTS('',3,(#47745,#47746,#47747,#47748,#47749,
#47750),.UNSPECIFIED.,.F.,.F.,(4,2,4),(-0.346939061794772,-0.172188193249223,
0.),.UNSPECIFIED.);
#4162=B_SPLINE_CURVE_WITH_KNOTS('',3,(#47752,#47753,#47754,#47755),
 .UNSPECIFIED.,.F.,.F.,(4,4),(0.13198468181481,0.18198468181481),
 .UNSPECIFIED.);
#4163=B_SPLINE_CURVE_WITH_KNOTS('',3,(#47759,#47760,#47761,#47762),
 .UNSPECIFIED.,.F.,.F.,(4,4),(0.359141033252549,0.413101552764933),
 .UNSPECIFIED.);
#4164=B_SPLINE_CURVE_WITH_KNOTS('',3,(#47764,#47765,#47766,#47767,#47768,
#47769),.UNSPECIFIED.,.F.,.F.,(4,2,4),(-0.358152325449159,-0.177938418239515,
0.),.UNSPECIFIED.);
#4165=B_SPLINE_CURVE_WITH_KNOTS('',3,(#47773,#47774,#47775,#47776,#47777,
#47778),.UNSPECIFIED.,.F.,.F.,(4,2,4),(-0.346939061574871,-0.172188198132723,
0.),.UNSPECIFIED.);
#4166=B_SPLINE_CURVE_WITH_KNOTS('',3,(#47780,#47781,#47782,#47783),
 .UNSPECIFIED.,.F.,.F.,(4,4),(0.13198468181481,0.181984681814809),
 .UNSPECIFIED.);
#4167=B_SPLINE_CURVE_WITH_KNOTS('',3,(#47787,#47788,#47789,#47790),
 .UNSPECIFIED.,.F.,.F.,(4,4),(0.359140823766061,0.413101294181171),
 .UNSPECIFIED.);
#4168=B_SPLINE_CURVE_WITH_KNOTS('',3,(#47792,#47793,#47794,#47795,#47796,
#47797),.UNSPECIFIED.,.F.,.F.,(4,2,4),(-0.358152343845461,-0.17793853757118,
0.),.UNSPECIFIED.);
#4169=B_SPLINE_CURVE_WITH_KNOTS('',3,(#47801,#47802,#47803,#47804,#47805,
#47806),.UNSPECIFIED.,.F.,.F.,(4,2,4),(-0.346939061794772,-0.172188193249223,
0.),.UNSPECIFIED.);
#4170=B_SPLINE_CURVE_WITH_KNOTS('',3,(#47808,#47809,#47810,#47811),
 .UNSPECIFIED.,.F.,.F.,(4,4),(0.131984681814811,0.18198468181481),
 .UNSPECIFIED.);
#4171=B_SPLINE_CURVE_WITH_KNOTS('',3,(#47815,#47816,#47817,#47818),
 .UNSPECIFIED.,.F.,.F.,(4,4),(0.359141024466694,0.413101541919935),
 .UNSPECIFIED.);
#4172=B_SPLINE_CURVE_WITH_KNOTS('',3,(#47820,#47821,#47822,#47823,#47824,
#47825),.UNSPECIFIED.,.F.,.F.,(4,2,4),(-0.358152325449159,-0.177938418239515,
0.),.UNSPECIFIED.);
#4173=B_SPLINE_CURVE_WITH_KNOTS('',3,(#47829,#47830,#47831,#47832,#47833,
#47834),.UNSPECIFIED.,.F.,.F.,(4,2,4),(-0.346939061574871,-0.172188198132723,
0.),.UNSPECIFIED.);
#4174=B_SPLINE_CURVE_WITH_KNOTS('',3,(#47836,#47837,#47838,#47839),
 .UNSPECIFIED.,.F.,.F.,(4,4),(0.13198468181481,0.18198468181481),
 .UNSPECIFIED.);
#4175=B_SPLINE_CURVE_WITH_KNOTS('',3,(#47843,#47844,#47845,#47846),
 .UNSPECIFIED.,.F.,.F.,(4,4),(0.359140822627922,0.413101292776284),
 .UNSPECIFIED.);
#4176=B_SPLINE_CURVE_WITH_KNOTS('',3,(#47848,#47849,#47850,#47851,#47852,
#47853),.UNSPECIFIED.,.F.,.F.,(4,2,4),(-0.358152343845461,-0.17793853757118,
0.),.UNSPECIFIED.);
#4177=B_SPLINE_CURVE_WITH_KNOTS('',3,(#47857,#47858,#47859,#47860,#47861,
#47862),.UNSPECIFIED.,.F.,.F.,(4,2,4),(-0.346939061794772,-0.172188193249223,
0.),.UNSPECIFIED.);
#4178=B_SPLINE_CURVE_WITH_KNOTS('',3,(#47864,#47865,#47866,#47867),
 .UNSPECIFIED.,.F.,.F.,(4,4),(0.13198468181481,0.18198468181481),
 .UNSPECIFIED.);
#4179=B_SPLINE_CURVE_WITH_KNOTS('',3,(#47871,#47872,#47873,#47874),
 .UNSPECIFIED.,.F.,.F.,(4,4),(0.359141034166343,0.413101553892894),
 .UNSPECIFIED.);
#4180=B_SPLINE_CURVE_WITH_KNOTS('',3,(#47876,#47877,#47878,#47879,#47880,
#47881),.UNSPECIFIED.,.F.,.F.,(4,2,4),(-0.358152325449159,-0.177938418239515,
0.),.UNSPECIFIED.);
#4181=B_SPLINE_CURVE_WITH_KNOTS('',3,(#47884,#47885,#47886,#47887,#47888,
#47889),.UNSPECIFIED.,.F.,.F.,(4,2,4),(-0.346939061574871,-0.172188198132723,
0.),.UNSPECIFIED.);
#4182=B_SPLINE_CURVE_WITH_KNOTS('',3,(#47892,#47893,#47894,#47895),
 .UNSPECIFIED.,.F.,.F.,(4,4),(-0.0834880103557405,0.),.UNSPECIFIED.);
#4183=B_SPLINE_CURVE_WITH_KNOTS('',3,(#47897,#47898,#47899,#47900),
 .UNSPECIFIED.,.F.,.F.,(4,4),(-0.083487959129736,0.),.UNSPECIFIED.);
#4184=B_SPLINE_CURVE_WITH_KNOTS('',3,(#47904,#47905,#47906,#47907),
 .UNSPECIFIED.,.F.,.F.,(4,4),(-0.0834880111905181,0.),.UNSPECIFIED.);
#4185=B_SPLINE_CURVE_WITH_KNOTS('',3,(#47909,#47910,#47911,#47912),
 .UNSPECIFIED.,.F.,.F.,(4,4),(-0.0834879604909712,0.),.UNSPECIFIED.);
#4186=B_SPLINE_CURVE_WITH_KNOTS('',3,(#47916,#47917,#47918,#47919),
 .UNSPECIFIED.,.F.,.F.,(4,4),(-0.0834880110227881,0.),.UNSPECIFIED.);
#4187=B_SPLINE_CURVE_WITH_KNOTS('',3,(#47921,#47922,#47923,#47924),
 .UNSPECIFIED.,.F.,.F.,(4,4),(-0.0834879596098838,0.),.UNSPECIFIED.);
#4188=B_SPLINE_CURVE_WITH_KNOTS('',3,(#47928,#47929,#47930,#47931),
 .UNSPECIFIED.,.F.,.F.,(4,4),(-0.0834880104037423,0.),.UNSPECIFIED.);
#4189=B_SPLINE_CURVE_WITH_KNOTS('',3,(#47933,#47934,#47935,#47936),
 .UNSPECIFIED.,.F.,.F.,(4,4),(-0.083487958469891,0.),.UNSPECIFIED.);
#4190=B_SPLINE_CURVE_WITH_KNOTS('',3,(#47940,#47941,#47942,#47943),
 .UNSPECIFIED.,.F.,.F.,(4,4),(-0.0834880117617837,0.),.UNSPECIFIED.);
#4191=B_SPLINE_CURVE_WITH_KNOTS('',3,(#47945,#47946,#47947,#47948),
 .UNSPECIFIED.,.F.,.F.,(4,4),(-0.0834879580772816,0.),.UNSPECIFIED.);
#4192=B_SPLINE_CURVE_WITH_KNOTS('',3,(#47952,#47953,#47954,#47955),
 .UNSPECIFIED.,.F.,.F.,(4,4),(-0.0834880120026571,0.),.UNSPECIFIED.);
#4193=B_SPLINE_CURVE_WITH_KNOTS('',3,(#47957,#47958,#47959,#47960),
 .UNSPECIFIED.,.F.,.F.,(4,4),(-0.0834879591399868,0.),.UNSPECIFIED.);
#4194=B_SPLINE_CURVE_WITH_KNOTS('',3,(#47964,#47965,#47966,#47967),
 .UNSPECIFIED.,.F.,.F.,(4,4),(-0.0834880112339728,0.),.UNSPECIFIED.);
#4195=B_SPLINE_CURVE_WITH_KNOTS('',3,(#47969,#47970,#47971,#47972),
 .UNSPECIFIED.,.F.,.F.,(4,4),(-0.0834879586604845,0.),.UNSPECIFIED.);
#4196=B_SPLINE_CURVE_WITH_KNOTS('',3,(#47976,#47977,#47978,#47979),
 .UNSPECIFIED.,.F.,.F.,(4,4),(-0.0834880108880153,0.),.UNSPECIFIED.);
#4197=B_SPLINE_CURVE_WITH_KNOTS('',3,(#47981,#47982,#47983,#47984),
 .UNSPECIFIED.,.F.,.F.,(4,4),(-0.083487960114269,0.),.UNSPECIFIED.);
#4198=B_SPLINE_CURVE_WITH_KNOTS('',3,(#47988,#47989,#47990,#47991),
 .UNSPECIFIED.,.F.,.F.,(4,4),(-0.0834880111006107,0.),.UNSPECIFIED.);
#4199=B_SPLINE_CURVE_WITH_KNOTS('',3,(#47993,#47994,#47995,#47996),
 .UNSPECIFIED.,.F.,.F.,(4,4),(-0.0834879593252191,0.),.UNSPECIFIED.);
#4200=B_SPLINE_CURVE_WITH_KNOTS('',3,(#48000,#48001,#48002,#48003),
 .UNSPECIFIED.,.F.,.F.,(4,4),(-0.0834880109980362,0.),.UNSPECIFIED.);
#4201=B_SPLINE_CURVE_WITH_KNOTS('',3,(#48005,#48006,#48007,#48008),
 .UNSPECIFIED.,.F.,.F.,(4,4),(-0.0834879591189384,0.),.UNSPECIFIED.);
#4202=B_SPLINE_CURVE_WITH_KNOTS('',3,(#48012,#48013,#48014,#48015),
 .UNSPECIFIED.,.F.,.F.,(4,4),(-0.0834880113860417,0.),.UNSPECIFIED.);
#4203=B_SPLINE_CURVE_WITH_KNOTS('',3,(#48017,#48018,#48019,#48020),
 .UNSPECIFIED.,.F.,.F.,(4,4),(-0.0834879599185004,0.),.UNSPECIFIED.);
#4204=B_SPLINE_CURVE_WITH_KNOTS('',3,(#48024,#48025,#48026,#48027),
 .UNSPECIFIED.,.F.,.F.,(4,4),(-0.0834880117067383,0.),.UNSPECIFIED.);
#4205=B_SPLINE_CURVE_WITH_KNOTS('',3,(#48029,#48030,#48031,#48032),
 .UNSPECIFIED.,.F.,.F.,(4,4),(-0.0834879582890902,0.),.UNSPECIFIED.);
#4206=B_SPLINE_CURVE_WITH_KNOTS('',3,(#48036,#48037,#48038,#48039),
 .UNSPECIFIED.,.F.,.F.,(4,4),(-0.0834880121469109,0.),.UNSPECIFIED.);
#4207=B_SPLINE_CURVE_WITH_KNOTS('',3,(#48041,#48042,#48043,#48044),
 .UNSPECIFIED.,.F.,.F.,(4,4),(-0.0834879588321369,0.),.UNSPECIFIED.);
#4208=B_SPLINE_CURVE_WITH_KNOTS('',3,(#48179,#48180,#48181,#48182),
 .UNSPECIFIED.,.F.,.F.,(4,4),(19.6867712077087,23.2012226018398),
 .UNSPECIFIED.);
#4209=B_SPLINE_CURVE_WITH_KNOTS('',3,(#48184,#48185,#48186,#48187,#48188,
#48189,#48190,#48191,#48192,#48193,#48194,#48195,#48196,#48197,#48198,#48199,
#48200,#48201,#48202,#48203,#48204,#48205,#48206,#48207,#48208,#48209,#48210,
#48211),.UNSPECIFIED.,.F.,.F.,(4,3,3,3,3,3,3,3,3,4),(-4.29295029280653,
-3.67766994701249,-2.97031632412777,-2.37424715288027,-2.00020115318578,
-1.70071199888906,-1.13202345479137,-0.387157778243597,-0.249187079614106,
0.),.UNSPECIFIED.);
#4210=B_SPLINE_CURVE_WITH_KNOTS('',3,(#48213,#48214,#48215,#48216),
 .UNSPECIFIED.,.F.,.F.,(4,4),(-2.25355902969558,-0.8318795023757),
 .UNSPECIFIED.);
#4211=B_SPLINE_CURVE_WITH_KNOTS('',3,(#48217,#48218,#48219,#48220,#48221,
#48222,#48223,#48224,#48225,#48226,#48227,#48228,#48229,#48230,#48231,#48232,
#48233,#48234,#48235,#48236,#48237,#48238,#48239,#48240,#48241,#48242,#48243,
#48244),.UNSPECIFIED.,.F.,.F.,(4,3,3,3,3,3,3,3,3,4),(0.,0.198329530181083,
0.718473337675007,0.921591739443192,1.13394541355614,1.63848434558204,1.82278760043539,
1.95589943946294,2.14302327760794,2.31810070175045),.UNSPECIFIED.);
#4212=B_SPLINE_CURVE_WITH_KNOTS('',3,(#48247,#48248,#48249,#48250),
 .UNSPECIFIED.,.F.,.F.,(4,4),(-1.48876608190222,-1.26494675411689),
 .UNSPECIFIED.);
#4213=B_SPLINE_CURVE_WITH_KNOTS('',3,(#48252,#48253,#48254,#48255),
 .UNSPECIFIED.,.F.,.F.,(4,4),(-1.29366209142284,-0.119188359258344),
 .UNSPECIFIED.);
#4214=B_SPLINE_CURVE_WITH_KNOTS('',3,(#48392,#48393,#48394,#48395,#48396,
#48397,#48398,#48399,#48400,#48401,#48402,#48403,#48404,#48405,#48406,#48407,
#48408,#48409,#48410,#48411,#48412,#48413),.UNSPECIFIED.,.F.,.F.,(4,3,3,
3,3,3,3,4),(0.,0.569336161400378,0.749177341007451,1.14873589832855,1.30429792490941,
1.39106145779858,1.54578048897719,1.61726052349904),.UNSPECIFIED.);
#4215=B_SPLINE_CURVE_WITH_KNOTS('',3,(#48515,#48516,#48517,#48518,#48519,
#48520,#48521,#48522,#48523,#48524,#48525,#48526,#48527,#48528),
 .UNSPECIFIED.,.F.,.F.,(4,2,2,2,2,2,4),(-1.99248695527052,-1.80900909844907,
-1.62729798972499,-1.17075046205823,-0.668721558372462,-0.361288435792185,
-0.0338550864812489),.UNSPECIFIED.);
#4216=B_SPLINE_CURVE_WITH_KNOTS('',3,(#48529,#48530,#48531,#48532),
 .UNSPECIFIED.,.F.,.F.,(4,4),(0.0499883320126331,0.152208129868745),
 .UNSPECIFIED.);
#4217=B_SPLINE_CURVE_WITH_KNOTS('',3,(#48536,#48537,#48538,#48539),
 .UNSPECIFIED.,.F.,.F.,(4,4),(12.602295500632,15.0893405989718),
 .UNSPECIFIED.);
#4218=B_SPLINE_CURVE_WITH_KNOTS('',3,(#48649,#48650,#48651,#48652),
 .UNSPECIFIED.,.F.,.F.,(4,4),(19.6867712029998,23.2012225962489),
 .UNSPECIFIED.);
#4219=B_SPLINE_CURVE_WITH_KNOTS('',3,(#48654,#48655,#48656,#48657,#48658,
#48659,#48660,#48661,#48662,#48663,#48664,#48665,#48666,#48667,#48668,#48669,
#48670,#48671,#48672,#48673,#48674,#48675,#48676,#48677,#48678,#48679,#48680,
#48681),.UNSPECIFIED.,.F.,.F.,(4,3,3,3,3,3,3,3,3,4),(-4.29295029287552,
-3.67766994705724,-2.97031632412703,-2.37424715288522,-2.00020115328328,
-1.70071199910858,-1.1320234547884,-0.387157778250069,-0.249187079614229,
0.),.UNSPECIFIED.);
#4220=B_SPLINE_CURVE_WITH_KNOTS('',3,(#48683,#48684,#48685,#48686),
 .UNSPECIFIED.,.F.,.F.,(4,4),(-2.25355902969558,-0.8318795023757),
 .UNSPECIFIED.);
#4221=B_SPLINE_CURVE_WITH_KNOTS('',3,(#48687,#48688,#48689,#48690,#48691,
#48692,#48693,#48694,#48695,#48696,#48697,#48698,#48699,#48700,#48701,#48702,
#48703,#48704,#48705,#48706,#48707,#48708,#48709,#48710,#48711,#48712,#48713,
#48714),.UNSPECIFIED.,.F.,.F.,(4,3,3,3,3,3,3,3,3,4),(0.,0.198329530181083,
0.718473337674969,0.921591739443174,1.13394541355614,1.63848434558204,1.82278760043539,
1.95589943946292,2.14302327760794,2.31810070175045),.UNSPECIFIED.);
#4222=B_SPLINE_CURVE_WITH_KNOTS('',3,(#48717,#48718,#48719,#48720),
 .UNSPECIFIED.,.F.,.F.,(4,4),(-0.781276345008619,-0.557585090072962),
 .UNSPECIFIED.);
#4223=B_SPLINE_CURVE_WITH_KNOTS('',3,(#48722,#48723,#48724,#48725),
 .UNSPECIFIED.,.F.,.F.,(4,4),(-1.29366209142284,-0.119188359258344),
 .UNSPECIFIED.);
#4224=B_SPLINE_CURVE_WITH_KNOTS('',3,(#48862,#48863,#48864,#48865,#48866,
#48867,#48868,#48869,#48870,#48871,#48872,#48873,#48874,#48875,#48876,#48877,
#48878,#48879,#48880,#48881,#48882,#48883),.UNSPECIFIED.,.F.,.F.,(4,3,3,
3,3,3,3,4),(0.,0.569336161400378,0.749177341007442,1.14873589832855,1.30429792490947,
1.39106145779861,1.54578048897719,1.61726052349904),.UNSPECIFIED.);
#4225=B_SPLINE_CURVE_WITH_KNOTS('',3,(#48985,#48986,#48987,#48988,#48989,
#48990,#48991,#48992,#48993,#48994,#48995,#48996,#48997,#48998),
 .UNSPECIFIED.,.F.,.F.,(4,2,2,2,2,2,4),(-1.99248695526783,-1.80900909844662,
-1.62729798972286,-1.17075046205687,-0.668721558371707,-0.361288435792094,
-0.0338550864812445),.UNSPECIFIED.);
#4226=B_SPLINE_CURVE_WITH_KNOTS('',3,(#48999,#49000,#49001,#49002),
 .UNSPECIFIED.,.F.,.F.,(4,4),(0.0499883320437557,0.152208130107415),
 .UNSPECIFIED.);
#4227=B_SPLINE_CURVE_WITH_KNOTS('',3,(#49006,#49007,#49008,#49009),
 .UNSPECIFIED.,.F.,.F.,(4,4),(12.6022955008651,15.0893406002079),
 .UNSPECIFIED.);
#4228=B_SPLINE_CURVE_WITH_KNOTS('',3,(#49119,#49120,#49121,#49122),
 .UNSPECIFIED.,.F.,.F.,(4,4),(19.6867712066972,23.2012226007436),
 .UNSPECIFIED.);
#4229=B_SPLINE_CURVE_WITH_KNOTS('',3,(#49124,#49125,#49126,#49127,#49128,
#49129,#49130,#49131,#49132,#49133,#49134,#49135,#49136,#49137,#49138,#49139,
#49140,#49141,#49142,#49143,#49144,#49145,#49146,#49147,#49148,#49149,#49150,
#49151),.UNSPECIFIED.,.F.,.F.,(4,3,3,3,3,3,3,3,3,4),(-4.29295029284741,
-3.67766994703848,-2.97031632412736,-2.37424715288436,-2.00020115322997,
-1.7007119989863,-1.13202345479092,-0.387157778245483,-0.249187079614217,
0.),.UNSPECIFIED.);
#4230=B_SPLINE_CURVE_WITH_KNOTS('',3,(#49153,#49154,#49155,#49156),
 .UNSPECIFIED.,.F.,.F.,(4,4),(-2.25355902969558,-0.8318795023757),
 .UNSPECIFIED.);
#4231=B_SPLINE_CURVE_WITH_KNOTS('',3,(#49157,#49158,#49159,#49160,#49161,
#49162,#49163,#49164,#49165,#49166,#49167,#49168,#49169,#49170,#49171,#49172,
#49173,#49174,#49175,#49176,#49177,#49178,#49179,#49180,#49181,#49182,#49183,
#49184),.UNSPECIFIED.,.F.,.F.,(4,3,3,3,3,3,3,3,3,4),(0.,0.198329530181083,
0.718473337675054,0.921591739443259,1.13394541355614,1.63848434558204,1.82278760043542,
1.95589943946294,2.14302327760794,2.31810070175045),.UNSPECIFIED.);
#4232=B_SPLINE_CURVE_WITH_KNOTS('',3,(#49187,#49188,#49189,#49190),
 .UNSPECIFIED.,.F.,.F.,(4,4),(-1.48004174124428,-1.25625514156074),
 .UNSPECIFIED.);
#4233=B_SPLINE_CURVE_WITH_KNOTS('',3,(#49192,#49193,#49194,#49195),
 .UNSPECIFIED.,.F.,.F.,(4,4),(-1.29366209142284,-0.119188359258344),
 .UNSPECIFIED.);
#4234=B_SPLINE_CURVE_WITH_KNOTS('',3,(#49332,#49333,#49334,#49335,#49336,
#49337,#49338,#49339,#49340,#49341,#49342,#49343,#49344,#49345,#49346,#49347,
#49348,#49349,#49350,#49351,#49352,#49353),.UNSPECIFIED.,.F.,.F.,(4,3,3,
3,3,3,3,4),(0.,0.569336161400378,0.74917734100748,1.14873589832855,1.30429792490946,
1.39106145779859,1.54578048897719,1.61726052349904),.UNSPECIFIED.);
#4235=B_SPLINE_CURVE_WITH_KNOTS('',3,(#49455,#49456,#49457,#49458,#49459,
#49460,#49461,#49462,#49463,#49464,#49465,#49466,#49467,#49468),
 .UNSPECIFIED.,.F.,.F.,(4,2,2,2,2,2,4),(-1.99248695526,-1.80900909843983,
-1.62729798971706,-1.1707504620537,-0.668721558369746,-0.361288435792709,
-0.0338550864812414),.UNSPECIFIED.);
#4236=B_SPLINE_CURVE_WITH_KNOTS('',3,(#49469,#49470,#49471,#49472),
 .UNSPECIFIED.,.F.,.F.,(4,4),(0.0499883320353046,0.152208130042536),
 .UNSPECIFIED.);
#4237=B_SPLINE_CURVE_WITH_KNOTS('',3,(#49476,#49477,#49478,#49479),
 .UNSPECIFIED.,.F.,.F.,(4,4),(12.6022955009377,15.0893406005466),
 .UNSPECIFIED.);
#4238=B_SPLINE_CURVE_WITH_KNOTS('',3,(#49589,#49590,#49591,#49592),
 .UNSPECIFIED.,.F.,.F.,(4,4),(19.6867712047202,23.201222598638),
 .UNSPECIFIED.);
#4239=B_SPLINE_CURVE_WITH_KNOTS('',3,(#49594,#49595,#49596,#49597,#49598,
#49599,#49600,#49601,#49602,#49603,#49604,#49605,#49606,#49607,#49608,#49609,
#49610,#49611,#49612,#49613,#49614,#49615,#49616,#49617,#49618,#49619,#49620,
#49621),.UNSPECIFIED.,.F.,.F.,(4,3,3,3,3,3,3,3,3,4),(-4.29295029281412,
-3.677669947019,-2.9703163241297,-2.37424715288221,-2.00020115321966,-1.70071199896483,
-1.13202345479064,-0.387157778248161,-0.249187079614164,0.),
 .UNSPECIFIED.);
#4240=B_SPLINE_CURVE_WITH_KNOTS('',3,(#49623,#49624,#49625,#49626),
 .UNSPECIFIED.,.F.,.F.,(4,4),(-2.25355902969558,-0.8318795023757),
 .UNSPECIFIED.);
#4241=B_SPLINE_CURVE_WITH_KNOTS('',3,(#49627,#49628,#49629,#49630,#49631,
#49632,#49633,#49634,#49635,#49636,#49637,#49638,#49639,#49640,#49641,#49642,
#49643,#49644,#49645,#49646,#49647,#49648,#49649,#49650,#49651,#49652,#49653,
#49654),.UNSPECIFIED.,.F.,.F.,(4,3,3,3,3,3,3,3,3,4),(0.,0.198329530181083,
0.718473337675014,0.921591739443205,1.13394541355614,1.63848434558204,1.8227876004354,
1.95589943946296,2.14302327760794,2.31810070175045),.UNSPECIFIED.);
#4242=B_SPLINE_CURVE_WITH_KNOTS('',3,(#49657,#49658,#49659,#49660,#49661,
#49662),.UNSPECIFIED.,.F.,.F.,(4,2,4),(-1.24678830233717,-1.23436729644851,
-1.02314392866673),.UNSPECIFIED.);
#4243=B_SPLINE_CURVE_WITH_KNOTS('',3,(#49664,#49665,#49666,#49667),
 .UNSPECIFIED.,.F.,.F.,(4,4),(-1.29366209142284,-0.119188359258344),
 .UNSPECIFIED.);
#4244=B_SPLINE_CURVE_WITH_KNOTS('',3,(#49804,#49805,#49806,#49807,#49808,
#49809,#49810,#49811,#49812,#49813,#49814,#49815,#49816,#49817,#49818,#49819,
#49820,#49821,#49822,#49823,#49824,#49825),.UNSPECIFIED.,.F.,.F.,(4,3,3,
3,3,3,3,4),(0.,0.569336161400378,0.749177341007471,1.14873589832855,1.30429792490946,
1.39106145779861,1.54578048897719,1.61726052349904),.UNSPECIFIED.);
#4245=B_SPLINE_CURVE_WITH_KNOTS('',3,(#49927,#49928,#49929,#49930,#49931,
#49932,#49933,#49934,#49935,#49936,#49937,#49938,#49939,#49940),
 .UNSPECIFIED.,.F.,.F.,(4,2,2,2,2,2,4),(-1.99248695526232,-1.80900909844183,
-1.62729798971886,-1.17075046205496,-0.668721558369855,-0.361288435792721,
-0.0338550864812465),.UNSPECIFIED.);
#4246=B_SPLINE_CURVE_WITH_KNOTS('',3,(#49941,#49942,#49943,#49944),
 .UNSPECIFIED.,.F.,.F.,(4,4),(0.04998833204185,0.152208130092823),
 .UNSPECIFIED.);
#4247=B_SPLINE_CURVE_WITH_KNOTS('',3,(#49948,#49949,#49950,#49951),
 .UNSPECIFIED.,.F.,.F.,(4,4),(12.6022955007997,15.0893405996947),
 .UNSPECIFIED.);
#4248=B_SPLINE_CURVE_WITH_KNOTS('',3,(#50061,#50062,#50063,#50064),
 .UNSPECIFIED.,.F.,.F.,(4,4),(19.6867712021019,23.2012225955095),
 .UNSPECIFIED.);
#4249=B_SPLINE_CURVE_WITH_KNOTS('',3,(#50066,#50067,#50068,#50069,#50070,
#50071,#50072,#50073,#50074,#50075,#50076,#50077,#50078,#50079,#50080,#50081,
#50082,#50083,#50084,#50085,#50086,#50087,#50088,#50089,#50090,#50091,#50092,
#50093),.UNSPECIFIED.,.F.,.F.,(4,3,3,3,3,3,3,3,3,4),(-4.29295029283852,
-3.67766994703207,-2.97031632412226,-2.37424715288117,-2.00020115324444,
-1.70071199902372,-1.1320234547888,-0.387157778246094,-0.249187079614028,
0.),.UNSPECIFIED.);
#4250=B_SPLINE_CURVE_WITH_KNOTS('',3,(#50095,#50096,#50097,#50098),
 .UNSPECIFIED.,.F.,.F.,(4,4),(-2.25355902969558,-0.8318795023757),
 .UNSPECIFIED.);
#4251=B_SPLINE_CURVE_WITH_KNOTS('',3,(#50099,#50100,#50101,#50102,#50103,
#50104,#50105,#50106,#50107,#50108,#50109,#50110,#50111,#50112,#50113,#50114,
#50115,#50116,#50117,#50118,#50119,#50120,#50121,#50122,#50123,#50124,#50125,
#50126),.UNSPECIFIED.,.F.,.F.,(4,3,3,3,3,3,3,3,3,4),(0.,0.198329530181083,
0.718473337675043,0.921591739443273,1.13394541355614,1.63848434558204,1.8227876004354,
1.95589943946294,2.14302327760794,2.31810070175045),.UNSPECIFIED.);
#4252=B_SPLINE_CURVE_WITH_KNOTS('',3,(#50129,#50130,#50131,#50132,#50133,
#50134),.UNSPECIFIED.,.F.,.F.,(4,2,4),(-1.45143148105007,-1.23436729644851,
-1.22796157678455),.UNSPECIFIED.);
#4253=B_SPLINE_CURVE_WITH_KNOTS('',3,(#50136,#50137,#50138,#50139),
 .UNSPECIFIED.,.F.,.F.,(4,4),(-1.29366209142284,-0.119188359258344),
 .UNSPECIFIED.);
#4254=B_SPLINE_CURVE_WITH_KNOTS('',3,(#50276,#50277,#50278,#50279,#50280,
#50281,#50282,#50283,#50284,#50285,#50286,#50287,#50288,#50289,#50290,#50291,
#50292,#50293,#50294,#50295,#50296,#50297),.UNSPECIFIED.,.F.,.F.,(4,3,3,
3,3,3,3,4),(0.,0.569336161400378,0.749177341007454,1.14873589832855,1.30429792490945,
1.39106145779861,1.54578048897719,1.61726052349904),.UNSPECIFIED.);
#4255=B_SPLINE_CURVE_WITH_KNOTS('',3,(#50399,#50400,#50401,#50402,#50403,
#50404,#50405,#50406,#50407,#50408,#50409,#50410,#50411,#50412),
 .UNSPECIFIED.,.F.,.F.,(4,2,2,2,2,2,4),(-1.99248695526215,-1.80900909844175,
-1.62729798971876,-1.17075046205484,-0.66872155836966,-0.361288435792731,
-0.0338550864812428),.UNSPECIFIED.);
#4256=B_SPLINE_CURVE_WITH_KNOTS('',3,(#50413,#50414,#50415,#50416),
 .UNSPECIFIED.,.F.,.F.,(4,4),(0.0499883320345709,0.152208130037191),
 .UNSPECIFIED.);
#4257=B_SPLINE_CURVE_WITH_KNOTS('',3,(#50420,#50421,#50422,#50423),
 .UNSPECIFIED.,.F.,.F.,(4,4),(12.6022955008531,15.0893406000084),
 .UNSPECIFIED.);
#4258=B_SPLINE_CURVE_WITH_KNOTS('',3,(#50533,#50534,#50535,#50536),
 .UNSPECIFIED.,.F.,.F.,(4,4),(19.6867712068538,23.2012226010116),
 .UNSPECIFIED.);
#4259=B_SPLINE_CURVE_WITH_KNOTS('',3,(#50538,#50539,#50540,#50541,#50542,
#50543,#50544,#50545,#50546,#50547,#50548,#50549,#50550,#50551,#50552,#50553,
#50554,#50555,#50556,#50557,#50558,#50559,#50560,#50561,#50562,#50563,#50564,
#50565),.UNSPECIFIED.,.F.,.F.,(4,3,3,3,3,3,3,3,3,4),(-4.29295029283119,
-3.67766994702957,-2.97031632412832,-2.37424715288224,-2.00020115323496,
-1.70071199900048,-1.13202345478954,-0.38715777824571,-0.249187079614159,
0.),.UNSPECIFIED.);
#4260=B_SPLINE_CURVE_WITH_KNOTS('',3,(#50567,#50568,#50569,#50570),
 .UNSPECIFIED.,.F.,.F.,(4,4),(-2.25355902969558,-0.8318795023757),
 .UNSPECIFIED.);
#4261=B_SPLINE_CURVE_WITH_KNOTS('',3,(#50571,#50572,#50573,#50574,#50575,
#50576,#50577,#50578,#50579,#50580,#50581,#50582,#50583,#50584,#50585,#50586,
#50587,#50588,#50589,#50590,#50591,#50592,#50593,#50594,#50595,#50596,#50597,
#50598),.UNSPECIFIED.,.F.,.F.,(4,3,3,3,3,3,3,3,3,4),(0.,0.198329530181083,
0.718473337675035,0.921591739443244,1.13394541355614,1.63848434558204,1.82278760043539,
1.95589943946293,2.14302327760794,2.31810070175045),.UNSPECIFIED.);
#4262=B_SPLINE_CURVE_WITH_KNOTS('',3,(#50601,#50602,#50603,#50604),
 .UNSPECIFIED.,.F.,.F.,(4,4),(-1.47623053088356,-1.25245876190875),
 .UNSPECIFIED.);
#4263=B_SPLINE_CURVE_WITH_KNOTS('',3,(#50606,#50607,#50608,#50609),
 .UNSPECIFIED.,.F.,.F.,(4,4),(-1.29366209142284,-0.119188359258344),
 .UNSPECIFIED.);
#4264=B_SPLINE_CURVE_WITH_KNOTS('',3,(#50746,#50747,#50748,#50749,#50750,
#50751,#50752,#50753,#50754,#50755,#50756,#50757,#50758,#50759,#50760,#50761,
#50762,#50763,#50764,#50765,#50766,#50767),.UNSPECIFIED.,.F.,.F.,(4,3,3,
3,3,3,3,4),(0.,0.569336161400378,0.749177341007436,1.14873589832855,1.30429792490944,
1.39106145779861,1.54578048897719,1.61726052349904),.UNSPECIFIED.);
#4265=B_SPLINE_CURVE_WITH_KNOTS('',3,(#50869,#50870,#50871,#50872,#50873,
#50874,#50875,#50876,#50877,#50878,#50879,#50880,#50881,#50882),
 .UNSPECIFIED.,.F.,.F.,(4,2,2,2,2,2,4),(-1.9924869552618,-1.80900909844148,
-1.62729798971846,-1.17075046205436,-0.668721558370139,-0.361288435792605,
-0.0338550864812418),.UNSPECIFIED.);
#4266=B_SPLINE_CURVE_WITH_KNOTS('',3,(#50883,#50884,#50885,#50886),
 .UNSPECIFIED.,.F.,.F.,(4,4),(0.0499883320206314,0.152208129929869),
 .UNSPECIFIED.);
#4267=B_SPLINE_CURVE_WITH_KNOTS('',3,(#50890,#50891,#50892,#50893),
 .UNSPECIFIED.,.F.,.F.,(4,4),(12.6022955008471,15.0893406001972),
 .UNSPECIFIED.);
#4268=B_SPLINE_CURVE_WITH_KNOTS('',3,(#51002,#51003,#51004,#51005),
 .UNSPECIFIED.,.F.,.F.,(4,4),(19.6867712032198,23.2012225965881),
 .UNSPECIFIED.);
#4269=B_SPLINE_CURVE_WITH_KNOTS('',3,(#51007,#51008,#51009,#51010),
 .UNSPECIFIED.,.F.,.F.,(4,4),(-2.25355902969558,-0.831879502375701),
 .UNSPECIFIED.);
#4270=B_SPLINE_CURVE_WITH_KNOTS('',3,(#51011,#51012,#51013,#51014,#51015,
#51016,#51017,#51018,#51019,#51020,#51021,#51022,#51023,#51024,#51025,#51026,
#51027,#51028,#51029,#51030,#51031,#51032,#51033,#51034,#51035,#51036,#51037,
#51038),.UNSPECIFIED.,.F.,.F.,(4,3,3,3,3,3,3,3,3,4),(0.,0.198329530181083,
0.718473337675014,0.921591739443195,1.13394541355614,1.63848434558204,1.82278760043539,
1.95589943946293,2.14302327760794,2.31810070175045),.UNSPECIFIED.);
#4271=B_SPLINE_CURVE_WITH_KNOTS('',3,(#51041,#51042,#51043,#51044),
 .UNSPECIFIED.,.F.,.F.,(4,4),(-1.29366209142284,-0.119188359258344),
 .UNSPECIFIED.);
#4272=B_SPLINE_CURVE_WITH_KNOTS('',3,(#51181,#51182,#51183,#51184,#51185,
#51186,#51187,#51188,#51189,#51190,#51191,#51192,#51193,#51194,#51195,#51196,
#51197,#51198,#51199,#51200,#51201,#51202),.UNSPECIFIED.,.F.,.F.,(4,3,3,
3,3,3,3,4),(0.,0.569336161400378,0.749177341007455,1.14873589832855,1.30429792490947,
1.39106145779862,1.54578048897719,1.61726052349904),.UNSPECIFIED.);
#4273=B_SPLINE_CURVE_WITH_KNOTS('',3,(#51303,#51304,#51305,#51306),
 .UNSPECIFIED.,.F.,.F.,(4,4),(0.0499883320316304,0.152208130014649),
 .UNSPECIFIED.);
#4274=B_SPLINE_CURVE_WITH_KNOTS('',3,(#51308,#51309,#51310,#51311),
 .UNSPECIFIED.,.F.,.F.,(4,4),(12.60229550093,15.0893406007716),
 .UNSPECIFIED.);
#4275=B_SPLINE_CURVE_WITH_KNOTS('',3,(#51488,#51489,#51490,#51491,#51492,
#51493,#51494,#51495,#51496,#51497,#51498,#51499,#51500,#51501,#51502,#51503,
#51504,#51505,#51506,#51507,#51508,#51509,#51510,#51511,#51512,#51513,#51514,
#51515,#51516,#51517,#51518,#51519,#51520,#51521,#51522,#51523,#51524,#51525,
#51526,#51527,#51528,#51529,#51530,#51531,#51532,#51533),.UNSPECIFIED.,
 .F.,.F.,(4,3,3,3,3,3,3,3,3,3,3,3,3,3,3,4),(-3.56163244824597,-3.30468798711506,
-3.18832863267718,-3.03317964462045,-2.79853132681797,-2.75550071537558,
-2.52404318191444,-2.41525037355583,-2.16219512366447,-1.94576347076795,
-1.75875950761201,-1.34373914266847,-1.06103160840153,-0.696688766667217,
-0.248712120244377,0.),.UNSPECIFIED.);
#4276=B_SPLINE_CURVE_WITH_KNOTS('',3,(#51535,#51536,#51537,#51538,#51539,
#51540),.UNSPECIFIED.,.F.,.F.,(4,2,4),(-1.81367248236635,-1.45004244433882,
-0.253045058252053),.UNSPECIFIED.);
#4277=B_SPLINE_CURVE_WITH_KNOTS('',3,(#51542,#51543,#51544,#51545,#51546,
#51547,#51548,#51549,#51550,#51551,#51552,#51553),.UNSPECIFIED.,.F.,.F.,
(4,2,2,2,2,4),(1.08484844498112,2.49572829361744,3.80512145389228,4.87611899720136,
6.43508432402471,7.63234746756005),.UNSPECIFIED.);
#4278=B_SPLINE_CURVE_WITH_KNOTS('',3,(#51554,#51555,#51556,#51557,#51558,
#51559),.UNSPECIFIED.,.F.,.F.,(4,2,4),(0.,0.791088048129032,1.08484844498112),
 .UNSPECIFIED.);
#4279=B_SPLINE_CURVE_WITH_KNOTS('',3,(#51562,#51563,#51564,#51565,#51566,
#51567),.UNSPECIFIED.,.F.,.F.,(4,2,4),(-0.46225453508618,-0.379477414403806,
-0.20889105167514),.UNSPECIFIED.);
#4280=B_SPLINE_CURVE_WITH_KNOTS('',3,(#51569,#51570,#51571,#51572),
 .UNSPECIFIED.,.F.,.F.,(4,4),(-3.09523587865368,-0.674081646507512),
 .UNSPECIFIED.);
#4281=B_SPLINE_CURVE_WITH_KNOTS('',3,(#51849,#51850,#51851,#51852,#51853,
#51854,#51855,#51856,#51857,#51858,#51859,#51860,#51861,#51862,#51863,#51864,
#51865,#51866,#51867,#51868,#51869,#51870,#51871,#51872,#51873,#51874,#51875,
#51876,#51877,#51878,#51879,#51880,#51881,#51882,#51883,#51884,#51885,#51886,
#51887,#51888,#51889,#51890,#51891,#51892,#51893,#51894),.UNSPECIFIED.,
 .F.,.F.,(4,3,3,3,3,3,3,3,3,3,3,3,3,3,3,4),(0.,0.929985381254847,1.4414618647496,
1.65956723730638,2.03170963890847,2.3019465940753,2.89554149400049,3.67764692687497,
4.06869964331221,4.3263657455837,4.45975235974945,5.09319960112738,5.36523598622997,
5.53913936027952,5.55541982778557,5.8077795608208),.UNSPECIFIED.);
#4282=B_SPLINE_CURVE_WITH_KNOTS('',3,(#52076,#52077,#52078,#52079,#52080,
#52081,#52082,#52083,#52084,#52085,#52086,#52087,#52088,#52089,#52090,#52091,
#52092,#52093,#52094,#52095,#52096,#52097,#52098,#52099,#52100,#52101,#52102,
#52103,#52104,#52105,#52106,#52107,#52108,#52109,#52110,#52111,#52112,#52113,
#52114,#52115,#52116,#52117,#52118,#52119,#52120,#52121,#52122,#52123,#52124,
#52125,#52126,#52127),.UNSPECIFIED.,.F.,.F.,(4,3,3,3,3,3,3,3,3,3,3,3,3,
3,3,3,3,4),(-7.12936283646632,-6.73503957360069,-5.85541917358046,-5.49840246106417,
-4.52430913776898,-4.07614123026294,-3.82946471505583,-3.0419774933968,
-2.81695323655032,-2.47734651704596,-2.09725773516292,-1.90438470328338,
-1.69190045629947,-1.20885650127841,-0.931359575121362,-0.50480048004898,
-0.268904979593478,-0.0293416084169379),.UNSPECIFIED.);
#4283=B_SPLINE_CURVE_WITH_KNOTS('',3,(#52128,#52129,#52130,#52131),
 .UNSPECIFIED.,.F.,.F.,(4,4),(0.0499738748996539,0.152077174914533),
 .UNSPECIFIED.);
#4284=B_SPLINE_CURVE_WITH_KNOTS('',3,(#52310,#52311,#52312,#52313,#52314,
#52315,#52316,#52317,#52318,#52319,#52320,#52321,#52322,#52323,#52324,#52325,
#52326,#52327,#52328,#52329,#52330,#52331,#52332,#52333,#52334,#52335,#52336,
#52337,#52338,#52339,#52340,#52341,#52342,#52343,#52344,#52345,#52346,#52347,
#52348,#52349,#52350,#52351,#52352,#52353,#52354,#52355),.UNSPECIFIED.,
 .F.,.F.,(4,3,3,3,3,3,3,3,3,3,3,3,3,3,3,4),(-3.56163244787668,-3.3046879868165,
-3.18832863247323,-3.03317964444258,-2.79853132694452,-2.75550071530183,
-2.52404318184636,-2.41525037352192,-2.16219512342656,-1.94576347074032,
-1.75875950758838,-1.34373914265465,-1.06103160839068,-0.696688766680895,
-0.248712120243363,0.),.UNSPECIFIED.);
#4285=B_SPLINE_CURVE_WITH_KNOTS('',3,(#52357,#52358,#52359,#52360,#52361,
#52362),.UNSPECIFIED.,.F.,.F.,(4,2,4),(-1.81367248236635,-1.45004244433882,
-0.253045058252053),.UNSPECIFIED.);
#4286=B_SPLINE_CURVE_WITH_KNOTS('',3,(#52364,#52365,#52366,#52367,#52368,
#52369,#52370,#52371,#52372,#52373,#52374,#52375),.UNSPECIFIED.,.F.,.F.,
(4,2,2,2,2,4),(1.08484844498112,2.49572829361744,3.80512145389228,4.87611899720136,
6.43508432402471,7.63234746756005),.UNSPECIFIED.);
#4287=B_SPLINE_CURVE_WITH_KNOTS('',3,(#52376,#52377,#52378,#52379,#52380,
#52381),.UNSPECIFIED.,.F.,.F.,(4,2,4),(0.,0.791088048129032,1.08484844498112),
 .UNSPECIFIED.);
#4288=B_SPLINE_CURVE_WITH_KNOTS('',3,(#52384,#52385,#52386,#52387,#52388,
#52389),.UNSPECIFIED.,.F.,.F.,(4,2,4),(-0.667329469112299,-0.60653547892591,
-0.414285256061857),.UNSPECIFIED.);
#4289=B_SPLINE_CURVE_WITH_KNOTS('',3,(#52391,#52392,#52393,#52394),
 .UNSPECIFIED.,.F.,.F.,(4,4),(-3.09523587865368,-0.674081646507512),
 .UNSPECIFIED.);
#4290=B_SPLINE_CURVE_WITH_KNOTS('',3,(#52671,#52672,#52673,#52674,#52675,
#52676,#52677,#52678,#52679,#52680,#52681,#52682,#52683,#52684,#52685,#52686,
#52687,#52688,#52689,#52690,#52691,#52692,#52693,#52694,#52695,#52696,#52697,
#52698,#52699,#52700,#52701,#52702,#52703,#52704,#52705,#52706,#52707,#52708,
#52709,#52710,#52711,#52712,#52713,#52714,#52715,#52716),.UNSPECIFIED.,
 .F.,.F.,(4,3,3,3,3,3,3,3,3,3,3,3,3,3,3,4),(0.,0.929985381254847,1.44146186475008,
1.65956723730638,2.03170963890849,2.30194659407527,2.89554149400049,3.67764692687497,
4.06869964331221,4.3263657455837,4.45975235974945,5.09319960112738,5.36523598622995,
5.53913936027952,5.55541982778557,5.8077795608208),.UNSPECIFIED.);
#4291=B_SPLINE_CURVE_WITH_KNOTS('',3,(#52928,#52929,#52930,#52931,#52932,
#52933,#52934,#52935,#52936,#52937,#52938,#52939,#52940,#52941,#52942,#52943,
#52944,#52945,#52946,#52947,#52948,#52949,#52950,#52951,#52952,#52953,#52954,
#52955,#52956,#52957,#52958,#52959,#52960,#52961,#52962,#52963,#52964,#52965,
#52966,#52967,#52968,#52969,#52970,#52971,#52972,#52973,#52974,#52975,#52976,
#52977,#52978,#52979),.UNSPECIFIED.,.F.,.F.,(4,3,3,3,3,3,3,3,3,3,3,3,3,
3,3,3,3,4),(-7.129362849605,-6.73503958541797,-5.85541919680017,-5.49840246643452,
-4.52430912729766,-4.07614123495784,-3.82946470458214,-3.04197748709441,
-2.81695323121577,-2.47734651344292,-2.09725773358231,-1.90438470263432,
-1.69190045765133,-1.20885650086995,-0.931359574991274,-0.50480048003591,
-0.268904979566511,-0.0293416084169345),.UNSPECIFIED.);
#4292=B_SPLINE_CURVE_WITH_KNOTS('',3,(#52980,#52981,#52982,#52983),
 .UNSPECIFIED.,.F.,.F.,(4,4),(0.0499738749072504,0.152077174976504),
 .UNSPECIFIED.);
#4293=B_SPLINE_CURVE_WITH_KNOTS('',3,(#53167,#53168,#53169,#53170,#53171,
#53172,#53173,#53174,#53175,#53176,#53177,#53178,#53179,#53180,#53181,#53182,
#53183,#53184,#53185,#53186,#53187,#53188,#53189,#53190,#53191,#53192,#53193,
#53194,#53195,#53196,#53197,#53198,#53199,#53200,#53201,#53202,#53203,#53204,
#53205,#53206,#53207,#53208,#53209,#53210,#53211,#53212),.UNSPECIFIED.,
 .F.,.F.,(4,3,3,3,3,3,3,3,3,3,3,3,3,3,3,4),(-3.56163244831553,-3.30468798717037,
-3.18832863271292,-3.03317964465101,-2.79853132678738,-2.75550071538447,
-2.52404318192142,-2.41525037355563,-2.16219512370471,-1.94576347077165,
-1.75875950761067,-1.34373914266885,-1.06103160840174,-0.69668876667261,
-0.2487121202443,0.),.UNSPECIFIED.);
#4294=B_SPLINE_CURVE_WITH_KNOTS('',3,(#53214,#53215,#53216,#53217,#53218,
#53219),.UNSPECIFIED.,.F.,.F.,(4,2,4),(-1.81367248236635,-1.45004244433882,
-0.253045058252053),.UNSPECIFIED.);
#4295=B_SPLINE_CURVE_WITH_KNOTS('',3,(#53221,#53222,#53223,#53224,#53225,
#53226,#53227,#53228,#53229,#53230,#53231,#53232),.UNSPECIFIED.,.F.,.F.,
(4,2,2,2,2,4),(1.08484844498112,2.49572829361744,3.80512145389228,4.87611899720136,
6.43508432402471,7.63234746756005),.UNSPECIFIED.);
#4296=B_SPLINE_CURVE_WITH_KNOTS('',3,(#53233,#53234,#53235,#53236,#53237,
#53238),.UNSPECIFIED.,.F.,.F.,(4,2,4),(0.,0.791088048129032,1.08484844498112),
 .UNSPECIFIED.);
#4297=B_SPLINE_CURVE_WITH_KNOTS('',3,(#53241,#53242,#53243,#53244,#53245,
#53246),.UNSPECIFIED.,.F.,.F.,(4,2,4),(-0.477412011610917,-0.379477414403805,
-0.22405790136428),.UNSPECIFIED.);
#4298=B_SPLINE_CURVE_WITH_KNOTS('',3,(#53248,#53249,#53250,#53251),
 .UNSPECIFIED.,.F.,.F.,(4,4),(-3.09523587865368,-0.674081646507512),
 .UNSPECIFIED.);
#4299=B_SPLINE_CURVE_WITH_KNOTS('',3,(#53528,#53529,#53530,#53531,#53532,
#53533,#53534,#53535,#53536,#53537,#53538,#53539,#53540,#53541,#53542,#53543,
#53544,#53545,#53546,#53547,#53548,#53549,#53550,#53551,#53552,#53553,#53554,
#53555,#53556,#53557,#53558,#53559,#53560,#53561,#53562,#53563,#53564,#53565,
#53566,#53567,#53568,#53569,#53570,#53571,#53572,#53573),.UNSPECIFIED.,
 .F.,.F.,(4,3,3,3,3,3,3,3,3,3,3,3,3,3,3,4),(0.,0.929985381254847,1.44146186474994,
1.65956723730638,2.03170963890847,2.3019465940753,2.89554149400049,3.67764692687497,
4.06869964331221,4.3263657455837,4.45975235974945,5.09319960112738,5.36523598623069,
5.53913936027934,5.55541982778557,5.8077795608208),.UNSPECIFIED.);
#4300=B_SPLINE_CURVE_WITH_KNOTS('',3,(#53750,#53751,#53752,#53753,#53754,
#53755,#53756,#53757,#53758,#53759,#53760,#53761,#53762,#53763,#53764,#53765,
#53766,#53767,#53768,#53769,#53770,#53771,#53772,#53773,#53774,#53775,#53776,
#53777,#53778,#53779,#53780,#53781,#53782,#53783,#53784,#53785,#53786,#53787,
#53788,#53789,#53790,#53791,#53792,#53793,#53794,#53795,#53796,#53797,#53798,
#53799,#53800,#53801),.UNSPECIFIED.,.F.,.F.,(4,3,3,3,3,3,3,3,3,3,3,3,3,
3,3,3,3,4),(-7.1293628478505,-6.73503958384616,-5.85541919345525,-5.49840246578807,
-4.52430912902298,-4.07614123434755,-3.82946470627502,-3.04197748811397,
-2.81695323207643,-2.47734651402268,-2.09725773383644,-1.90438470273958,
-1.69190045743555,-1.20885650093581,-0.931359575012167,-0.50480048003812,
-0.268904979571344,-0.0293416084169348),.UNSPECIFIED.);
#4301=B_SPLINE_CURVE_WITH_KNOTS('',3,(#53802,#53803,#53804,#53805),
 .UNSPECIFIED.,.F.,.F.,(4,4),(0.0499738749087634,0.152077174988778),
 .UNSPECIFIED.);
#4302=B_SPLINE_CURVE_WITH_KNOTS('',3,(#53984,#53985,#53986,#53987,#53988,
#53989,#53990,#53991,#53992,#53993,#53994,#53995,#53996,#53997,#53998,#53999,
#54000,#54001,#54002,#54003,#54004,#54005,#54006,#54007,#54008,#54009,#54010,
#54011,#54012,#54013,#54014,#54015,#54016,#54017,#54018,#54019,#54020,#54021,
#54022,#54023,#54024,#54025,#54026,#54027,#54028,#54029),.UNSPECIFIED.,
 .F.,.F.,(4,3,3,3,3,3,3,3,3,3,3,3,3,3,3,4),(-3.56163244846089,-3.30468798728467,
-3.1883286327842,-3.03317964471123,-2.79853132670929,-2.75550071539819,
-2.52404318193367,-2.41525037355264,-2.16219512378884,-1.94576347076806,
-1.75875950760639,-1.34373914266426,-1.06103160839798,-0.696688766664339,
-0.248712120244048,0.),.UNSPECIFIED.);
#4303=B_SPLINE_CURVE_WITH_KNOTS('',3,(#54031,#54032,#54033,#54034,#54035,
#54036),.UNSPECIFIED.,.F.,.F.,(4,2,4),(-1.81367248236635,-1.45004244433882,
-0.253045058252053),.UNSPECIFIED.);
#4304=B_SPLINE_CURVE_WITH_KNOTS('',3,(#54038,#54039,#54040,#54041,#54042,
#54043,#54044,#54045,#54046,#54047,#54048,#54049),.UNSPECIFIED.,.F.,.F.,
(4,2,2,2,2,4),(1.08484844498112,2.49572829361744,3.80512145389228,4.87611899720136,
6.43508432402471,7.63234746756005),.UNSPECIFIED.);
#4305=B_SPLINE_CURVE_WITH_KNOTS('',3,(#54050,#54051,#54052,#54053,#54054,
#54055),.UNSPECIFIED.,.F.,.F.,(4,2,4),(0.,0.791088048129032,1.08484844498112),
 .UNSPECIFIED.);
#4306=B_SPLINE_CURVE_WITH_KNOTS('',3,(#54058,#54059,#54060,#54061,#54062,
#54063),.UNSPECIFIED.,.F.,.F.,(4,2,4),(-0.711364948515675,-0.629369591998026,
-0.458258817348068),.UNSPECIFIED.);
#4307=B_SPLINE_CURVE_WITH_KNOTS('',3,(#54065,#54066,#54067,#54068),
 .UNSPECIFIED.,.F.,.F.,(4,4),(-3.09523587865368,-0.674081646507512),
 .UNSPECIFIED.);
#4308=B_SPLINE_CURVE_WITH_KNOTS('',3,(#54345,#54346,#54347,#54348,#54349,
#54350,#54351,#54352,#54353,#54354,#54355,#54356,#54357,#54358,#54359,#54360,
#54361,#54362,#54363,#54364,#54365,#54366,#54367,#54368,#54369,#54370,#54371,
#54372,#54373,#54374,#54375,#54376,#54377,#54378,#54379,#54380,#54381,#54382,
#54383,#54384,#54385,#54386,#54387,#54388,#54389,#54390),.UNSPECIFIED.,
 .F.,.F.,(4,3,3,3,3,3,3,3,3,3,3,3,3,3,3,4),(0.,0.929985381254847,1.441461864751,
1.65956723730638,2.03170963890802,2.30194659407528,2.89554149400049,3.67764692687497,
4.06869964331221,4.3263657455837,4.45975235974945,5.09319960112738,5.36523598622979,
5.53913936027954,5.55541982778557,5.8077795608208),.UNSPECIFIED.);
#4309=B_SPLINE_CURVE_WITH_KNOTS('',3,(#54602,#54603,#54604,#54605,#54606,
#54607,#54608,#54609,#54610,#54611,#54612,#54613,#54614,#54615,#54616,#54617,
#54618,#54619,#54620,#54621,#54622,#54623,#54624,#54625,#54626,#54627,#54628,
#54629,#54630,#54631,#54632,#54633,#54634,#54635,#54636,#54637,#54638,#54639,
#54640,#54641,#54642,#54643,#54644,#54645,#54646,#54647,#54648,#54649,#54650,
#54651,#54652,#54653),.UNSPECIFIED.,.F.,.F.,(4,3,3,3,3,3,3,3,3,3,3,3,3,
3,3,3,3,4),(-7.12936284888383,-6.73503958477952,-5.85541919513442,-5.49840246625061,
-4.52430912838489,-4.07614123472496,-3.82946470561722,-3.04197748771621,
-2.81695323173874,-2.47734651379395,-2.0972577337344,-1.90438470269788,
-1.69190045751967,-1.20885650091009,-0.931359575004032,-0.50480048003733,
-0.268904979571053,-0.0293416084169338),.UNSPECIFIED.);
#4310=B_SPLINE_CURVE_WITH_KNOTS('',3,(#54654,#54655,#54656,#54657),
 .UNSPECIFIED.,.F.,.F.,(4,4),(0.0499738749069921,0.152077174974249),
 .UNSPECIFIED.);
#4311=B_SPLINE_CURVE_WITH_KNOTS('',3,(#54836,#54837,#54838,#54839,#54840,
#54841,#54842,#54843,#54844,#54845,#54846,#54847,#54848,#54849,#54850,#54851,
#54852,#54853,#54854,#54855,#54856,#54857,#54858,#54859,#54860,#54861,#54862,
#54863,#54864,#54865,#54866,#54867,#54868,#54869,#54870,#54871,#54872,#54873,
#54874,#54875,#54876,#54877,#54878,#54879,#54880,#54881),.UNSPECIFIED.,
 .F.,.F.,(4,3,3,3,3,3,3,3,3,3,3,3,3,3,3,4),(-3.56163244787237,-3.30468798681601,
-3.18832863247848,-3.0331796444491,-2.79853132696934,-2.75550071531438,
-2.5240431818579,-2.4152503735364,-2.16219512344052,-1.94576347075244,-1.75875950760127,
-1.34373914266267,-1.06103160839734,-0.696688766676754,-0.248712120244055,
0.),.UNSPECIFIED.);
#4312=B_SPLINE_CURVE_WITH_KNOTS('',3,(#54883,#54884,#54885,#54886,#54887,
#54888),.UNSPECIFIED.,.F.,.F.,(4,2,4),(-1.81367248236635,-1.45004244433882,
-0.253045058252053),.UNSPECIFIED.);
#4313=B_SPLINE_CURVE_WITH_KNOTS('',3,(#54890,#54891,#54892,#54893,#54894,
#54895,#54896,#54897,#54898,#54899,#54900,#54901),.UNSPECIFIED.,.F.,.F.,
(4,2,2,2,2,4),(1.08484844498112,2.49572829361744,3.80512145389228,4.87611899720136,
6.43508432402471,7.63234746756005),.UNSPECIFIED.);
#4314=B_SPLINE_CURVE_WITH_KNOTS('',3,(#54902,#54903,#54904,#54905,#54906,
#54907),.UNSPECIFIED.,.F.,.F.,(4,2,4),(0.,0.791088048129032,1.08484844498112),
 .UNSPECIFIED.);
#4315=B_SPLINE_CURVE_WITH_KNOTS('',3,(#54910,#54911,#54912,#54913,#54914,
#54915),.UNSPECIFIED.,.F.,.F.,(4,2,4),(-0.465430185158785,-0.379477414403806,
-0.212084448966329),.UNSPECIFIED.);
#4316=B_SPLINE_CURVE_WITH_KNOTS('',3,(#54917,#54918,#54919,#54920),
 .UNSPECIFIED.,.F.,.F.,(4,4),(-3.09523587865368,-0.674081646507512),
 .UNSPECIFIED.);
#4317=B_SPLINE_CURVE_WITH_KNOTS('',3,(#55197,#55198,#55199,#55200,#55201,
#55202,#55203,#55204,#55205,#55206,#55207,#55208,#55209,#55210,#55211,#55212,
#55213,#55214,#55215,#55216,#55217,#55218,#55219,#55220,#55221,#55222,#55223,
#55224,#55225,#55226,#55227,#55228,#55229,#55230,#55231,#55232,#55233,#55234,
#55235,#55236,#55237,#55238,#55239,#55240,#55241,#55242),.UNSPECIFIED.,
 .F.,.F.,(4,3,3,3,3,3,3,3,3,3,3,3,3,3,3,4),(0.,0.929985381254847,1.44146186475097,
1.65956723730638,2.03170963890849,2.30194659407532,2.89554149400049,3.67764692687497,
4.06869964331221,4.3263657455837,4.45975235974945,5.09319960112738,5.36523598623038,
5.5391393602794,5.55541982778557,5.8077795608208),.UNSPECIFIED.);
#4318=B_SPLINE_CURVE_WITH_KNOTS('',3,(#55419,#55420,#55421,#55422,#55423,
#55424,#55425,#55426,#55427,#55428,#55429,#55430,#55431,#55432,#55433,#55434,
#55435,#55436,#55437,#55438,#55439,#55440,#55441,#55442,#55443,#55444,#55445,
#55446,#55447,#55448,#55449,#55450,#55451,#55452,#55453,#55454,#55455,#55456,
#55457,#55458,#55459,#55460,#55461,#55462,#55463,#55464,#55465,#55466,#55467,
#55468,#55469,#55470),.UNSPECIFIED.,.F.,.F.,(4,3,3,3,3,3,3,3,3,3,3,3,3,
3,3,3,3,4),(-7.12936285432264,-6.73503958969706,-5.85541920372173,-5.49840246875718,
-4.5243091253641,-4.07614123673017,-3.82946470246266,-3.04197748581819,
-2.81695323012233,-2.47734651269469,-2.0972577332487,-1.90438470249889,
-1.69190045792947,-1.20885650078461,-0.931359574963469,-0.504800480033217,
-0.268904979561171,-0.0293416084169337),.UNSPECIFIED.);
#4319=B_SPLINE_CURVE_WITH_KNOTS('',3,(#55471,#55472,#55473,#55474),
 .UNSPECIFIED.,.F.,.F.,(4,4),(0.0499738749012791,0.152077174927713),
 .UNSPECIFIED.);
#4320=B_SPLINE_CURVE_WITH_KNOTS('',3,(#55653,#55654,#55655,#55656,#55657,
#55658,#55659,#55660,#55661,#55662,#55663,#55664,#55665,#55666,#55667,#55668,
#55669,#55670,#55671,#55672,#55673,#55674,#55675,#55676,#55677,#55678,#55679,
#55680,#55681,#55682,#55683,#55684,#55685,#55686,#55687,#55688,#55689,#55690,
#55691,#55692,#55693,#55694,#55695,#55696,#55697,#55698),.UNSPECIFIED.,
 .F.,.F.,(4,3,3,3,3,3,3,3,3,3,3,3,3,3,3,4),(-3.56163244820022,-3.30468798707926,
-3.18832863265333,-3.03317964460065,-2.79853132683733,-2.75550071536956,
-2.52404318190956,-2.41525037355576,-2.16219512362947,-1.94576347077181,
-1.75875950761541,-1.34373914267237,-1.06103160840431,-0.696688766670289,
-0.248712120244514,0.),.UNSPECIFIED.);
#4321=B_SPLINE_CURVE_WITH_KNOTS('',3,(#55700,#55701,#55702,#55703,#55704,
#55705),.UNSPECIFIED.,.F.,.F.,(4,2,4),(-1.81367248236635,-1.45004244433882,
-0.253045058252053),.UNSPECIFIED.);
#4322=B_SPLINE_CURVE_WITH_KNOTS('',3,(#55707,#55708,#55709,#55710,#55711,
#55712,#55713,#55714,#55715,#55716,#55717,#55718),.UNSPECIFIED.,.F.,.F.,
(4,2,2,2,2,4),(1.08484844498112,2.49572829361744,3.80512145389228,4.87611899720136,
6.43508432402471,7.63234746756005),.UNSPECIFIED.);
#4323=B_SPLINE_CURVE_WITH_KNOTS('',3,(#55719,#55720,#55721,#55722,#55723,
#55724),.UNSPECIFIED.,.F.,.F.,(4,2,4),(0.,0.791088048129032,1.08484844498112),
 .UNSPECIFIED.);
#4324=B_SPLINE_CURVE_WITH_KNOTS('',3,(#55727,#55728,#55729,#55730,#55731,
#55732),.UNSPECIFIED.,.F.,.F.,(4,2,4),(-0.461840180389379,-0.379477414403805,
-0.309127170343164),.UNSPECIFIED.);
#4325=B_SPLINE_CURVE_WITH_KNOTS('',3,(#55734,#55735,#55736,#55737),
 .UNSPECIFIED.,.F.,.F.,(4,4),(-0.562176391928348,-0.461840180389379),
 .UNSPECIFIED.);
#4326=B_SPLINE_CURVE_WITH_KNOTS('',3,(#55739,#55740,#55741,#55742),
 .UNSPECIFIED.,.F.,.F.,(4,4),(-3.09523587865368,-0.674081646507512),
 .UNSPECIFIED.);
#4327=B_SPLINE_CURVE_WITH_KNOTS('',3,(#56019,#56020,#56021,#56022,#56023,
#56024,#56025,#56026,#56027,#56028,#56029,#56030,#56031,#56032,#56033,#56034,
#56035,#56036,#56037,#56038,#56039,#56040,#56041,#56042,#56043,#56044,#56045,
#56046,#56047,#56048,#56049,#56050,#56051,#56052,#56053,#56054,#56055,#56056,
#56057,#56058,#56059,#56060,#56061,#56062,#56063,#56064),.UNSPECIFIED.,
 .F.,.F.,(4,3,3,3,3,3,3,3,3,3,3,3,3,3,3,4),(0.,0.929985381254847,1.44146186474925,
1.65956723730638,2.03170963890846,2.30194659407528,2.89554149400049,3.67764692687497,
4.06869964331221,4.3263657455837,4.45975235974945,5.09319960112738,5.36523598622953,
5.53913936027956,5.55541982778557,5.8077795608208),.UNSPECIFIED.);
#4328=B_SPLINE_CURVE_WITH_KNOTS('',3,(#56245,#56246,#56247,#56248),
 .UNSPECIFIED.,.F.,.F.,(4,4),(-0.172427513903814,-0.0293416084169363),
 .UNSPECIFIED.);
#4329=B_SPLINE_CURVE_WITH_KNOTS('',3,(#56249,#56250,#56251,#56252),
 .UNSPECIFIED.,.F.,.F.,(4,4),(0.0499738748984973,0.152077174905035),
 .UNSPECIFIED.);
#4330=B_SPLINE_CURVE_WITH_KNOTS('',3,(#56539,#56540,#56541,#56542,#56543,
#56544,#56545,#56546,#56547,#56548,#56549,#56550,#56551,#56552,#56553,#56554,
#56555,#56556,#56557,#56558,#56559,#56560,#56561,#56562,#56563,#56564,#56565,
#56566,#56567,#56568,#56569,#56570,#56571,#56572,#56573,#56574,#56575,#56576,
#56577,#56578,#56579,#56580,#56581,#56582,#56583,#56584,#56585,#56586,#56587,
#56588,#56589,#56590),.UNSPECIFIED.,.F.,.F.,(4,3,3,3,3,3,3,3,3,3,3,3,3,
3,3,3,3,4),(-7.12936283895551,-6.73503957583632,-5.85541917810278,-5.49840246204903,
-4.52430913563507,-4.07614123114609,-3.82946471293636,-3.04197749212362,
-2.81695323547345,-2.47734651631999,-2.09725773484647,-1.90438470315448,
-1.69190045657557,-1.20885650119729,-0.931359575096543,-0.504800480046614,
-0.268904979590904,-0.0293416084169361),.UNSPECIFIED.);
#4331=B_SPLINE_CURVE_WITH_KNOTS('',3,(#56592,#56593,#56594,#56595,#56596,
#56597),.UNSPECIFIED.,.F.,.F.,(4,2,4),(-0.427788912726286,-0.283829973314833,
-0.17460945272576),.UNSPECIFIED.);
#4332=B_SPLINE_CURVE_WITH_KNOTS('',3,(#56598,#56599,#56600,#56601,#56602,
#56603,#56604,#56605,#56606,#56607,#56608,#56609,#56610,#56611,#56612,#56613,
#56614,#56615,#56616,#56617,#56618,#56619,#56620,#56621,#56622,#56623,#56624,
#56625),.UNSPECIFIED.,.F.,.F.,(4,3,3,3,3,3,3,3,3,4),(-3.56163244767533,
-3.30468798665615,-3.18832863236903,-3.03317964435316,-2.79853132703271,
-2.75550071527398,-2.5240431818226,-2.41525037351813,-2.15906056771207,
-1.95549230332054),.UNSPECIFIED.);
#4333=B_SPLINE_CURVE_WITH_KNOTS('',3,(#56802,#56803,#56804,#56805,#56806,
#56807),.UNSPECIFIED.,.F.,.F.,(4,2,4),(-1.81367248236635,-1.45004244433882,
-0.253045058252053),.UNSPECIFIED.);
#4334=B_SPLINE_CURVE_WITH_KNOTS('',3,(#56809,#56810,#56811,#56812,#56813,
#56814,#56815,#56816,#56817,#56818,#56819,#56820),.UNSPECIFIED.,.F.,.F.,
(4,2,2,2,2,4),(1.08484844498112,2.49572829361744,3.80512145389228,4.87611899720136,
6.43508432402471,7.63234746756005),.UNSPECIFIED.);
#4335=B_SPLINE_CURVE_WITH_KNOTS('',3,(#56821,#56822,#56823,#56824,#56825,
#56826),.UNSPECIFIED.,.F.,.F.,(4,2,4),(0.,0.791088048129032,1.08484844498112),
 .UNSPECIFIED.);
#4336=B_SPLINE_CURVE_WITH_KNOTS('',3,(#56829,#56830,#56831,#56832),
 .UNSPECIFIED.,.F.,.F.,(4,4),(-3.09523587865368,-0.674081646507512),
 .UNSPECIFIED.);
#4337=B_SPLINE_CURVE_WITH_KNOTS('',3,(#57109,#57110,#57111,#57112,#57113,
#57114,#57115,#57116,#57117,#57118,#57119,#57120,#57121,#57122,#57123,#57124,
#57125,#57126,#57127,#57128,#57129,#57130,#57131,#57132,#57133,#57134,#57135,
#57136,#57137,#57138,#57139,#57140,#57141,#57142,#57143,#57144,#57145,#57146,
#57147,#57148,#57149,#57150,#57151,#57152,#57153,#57154),.UNSPECIFIED.,
 .F.,.F.,(4,3,3,3,3,3,3,3,3,3,3,3,3,3,3,4),(0.,0.929985381254847,1.44146186475013,
1.65956723730638,2.03170963890882,2.30194659407531,2.89554149400049,3.67764692687497,
4.06869964331221,4.3263657455837,4.45975235974945,5.09319960112738,5.36523598623043,
5.5391393602794,5.55541982778557,5.8077795608208),.UNSPECIFIED.);
#4338=B_SPLINE_CURVE_WITH_KNOTS('',3,(#57365,#57366,#57367,#57368),
 .UNSPECIFIED.,.F.,.F.,(4,4),(0.0499738749129155,0.152077175022647),
 .UNSPECIFIED.);
#5348=LINE('',#47684,#6760);
#5349=LINE('',#48050,#6761);
#5350=LINE('',#48059,#6762);
#5351=LINE('',#48065,#6763);
#5352=LINE('',#57370,#6764);
#5353=LINE('',#57375,#6765);
#5354=LINE('',#57379,#6766);
#5355=LINE('',#57381,#6767);
#6760=VECTOR('',#22192,39.);
#6761=VECTOR('',#22281,3.675);
#6762=VECTOR('',#22292,3.525);
#6763=VECTOR('',#22299,3.675);
#6764=VECTOR('',#22418,38.75);
#6765=VECTOR('',#22425,8.95);
#6766=VECTOR('',#22430,8.7);
#6767=VECTOR('',#22433,8.4);
#8384=VERTEX_POINT('',#47336);
#8385=VERTEX_POINT('',#47337);
#8386=VERTEX_POINT('',#47355);
#8387=VERTEX_POINT('',#47375);
#8388=VERTEX_POINT('',#47377);
#8389=VERTEX_POINT('',#47392);
#8390=VERTEX_POINT('',#47397);
#8391=VERTEX_POINT('',#47426);
#8392=VERTEX_POINT('',#47481);
#8393=VERTEX_POINT('',#47482);
#8394=VERTEX_POINT('',#47487);
#8395=VERTEX_POINT('',#47489);
#8396=VERTEX_POINT('',#47496);
#8397=VERTEX_POINT('',#47501);
#8398=VERTEX_POINT('',#47506);
#8399=VERTEX_POINT('',#47513);
#8400=VERTEX_POINT('',#47515);
#8401=VERTEX_POINT('',#47522);
#8402=VERTEX_POINT('',#47527);
#8403=VERTEX_POINT('',#47529);
#8404=VERTEX_POINT('',#47534);
#8405=VERTEX_POINT('',#47541);
#8406=VERTEX_POINT('',#47543);
#8407=VERTEX_POINT('',#47550);
#8408=VERTEX_POINT('',#47555);
#8409=VERTEX_POINT('',#47557);
#8410=VERTEX_POINT('',#47562);
#8411=VERTEX_POINT('',#47569);
#8412=VERTEX_POINT('',#47571);
#8413=VERTEX_POINT('',#47578);
#8414=VERTEX_POINT('',#47583);
#8415=VERTEX_POINT('',#47585);
#8416=VERTEX_POINT('',#47590);
#8417=VERTEX_POINT('',#47597);
#8418=VERTEX_POINT('',#47599);
#8419=VERTEX_POINT('',#47606);
#8420=VERTEX_POINT('',#47611);
#8421=VERTEX_POINT('',#47613);
#8422=VERTEX_POINT('',#47618);
#8423=VERTEX_POINT('',#47625);
#8424=VERTEX_POINT('',#47627);
#8425=VERTEX_POINT('',#47634);
#8426=VERTEX_POINT('',#47639);
#8427=VERTEX_POINT('',#47641);
#8428=VERTEX_POINT('',#47646);
#8429=VERTEX_POINT('',#47653);
#8430=VERTEX_POINT('',#47655);
#8431=VERTEX_POINT('',#47662);
#8432=VERTEX_POINT('',#47667);
#8433=VERTEX_POINT('',#47669);
#8434=VERTEX_POINT('',#47674);
#8435=VERTEX_POINT('',#47681);
#8436=VERTEX_POINT('',#47683);
#8437=VERTEX_POINT('',#47686);
#8438=VERTEX_POINT('',#47688);
#8439=VERTEX_POINT('',#47695);
#8440=VERTEX_POINT('',#47700);
#8441=VERTEX_POINT('',#47702);
#8442=VERTEX_POINT('',#47707);
#8443=VERTEX_POINT('',#47714);
#8444=VERTEX_POINT('',#47716);
#8445=VERTEX_POINT('',#47723);
#8446=VERTEX_POINT('',#47728);
#8447=VERTEX_POINT('',#47730);
#8448=VERTEX_POINT('',#47735);
#8449=VERTEX_POINT('',#47742);
#8450=VERTEX_POINT('',#47744);
#8451=VERTEX_POINT('',#47751);
#8452=VERTEX_POINT('',#47756);
#8453=VERTEX_POINT('',#47758);
#8454=VERTEX_POINT('',#47763);
#8455=VERTEX_POINT('',#47770);
#8456=VERTEX_POINT('',#47772);
#8457=VERTEX_POINT('',#47779);
#8458=VERTEX_POINT('',#47784);
#8459=VERTEX_POINT('',#47786);
#8460=VERTEX_POINT('',#47791);
#8461=VERTEX_POINT('',#47798);
#8462=VERTEX_POINT('',#47800);
#8463=VERTEX_POINT('',#47807);
#8464=VERTEX_POINT('',#47812);
#8465=VERTEX_POINT('',#47814);
#8466=VERTEX_POINT('',#47819);
#8467=VERTEX_POINT('',#47826);
#8468=VERTEX_POINT('',#47828);
#8469=VERTEX_POINT('',#47835);
#8470=VERTEX_POINT('',#47840);
#8471=VERTEX_POINT('',#47842);
#8472=VERTEX_POINT('',#47847);
#8473=VERTEX_POINT('',#47854);
#8474=VERTEX_POINT('',#47856);
#8475=VERTEX_POINT('',#47863);
#8476=VERTEX_POINT('',#47868);
#8477=VERTEX_POINT('',#47870);
#8478=VERTEX_POINT('',#47875);
#8479=VERTEX_POINT('',#47882);
#8480=VERTEX_POINT('',#47891);
#8481=VERTEX_POINT('',#47896);
#8482=VERTEX_POINT('',#47903);
#8483=VERTEX_POINT('',#47908);
#8484=VERTEX_POINT('',#47915);
#8485=VERTEX_POINT('',#47920);
#8486=VERTEX_POINT('',#47927);
#8487=VERTEX_POINT('',#47932);
#8488=VERTEX_POINT('',#47939);
#8489=VERTEX_POINT('',#47944);
#8490=VERTEX_POINT('',#47951);
#8491=VERTEX_POINT('',#47956);
#8492=VERTEX_POINT('',#47963);
#8493=VERTEX_POINT('',#47968);
#8494=VERTEX_POINT('',#47975);
#8495=VERTEX_POINT('',#47980);
#8496=VERTEX_POINT('',#47987);
#8497=VERTEX_POINT('',#47992);
#8498=VERTEX_POINT('',#47999);
#8499=VERTEX_POINT('',#48004);
#8500=VERTEX_POINT('',#48011);
#8501=VERTEX_POINT('',#48016);
#8502=VERTEX_POINT('',#48023);
#8503=VERTEX_POINT('',#48028);
#8504=VERTEX_POINT('',#48035);
#8505=VERTEX_POINT('',#48040);
#8506=VERTEX_POINT('',#48047);
#8507=VERTEX_POINT('',#48049);
#8508=VERTEX_POINT('',#48051);
#8509=VERTEX_POINT('',#48055);
#8510=VERTEX_POINT('',#48056);
#8511=VERTEX_POINT('',#48061);
#8512=VERTEX_POINT('',#48064);
#8513=VERTEX_POINT('',#48068);
#8514=VERTEX_POINT('',#48178);
#8515=VERTEX_POINT('',#48183);
#8516=VERTEX_POINT('',#48212);
#8517=VERTEX_POINT('',#48246);
#8518=VERTEX_POINT('',#48251);
#8519=VERTEX_POINT('',#48514);
#8520=VERTEX_POINT('',#48534);
#8521=VERTEX_POINT('',#48648);
#8522=VERTEX_POINT('',#48653);
#8523=VERTEX_POINT('',#48682);
#8524=VERTEX_POINT('',#48716);
#8525=VERTEX_POINT('',#48721);
#8526=VERTEX_POINT('',#48984);
#8527=VERTEX_POINT('',#49004);
#8528=VERTEX_POINT('',#49118);
#8529=VERTEX_POINT('',#49123);
#8530=VERTEX_POINT('',#49152);
#8531=VERTEX_POINT('',#49186);
#8532=VERTEX_POINT('',#49191);
#8533=VERTEX_POINT('',#49454);
#8534=VERTEX_POINT('',#49474);
#8535=VERTEX_POINT('',#49588);
#8536=VERTEX_POINT('',#49593);
#8537=VERTEX_POINT('',#49622);
#8538=VERTEX_POINT('',#49656);
#8539=VERTEX_POINT('',#49663);
#8540=VERTEX_POINT('',#49926);
#8541=VERTEX_POINT('',#49946);
#8542=VERTEX_POINT('',#50060);
#8543=VERTEX_POINT('',#50065);
#8544=VERTEX_POINT('',#50094);
#8545=VERTEX_POINT('',#50128);
#8546=VERTEX_POINT('',#50135);
#8547=VERTEX_POINT('',#50398);
#8548=VERTEX_POINT('',#50418);
#8549=VERTEX_POINT('',#50532);
#8550=VERTEX_POINT('',#50537);
#8551=VERTEX_POINT('',#50566);
#8552=VERTEX_POINT('',#50600);
#8553=VERTEX_POINT('',#50605);
#8554=VERTEX_POINT('',#50868);
#8555=VERTEX_POINT('',#50888);
#8556=VERTEX_POINT('',#51006);
#8557=VERTEX_POINT('',#51040);
#8558=VERTEX_POINT('',#51487);
#8559=VERTEX_POINT('',#51534);
#8560=VERTEX_POINT('',#51541);
#8561=VERTEX_POINT('',#51561);
#8562=VERTEX_POINT('',#51568);
#8563=VERTEX_POINT('',#52075);
#8564=VERTEX_POINT('',#52309);
#8565=VERTEX_POINT('',#52356);
#8566=VERTEX_POINT('',#52363);
#8567=VERTEX_POINT('',#52383);
#8568=VERTEX_POINT('',#52390);
#8569=VERTEX_POINT('',#52927);
#8570=VERTEX_POINT('',#53166);
#8571=VERTEX_POINT('',#53213);
#8572=VERTEX_POINT('',#53220);
#8573=VERTEX_POINT('',#53240);
#8574=VERTEX_POINT('',#53247);
#8575=VERTEX_POINT('',#53749);
#8576=VERTEX_POINT('',#53983);
#8577=VERTEX_POINT('',#54030);
#8578=VERTEX_POINT('',#54037);
#8579=VERTEX_POINT('',#54057);
#8580=VERTEX_POINT('',#54064);
#8581=VERTEX_POINT('',#54601);
#8582=VERTEX_POINT('',#54835);
#8583=VERTEX_POINT('',#54882);
#8584=VERTEX_POINT('',#54889);
#8585=VERTEX_POINT('',#54909);
#8586=VERTEX_POINT('',#54916);
#8587=VERTEX_POINT('',#55418);
#8588=VERTEX_POINT('',#55652);
#8589=VERTEX_POINT('',#55699);
#8590=VERTEX_POINT('',#55706);
#8591=VERTEX_POINT('',#55726);
#8592=VERTEX_POINT('',#55733);
#8593=VERTEX_POINT('',#55738);
#8594=VERTEX_POINT('',#56524);
#8595=VERTEX_POINT('',#56533);
#8596=VERTEX_POINT('',#56536);
#8597=VERTEX_POINT('',#56538);
#8598=VERTEX_POINT('',#56591);
#8599=VERTEX_POINT('',#56801);
#8600=VERTEX_POINT('',#56808);
#8601=VERTEX_POINT('',#56828);
#8602=VERTEX_POINT('',#57373);
#8603=VERTEX_POINT('',#57377);
#10723=EDGE_CURVE('',#8384,#8385,#1054,.T.);
#10724=EDGE_CURVE('',#8384,#8386,#4119,.T.);
#10725=EDGE_CURVE('',#8386,#8387,#3568,.T.);
#10726=EDGE_CURVE('',#8387,#8388,#4120,.T.);
#10727=EDGE_CURVE('',#8388,#8389,#4121,.T.);
#10728=EDGE_CURVE('',#8389,#8390,#4122,.T.);
#10729=EDGE_CURVE('',#8390,#8391,#3569,.T.);
#10730=EDGE_CURVE('',#8391,#8385,#4123,.T.);
#10731=EDGE_CURVE('',#8392,#8393,#4124,.F.);
#10732=EDGE_CURVE('',#8393,#8394,#3570,.T.);
#10733=EDGE_CURVE('',#8394,#8395,#4125,.F.);
#10734=EDGE_CURVE('',#8395,#8392,#3571,.T.);
#10735=EDGE_CURVE('',#8394,#8396,#4126,.T.);
#10736=EDGE_CURVE('',#8397,#8393,#4127,.T.);
#10737=EDGE_CURVE('',#8397,#8398,#4128,.T.);
#10738=EDGE_CURVE('',#8399,#8398,#3572,.T.);
#10739=EDGE_CURVE('',#8399,#8400,#4129,.T.);
#10740=EDGE_CURVE('',#8401,#8400,#4130,.T.);
#10741=EDGE_CURVE('',#8402,#8401,#3573,.T.);
#10742=EDGE_CURVE('',#8403,#8402,#4131,.T.);
#10743=EDGE_CURVE('',#8403,#8404,#4132,.T.);
#10744=EDGE_CURVE('',#8405,#8404,#3574,.T.);
#10745=EDGE_CURVE('',#8405,#8406,#4133,.T.);
#10746=EDGE_CURVE('',#8407,#8406,#4134,.T.);
#10747=EDGE_CURVE('',#8408,#8407,#3575,.T.);
#10748=EDGE_CURVE('',#8409,#8408,#4135,.T.);
#10749=EDGE_CURVE('',#8409,#8410,#4136,.T.);
#10750=EDGE_CURVE('',#8411,#8410,#3576,.T.);
#10751=EDGE_CURVE('',#8411,#8412,#4137,.T.);
#10752=EDGE_CURVE('',#8413,#8412,#4138,.T.);
#10753=EDGE_CURVE('',#8414,#8413,#3577,.T.);
#10754=EDGE_CURVE('',#8415,#8414,#4139,.T.);
#10755=EDGE_CURVE('',#8415,#8416,#4140,.T.);
#10756=EDGE_CURVE('',#8417,#8416,#3578,.T.);
#10757=EDGE_CURVE('',#8417,#8418,#4141,.T.);
#10758=EDGE_CURVE('',#8419,#8418,#4142,.T.);
#10759=EDGE_CURVE('',#8420,#8419,#3579,.T.);
#10760=EDGE_CURVE('',#8421,#8420,#4143,.T.);
#10761=EDGE_CURVE('',#8421,#8422,#4144,.T.);
#10762=EDGE_CURVE('',#8423,#8422,#3580,.T.);
#10763=EDGE_CURVE('',#8423,#8424,#4145,.T.);
#10764=EDGE_CURVE('',#8425,#8424,#4146,.T.);
#10765=EDGE_CURVE('',#8426,#8425,#3581,.T.);
#10766=EDGE_CURVE('',#8427,#8426,#4147,.T.);
#10767=EDGE_CURVE('',#8427,#8428,#4148,.T.);
#10768=EDGE_CURVE('',#8429,#8428,#3582,.T.);
#10769=EDGE_CURVE('',#8429,#8430,#4149,.T.);
#10770=EDGE_CURVE('',#8431,#8430,#4150,.T.);
#10771=EDGE_CURVE('',#8432,#8431,#3583,.T.);
#10772=EDGE_CURVE('',#8433,#8432,#4151,.T.);
#10773=EDGE_CURVE('',#8433,#8434,#4152,.T.);
#10774=EDGE_CURVE('',#8435,#8434,#3584,.T.);
#10775=EDGE_CURVE('',#8435,#8436,#5348,.T.);
#10776=EDGE_CURVE('',#8436,#8436,#3585,.T.);
#10777=EDGE_CURVE('',#8437,#8435,#3586,.T.);
#10778=EDGE_CURVE('',#8437,#8438,#4153,.T.);
#10779=EDGE_CURVE('',#8439,#8438,#4154,.T.);
#10780=EDGE_CURVE('',#8440,#8439,#3587,.T.);
#10781=EDGE_CURVE('',#8441,#8440,#4155,.T.);
#10782=EDGE_CURVE('',#8441,#8442,#4156,.T.);
#10783=EDGE_CURVE('',#8443,#8442,#3588,.T.);
#10784=EDGE_CURVE('',#8443,#8444,#4157,.T.);
#10785=EDGE_CURVE('',#8445,#8444,#4158,.T.);
#10786=EDGE_CURVE('',#8446,#8445,#3589,.T.);
#10787=EDGE_CURVE('',#8447,#8446,#4159,.T.);
#10788=EDGE_CURVE('',#8447,#8448,#4160,.T.);
#10789=EDGE_CURVE('',#8449,#8448,#3590,.T.);
#10790=EDGE_CURVE('',#8449,#8450,#4161,.T.);
#10791=EDGE_CURVE('',#8451,#8450,#4162,.T.);
#10792=EDGE_CURVE('',#8452,#8451,#3591,.T.);
#10793=EDGE_CURVE('',#8453,#8452,#4163,.T.);
#10794=EDGE_CURVE('',#8453,#8454,#4164,.T.);
#10795=EDGE_CURVE('',#8455,#8454,#3592,.T.);
#10796=EDGE_CURVE('',#8455,#8456,#4165,.T.);
#10797=EDGE_CURVE('',#8457,#8456,#4166,.T.);
#10798=EDGE_CURVE('',#8458,#8457,#3593,.T.);
#10799=EDGE_CURVE('',#8459,#8458,#4167,.T.);
#10800=EDGE_CURVE('',#8459,#8460,#4168,.T.);
#10801=EDGE_CURVE('',#8461,#8460,#3594,.T.);
#10802=EDGE_CURVE('',#8461,#8462,#4169,.T.);
#10803=EDGE_CURVE('',#8463,#8462,#4170,.T.);
#10804=EDGE_CURVE('',#8464,#8463,#3595,.T.);
#10805=EDGE_CURVE('',#8465,#8464,#4171,.T.);
#10806=EDGE_CURVE('',#8465,#8466,#4172,.T.);
#10807=EDGE_CURVE('',#8467,#8466,#3596,.T.);
#10808=EDGE_CURVE('',#8467,#8468,#4173,.T.);
#10809=EDGE_CURVE('',#8469,#8468,#4174,.T.);
#10810=EDGE_CURVE('',#8470,#8469,#3597,.T.);
#10811=EDGE_CURVE('',#8471,#8470,#4175,.T.);
#10812=EDGE_CURVE('',#8471,#8472,#4176,.T.);
#10813=EDGE_CURVE('',#8473,#8472,#3598,.T.);
#10814=EDGE_CURVE('',#8473,#8474,#4177,.T.);
#10815=EDGE_CURVE('',#8475,#8474,#4178,.T.);
#10816=EDGE_CURVE('',#8476,#8475,#3599,.T.);
#10817=EDGE_CURVE('',#8477,#8476,#4179,.T.);
#10818=EDGE_CURVE('',#8477,#8478,#4180,.T.);
#10819=EDGE_CURVE('',#8479,#8478,#3600,.T.);
#10820=EDGE_CURVE('',#8479,#8396,#4181,.T.);
#10821=EDGE_CURVE('',#8480,#8470,#4182,.F.);
#10822=EDGE_CURVE('',#8469,#8481,#4183,.F.);
#10823=EDGE_CURVE('',#8481,#8480,#3601,.T.);
#10824=EDGE_CURVE('',#8482,#8458,#4184,.F.);
#10825=EDGE_CURVE('',#8457,#8483,#4185,.F.);
#10826=EDGE_CURVE('',#8483,#8482,#3602,.T.);
#10827=EDGE_CURVE('',#8484,#8446,#4186,.F.);
#10828=EDGE_CURVE('',#8445,#8485,#4187,.F.);
#10829=EDGE_CURVE('',#8485,#8484,#3603,.T.);
#10830=EDGE_CURVE('',#8486,#8432,#4188,.F.);
#10831=EDGE_CURVE('',#8431,#8487,#4189,.F.);
#10832=EDGE_CURVE('',#8487,#8486,#3604,.T.);
#10833=EDGE_CURVE('',#8488,#8420,#4190,.F.);
#10834=EDGE_CURVE('',#8419,#8489,#4191,.F.);
#10835=EDGE_CURVE('',#8489,#8488,#3605,.T.);
#10836=EDGE_CURVE('',#8490,#8408,#4192,.F.);
#10837=EDGE_CURVE('',#8407,#8491,#4193,.F.);
#10838=EDGE_CURVE('',#8491,#8490,#3606,.T.);
#10839=EDGE_CURVE('',#8492,#8476,#4194,.F.);
#10840=EDGE_CURVE('',#8475,#8493,#4195,.F.);
#10841=EDGE_CURVE('',#8493,#8492,#3607,.T.);
#10842=EDGE_CURVE('',#8494,#8464,#4196,.F.);
#10843=EDGE_CURVE('',#8463,#8495,#4197,.F.);
#10844=EDGE_CURVE('',#8495,#8494,#3608,.T.);
#10845=EDGE_CURVE('',#8496,#8452,#4198,.F.);
#10846=EDGE_CURVE('',#8451,#8497,#4199,.F.);
#10847=EDGE_CURVE('',#8497,#8496,#3609,.T.);
#10848=EDGE_CURVE('',#8498,#8440,#4200,.F.);
#10849=EDGE_CURVE('',#8439,#8499,#4201,.F.);
#10850=EDGE_CURVE('',#8499,#8498,#3610,.T.);
#10851=EDGE_CURVE('',#8500,#8426,#4202,.F.);
#10852=EDGE_CURVE('',#8425,#8501,#4203,.F.);
#10853=EDGE_CURVE('',#8501,#8500,#3611,.T.);
#10854=EDGE_CURVE('',#8502,#8414,#4204,.F.);
#10855=EDGE_CURVE('',#8413,#8503,#4205,.F.);
#10856=EDGE_CURVE('',#8503,#8502,#3612,.T.);
#10857=EDGE_CURVE('',#8504,#8402,#4206,.F.);
#10858=EDGE_CURVE('',#8401,#8505,#4207,.F.);
#10859=EDGE_CURVE('',#8505,#8504,#3613,.T.);
#10860=EDGE_CURVE('',#8506,#8506,#3614,.T.);
#10861=EDGE_CURVE('',#8506,#8507,#5349,.T.);
#10862=EDGE_CURVE('',#8507,#8508,#3615,.T.);
#10863=EDGE_CURVE('',#8508,#8507,#3616,.T.);
#10864=EDGE_CURVE('',#8509,#8510,#3617,.T.);
#10865=EDGE_CURVE('',#8510,#8509,#3618,.T.);
#10866=EDGE_CURVE('',#8510,#8508,#5350,.T.);
#10867=EDGE_CURVE('',#8511,#8511,#3619,.T.);
#10868=EDGE_CURVE('',#8509,#8512,#5351,.T.);
#10869=EDGE_CURVE('',#8512,#8512,#3620,.T.);
#10870=EDGE_CURVE('',#8513,#8513,#3621,.T.);
#10871=EDGE_CURVE('',#8514,#8392,#4208,.T.);
#10872=EDGE_CURVE('',#8515,#8514,#4209,.T.);
#10873=EDGE_CURVE('',#8516,#8515,#4210,.T.);
#10874=EDGE_CURVE('',#8398,#8516,#4211,.T.);
#10875=EDGE_CURVE('',#8517,#8515,#4212,.T.);
#10876=EDGE_CURVE('',#8517,#8518,#4213,.T.);
#10877=EDGE_CURVE('',#8518,#8516,#3622,.T.);
#10878=EDGE_CURVE('',#8518,#8399,#4214,.T.);
#10879=EDGE_CURVE('',#8519,#8517,#4215,.T.);
#10880=EDGE_CURVE('',#8505,#8519,#4216,.T.);
#10881=EDGE_CURVE('',#8520,#8519,#3623,.T.);
#10882=EDGE_CURVE('',#8520,#8504,#4217,.T.);
#10883=EDGE_CURVE('',#8521,#8490,#4218,.T.);
#10884=EDGE_CURVE('',#8522,#8521,#4219,.T.);
#10885=EDGE_CURVE('',#8523,#8522,#4220,.T.);
#10886=EDGE_CURVE('',#8410,#8523,#4221,.T.);
#10887=EDGE_CURVE('',#8524,#8522,#4222,.T.);
#10888=EDGE_CURVE('',#8524,#8525,#4223,.T.);
#10889=EDGE_CURVE('',#8525,#8523,#3624,.T.);
#10890=EDGE_CURVE('',#8525,#8411,#4224,.T.);
#10891=EDGE_CURVE('',#8526,#8524,#4225,.T.);
#10892=EDGE_CURVE('',#8503,#8526,#4226,.T.);
#10893=EDGE_CURVE('',#8527,#8526,#3625,.T.);
#10894=EDGE_CURVE('',#8527,#8502,#4227,.T.);
#10895=EDGE_CURVE('',#8528,#8488,#4228,.T.);
#10896=EDGE_CURVE('',#8529,#8528,#4229,.T.);
#10897=EDGE_CURVE('',#8530,#8529,#4230,.T.);
#10898=EDGE_CURVE('',#8422,#8530,#4231,.T.);
#10899=EDGE_CURVE('',#8531,#8529,#4232,.T.);
#10900=EDGE_CURVE('',#8531,#8532,#4233,.T.);
#10901=EDGE_CURVE('',#8532,#8530,#3626,.T.);
#10902=EDGE_CURVE('',#8532,#8423,#4234,.T.);
#10903=EDGE_CURVE('',#8533,#8531,#4235,.T.);
#10904=EDGE_CURVE('',#8501,#8533,#4236,.T.);
#10905=EDGE_CURVE('',#8534,#8533,#3627,.T.);
#10906=EDGE_CURVE('',#8534,#8500,#4237,.T.);
#10907=EDGE_CURVE('',#8535,#8486,#4238,.T.);
#10908=EDGE_CURVE('',#8536,#8535,#4239,.T.);
#10909=EDGE_CURVE('',#8537,#8536,#4240,.T.);
#10910=EDGE_CURVE('',#8434,#8537,#4241,.T.);
#10911=EDGE_CURVE('',#8538,#8536,#4242,.T.);
#10912=EDGE_CURVE('',#8538,#8539,#4243,.T.);
#10913=EDGE_CURVE('',#8539,#8537,#3628,.T.);
#10914=EDGE_CURVE('',#8539,#8437,#4244,.T.);
#10915=EDGE_CURVE('',#8540,#8538,#4245,.T.);
#10916=EDGE_CURVE('',#8499,#8540,#4246,.T.);
#10917=EDGE_CURVE('',#8541,#8540,#3629,.T.);
#10918=EDGE_CURVE('',#8541,#8498,#4247,.T.);
#10919=EDGE_CURVE('',#8542,#8484,#4248,.T.);
#10920=EDGE_CURVE('',#8543,#8542,#4249,.T.);
#10921=EDGE_CURVE('',#8544,#8543,#4250,.T.);
#10922=EDGE_CURVE('',#8448,#8544,#4251,.T.);
#10923=EDGE_CURVE('',#8545,#8543,#4252,.T.);
#10924=EDGE_CURVE('',#8545,#8546,#4253,.T.);
#10925=EDGE_CURVE('',#8546,#8544,#3630,.T.);
#10926=EDGE_CURVE('',#8546,#8449,#4254,.T.);
#10927=EDGE_CURVE('',#8547,#8545,#4255,.T.);
#10928=EDGE_CURVE('',#8497,#8547,#4256,.T.);
#10929=EDGE_CURVE('',#8548,#8547,#3631,.T.);
#10930=EDGE_CURVE('',#8548,#8496,#4257,.T.);
#10931=EDGE_CURVE('',#8549,#8482,#4258,.T.);
#10932=EDGE_CURVE('',#8550,#8549,#4259,.T.);
#10933=EDGE_CURVE('',#8551,#8550,#4260,.T.);
#10934=EDGE_CURVE('',#8460,#8551,#4261,.T.);
#10935=EDGE_CURVE('',#8552,#8550,#4262,.T.);
#10936=EDGE_CURVE('',#8552,#8553,#4263,.T.);
#10937=EDGE_CURVE('',#8553,#8551,#3632,.T.);
#10938=EDGE_CURVE('',#8553,#8461,#4264,.T.);
#10939=EDGE_CURVE('',#8554,#8552,#4265,.T.);
#10940=EDGE_CURVE('',#8495,#8554,#4266,.T.);
#10941=EDGE_CURVE('',#8555,#8554,#3633,.T.);
#10942=EDGE_CURVE('',#8555,#8494,#4267,.T.);
#10943=EDGE_CURVE('',#8390,#8480,#4268,.T.);
#10944=EDGE_CURVE('',#8556,#8389,#4269,.T.);
#10945=EDGE_CURVE('',#8472,#8556,#4270,.T.);
#10946=EDGE_CURVE('',#8388,#8557,#4271,.T.);
#10947=EDGE_CURVE('',#8557,#8556,#3634,.T.);
#10948=EDGE_CURVE('',#8557,#8473,#4272,.T.);
#10949=EDGE_CURVE('',#8493,#8387,#4273,.T.);
#10950=EDGE_CURVE('',#8386,#8492,#4274,.T.);
#10951=EDGE_CURVE('',#8558,#8520,#4275,.T.);
#10952=EDGE_CURVE('',#8559,#8558,#4276,.T.);
#10953=EDGE_CURVE('',#8560,#8559,#4277,.T.);
#10954=EDGE_CURVE('',#8404,#8560,#4278,.T.);
#10955=EDGE_CURVE('',#8561,#8558,#4279,.T.);
#10956=EDGE_CURVE('',#8561,#8562,#4280,.T.);
#10957=EDGE_CURVE('',#8562,#8559,#3635,.T.);
#10958=EDGE_CURVE('',#8562,#8405,#4281,.T.);
#10959=EDGE_CURVE('',#8563,#8561,#4282,.T.);
#10960=EDGE_CURVE('',#8491,#8563,#4283,.T.);
#10961=EDGE_CURVE('',#8521,#8563,#3636,.T.);
#10962=EDGE_CURVE('',#8564,#8527,#4284,.T.);
#10963=EDGE_CURVE('',#8565,#8564,#4285,.T.);
#10964=EDGE_CURVE('',#8566,#8565,#4286,.T.);
#10965=EDGE_CURVE('',#8416,#8566,#4287,.T.);
#10966=EDGE_CURVE('',#8567,#8564,#4288,.T.);
#10967=EDGE_CURVE('',#8567,#8568,#4289,.T.);
#10968=EDGE_CURVE('',#8568,#8565,#3637,.T.);
#10969=EDGE_CURVE('',#8568,#8417,#4290,.T.);
#10970=EDGE_CURVE('',#8569,#8567,#4291,.T.);
#10971=EDGE_CURVE('',#8489,#8569,#4292,.T.);
#10972=EDGE_CURVE('',#8528,#8569,#3638,.T.);
#10973=EDGE_CURVE('',#8570,#8534,#4293,.T.);
#10974=EDGE_CURVE('',#8571,#8570,#4294,.T.);
#10975=EDGE_CURVE('',#8572,#8571,#4295,.T.);
#10976=EDGE_CURVE('',#8428,#8572,#4296,.T.);
#10977=EDGE_CURVE('',#8573,#8570,#4297,.T.);
#10978=EDGE_CURVE('',#8573,#8574,#4298,.T.);
#10979=EDGE_CURVE('',#8574,#8571,#3639,.T.);
#10980=EDGE_CURVE('',#8574,#8429,#4299,.T.);
#10981=EDGE_CURVE('',#8575,#8573,#4300,.T.);
#10982=EDGE_CURVE('',#8487,#8575,#4301,.T.);
#10983=EDGE_CURVE('',#8535,#8575,#3640,.T.);
#10984=EDGE_CURVE('',#8576,#8541,#4302,.T.);
#10985=EDGE_CURVE('',#8577,#8576,#4303,.T.);
#10986=EDGE_CURVE('',#8578,#8577,#4304,.T.);
#10987=EDGE_CURVE('',#8442,#8578,#4305,.T.);
#10988=EDGE_CURVE('',#8579,#8576,#4306,.T.);
#10989=EDGE_CURVE('',#8579,#8580,#4307,.T.);
#10990=EDGE_CURVE('',#8580,#8577,#3641,.T.);
#10991=EDGE_CURVE('',#8580,#8443,#4308,.T.);
#10992=EDGE_CURVE('',#8581,#8579,#4309,.T.);
#10993=EDGE_CURVE('',#8485,#8581,#4310,.T.);
#10994=EDGE_CURVE('',#8542,#8581,#3642,.T.);
#10995=EDGE_CURVE('',#8582,#8548,#4311,.T.);
#10996=EDGE_CURVE('',#8583,#8582,#4312,.T.);
#10997=EDGE_CURVE('',#8584,#8583,#4313,.T.);
#10998=EDGE_CURVE('',#8454,#8584,#4314,.T.);
#10999=EDGE_CURVE('',#8585,#8582,#4315,.T.);
#11000=EDGE_CURVE('',#8585,#8586,#4316,.T.);
#11001=EDGE_CURVE('',#8586,#8583,#3643,.T.);
#11002=EDGE_CURVE('',#8586,#8455,#4317,.T.);
#11003=EDGE_CURVE('',#8587,#8585,#4318,.T.);
#11004=EDGE_CURVE('',#8483,#8587,#4319,.T.);
#11005=EDGE_CURVE('',#8549,#8587,#3644,.T.);
#11006=EDGE_CURVE('',#8588,#8555,#4320,.T.);
#11007=EDGE_CURVE('',#8589,#8588,#4321,.T.);
#11008=EDGE_CURVE('',#8590,#8589,#4322,.T.);
#11009=EDGE_CURVE('',#8466,#8590,#4323,.T.);
#11010=EDGE_CURVE('',#8591,#8588,#4324,.T.);
#11011=EDGE_CURVE('',#8592,#8591,#4325,.T.);
#11012=EDGE_CURVE('',#8592,#8593,#4326,.T.);
#11013=EDGE_CURVE('',#8593,#8589,#3645,.T.);
#11014=EDGE_CURVE('',#8593,#8467,#4327,.T.);
#11015=EDGE_CURVE('',#8385,#8592,#4328,.T.);
#11016=EDGE_CURVE('',#8481,#8391,#4329,.T.);
#11017=EDGE_CURVE('',#8591,#8594,#1055,.T.);
#11018=EDGE_CURVE('',#8595,#8594,#3646,.T.);
#11019=EDGE_CURVE('',#8594,#8595,#3647,.T.);
#11020=EDGE_CURVE('',#8514,#8596,#3648,.T.);
#11021=EDGE_CURVE('',#8596,#8597,#4330,.T.);
#11022=EDGE_CURVE('',#8597,#8598,#4331,.T.);
#11023=EDGE_CURVE('',#8598,#8384,#4332,.T.);
#11024=EDGE_CURVE('',#8599,#8598,#4333,.T.);
#11025=EDGE_CURVE('',#8600,#8599,#4334,.T.);
#11026=EDGE_CURVE('',#8478,#8600,#4335,.T.);
#11027=EDGE_CURVE('',#8597,#8601,#4336,.T.);
#11028=EDGE_CURVE('',#8601,#8599,#3649,.T.);
#11029=EDGE_CURVE('',#8601,#8479,#4337,.T.);
#11030=EDGE_CURVE('',#8395,#8596,#4338,.T.);
#11031=EDGE_CURVE('',#8436,#8511,#5352,.T.);
#11032=EDGE_CURVE('',#8602,#8602,#3650,.T.);
#11033=EDGE_CURVE('',#8602,#8595,#5353,.T.);
#11034=EDGE_CURVE('',#8603,#8603,#3651,.T.);
#11035=EDGE_CURVE('',#8603,#8602,#5354,.T.);
#11036=EDGE_CURVE('',#8513,#8603,#5355,.T.);
#15031=ORIENTED_EDGE('',*,*,#10723,.F.);
#15032=ORIENTED_EDGE('',*,*,#10724,.T.);
#15033=ORIENTED_EDGE('',*,*,#10725,.T.);
#15034=ORIENTED_EDGE('',*,*,#10726,.T.);
#15035=ORIENTED_EDGE('',*,*,#10727,.T.);
#15036=ORIENTED_EDGE('',*,*,#10728,.T.);
#15037=ORIENTED_EDGE('',*,*,#10729,.T.);
#15038=ORIENTED_EDGE('',*,*,#10730,.T.);
#15039=ORIENTED_EDGE('',*,*,#10731,.T.);
#15040=ORIENTED_EDGE('',*,*,#10732,.T.);
#15041=ORIENTED_EDGE('',*,*,#10733,.T.);
#15042=ORIENTED_EDGE('',*,*,#10734,.T.);
#15043=ORIENTED_EDGE('',*,*,#10735,.F.);
#15044=ORIENTED_EDGE('',*,*,#10732,.F.);
#15045=ORIENTED_EDGE('',*,*,#10736,.F.);
#15046=ORIENTED_EDGE('',*,*,#10737,.T.);
#15047=ORIENTED_EDGE('',*,*,#10738,.F.);
#15048=ORIENTED_EDGE('',*,*,#10739,.T.);
#15049=ORIENTED_EDGE('',*,*,#10740,.F.);
#15050=ORIENTED_EDGE('',*,*,#10741,.F.);
#15051=ORIENTED_EDGE('',*,*,#10742,.F.);
#15052=ORIENTED_EDGE('',*,*,#10743,.T.);
#15053=ORIENTED_EDGE('',*,*,#10744,.F.);
#15054=ORIENTED_EDGE('',*,*,#10745,.T.);
#15055=ORIENTED_EDGE('',*,*,#10746,.F.);
#15056=ORIENTED_EDGE('',*,*,#10747,.F.);
#15057=ORIENTED_EDGE('',*,*,#10748,.F.);
#15058=ORIENTED_EDGE('',*,*,#10749,.T.);
#15059=ORIENTED_EDGE('',*,*,#10750,.F.);
#15060=ORIENTED_EDGE('',*,*,#10751,.T.);
#15061=ORIENTED_EDGE('',*,*,#10752,.F.);
#15062=ORIENTED_EDGE('',*,*,#10753,.F.);
#15063=ORIENTED_EDGE('',*,*,#10754,.F.);
#15064=ORIENTED_EDGE('',*,*,#10755,.T.);
#15065=ORIENTED_EDGE('',*,*,#10756,.F.);
#15066=ORIENTED_EDGE('',*,*,#10757,.T.);
#15067=ORIENTED_EDGE('',*,*,#10758,.F.);
#15068=ORIENTED_EDGE('',*,*,#10759,.F.);
#15069=ORIENTED_EDGE('',*,*,#10760,.F.);
#15070=ORIENTED_EDGE('',*,*,#10761,.T.);
#15071=ORIENTED_EDGE('',*,*,#10762,.F.);
#15072=ORIENTED_EDGE('',*,*,#10763,.T.);
#15073=ORIENTED_EDGE('',*,*,#10764,.F.);
#15074=ORIENTED_EDGE('',*,*,#10765,.F.);
#15075=ORIENTED_EDGE('',*,*,#10766,.F.);
#15076=ORIENTED_EDGE('',*,*,#10767,.T.);
#15077=ORIENTED_EDGE('',*,*,#10768,.F.);
#15078=ORIENTED_EDGE('',*,*,#10769,.T.);
#15079=ORIENTED_EDGE('',*,*,#10770,.F.);
#15080=ORIENTED_EDGE('',*,*,#10771,.F.);
#15081=ORIENTED_EDGE('',*,*,#10772,.F.);
#15082=ORIENTED_EDGE('',*,*,#10773,.T.);
#15083=ORIENTED_EDGE('',*,*,#10774,.F.);
#15084=ORIENTED_EDGE('',*,*,#10775,.T.);
#15085=ORIENTED_EDGE('',*,*,#10776,.T.);
#15086=ORIENTED_EDGE('',*,*,#10775,.F.);
#15087=ORIENTED_EDGE('',*,*,#10777,.F.);
#15088=ORIENTED_EDGE('',*,*,#10778,.T.);
#15089=ORIENTED_EDGE('',*,*,#10779,.F.);
#15090=ORIENTED_EDGE('',*,*,#10780,.F.);
#15091=ORIENTED_EDGE('',*,*,#10781,.F.);
#15092=ORIENTED_EDGE('',*,*,#10782,.T.);
#15093=ORIENTED_EDGE('',*,*,#10783,.F.);
#15094=ORIENTED_EDGE('',*,*,#10784,.T.);
#15095=ORIENTED_EDGE('',*,*,#10785,.F.);
#15096=ORIENTED_EDGE('',*,*,#10786,.F.);
#15097=ORIENTED_EDGE('',*,*,#10787,.F.);
#15098=ORIENTED_EDGE('',*,*,#10788,.T.);
#15099=ORIENTED_EDGE('',*,*,#10789,.F.);
#15100=ORIENTED_EDGE('',*,*,#10790,.T.);
#15101=ORIENTED_EDGE('',*,*,#10791,.F.);
#15102=ORIENTED_EDGE('',*,*,#10792,.F.);
#15103=ORIENTED_EDGE('',*,*,#10793,.F.);
#15104=ORIENTED_EDGE('',*,*,#10794,.T.);
#15105=ORIENTED_EDGE('',*,*,#10795,.F.);
#15106=ORIENTED_EDGE('',*,*,#10796,.T.);
#15107=ORIENTED_EDGE('',*,*,#10797,.F.);
#15108=ORIENTED_EDGE('',*,*,#10798,.F.);
#15109=ORIENTED_EDGE('',*,*,#10799,.F.);
#15110=ORIENTED_EDGE('',*,*,#10800,.T.);
#15111=ORIENTED_EDGE('',*,*,#10801,.F.);
#15112=ORIENTED_EDGE('',*,*,#10802,.T.);
#15113=ORIENTED_EDGE('',*,*,#10803,.F.);
#15114=ORIENTED_EDGE('',*,*,#10804,.F.);
#15115=ORIENTED_EDGE('',*,*,#10805,.F.);
#15116=ORIENTED_EDGE('',*,*,#10806,.T.);
#15117=ORIENTED_EDGE('',*,*,#10807,.F.);
#15118=ORIENTED_EDGE('',*,*,#10808,.T.);
#15119=ORIENTED_EDGE('',*,*,#10809,.F.);
#15120=ORIENTED_EDGE('',*,*,#10810,.F.);
#15121=ORIENTED_EDGE('',*,*,#10811,.F.);
#15122=ORIENTED_EDGE('',*,*,#10812,.T.);
#15123=ORIENTED_EDGE('',*,*,#10813,.F.);
#15124=ORIENTED_EDGE('',*,*,#10814,.T.);
#15125=ORIENTED_EDGE('',*,*,#10815,.F.);
#15126=ORIENTED_EDGE('',*,*,#10816,.F.);
#15127=ORIENTED_EDGE('',*,*,#10817,.F.);
#15128=ORIENTED_EDGE('',*,*,#10818,.T.);
#15129=ORIENTED_EDGE('',*,*,#10819,.F.);
#15130=ORIENTED_EDGE('',*,*,#10820,.T.);
#15131=ORIENTED_EDGE('',*,*,#10821,.T.);
#15132=ORIENTED_EDGE('',*,*,#10810,.T.);
#15133=ORIENTED_EDGE('',*,*,#10822,.T.);
#15134=ORIENTED_EDGE('',*,*,#10823,.T.);
#15135=ORIENTED_EDGE('',*,*,#10824,.T.);
#15136=ORIENTED_EDGE('',*,*,#10798,.T.);
#15137=ORIENTED_EDGE('',*,*,#10825,.T.);
#15138=ORIENTED_EDGE('',*,*,#10826,.T.);
#15139=ORIENTED_EDGE('',*,*,#10827,.T.);
#15140=ORIENTED_EDGE('',*,*,#10786,.T.);
#15141=ORIENTED_EDGE('',*,*,#10828,.T.);
#15142=ORIENTED_EDGE('',*,*,#10829,.T.);
#15143=ORIENTED_EDGE('',*,*,#10830,.T.);
#15144=ORIENTED_EDGE('',*,*,#10771,.T.);
#15145=ORIENTED_EDGE('',*,*,#10831,.T.);
#15146=ORIENTED_EDGE('',*,*,#10832,.T.);
#15147=ORIENTED_EDGE('',*,*,#10833,.T.);
#15148=ORIENTED_EDGE('',*,*,#10759,.T.);
#15149=ORIENTED_EDGE('',*,*,#10834,.T.);
#15150=ORIENTED_EDGE('',*,*,#10835,.T.);
#15151=ORIENTED_EDGE('',*,*,#10836,.T.);
#15152=ORIENTED_EDGE('',*,*,#10747,.T.);
#15153=ORIENTED_EDGE('',*,*,#10837,.T.);
#15154=ORIENTED_EDGE('',*,*,#10838,.T.);
#15155=ORIENTED_EDGE('',*,*,#10839,.T.);
#15156=ORIENTED_EDGE('',*,*,#10816,.T.);
#15157=ORIENTED_EDGE('',*,*,#10840,.T.);
#15158=ORIENTED_EDGE('',*,*,#10841,.T.);
#15159=ORIENTED_EDGE('',*,*,#10842,.T.);
#15160=ORIENTED_EDGE('',*,*,#10804,.T.);
#15161=ORIENTED_EDGE('',*,*,#10843,.T.);
#15162=ORIENTED_EDGE('',*,*,#10844,.T.);
#15163=ORIENTED_EDGE('',*,*,#10845,.T.);
#15164=ORIENTED_EDGE('',*,*,#10792,.T.);
#15165=ORIENTED_EDGE('',*,*,#10846,.T.);
#15166=ORIENTED_EDGE('',*,*,#10847,.T.);
#15167=ORIENTED_EDGE('',*,*,#10848,.T.);
#15168=ORIENTED_EDGE('',*,*,#10780,.T.);
#15169=ORIENTED_EDGE('',*,*,#10849,.T.);
#15170=ORIENTED_EDGE('',*,*,#10850,.T.);
#15171=ORIENTED_EDGE('',*,*,#10851,.T.);
#15172=ORIENTED_EDGE('',*,*,#10765,.T.);
#15173=ORIENTED_EDGE('',*,*,#10852,.T.);
#15174=ORIENTED_EDGE('',*,*,#10853,.T.);
#15175=ORIENTED_EDGE('',*,*,#10854,.T.);
#15176=ORIENTED_EDGE('',*,*,#10753,.T.);
#15177=ORIENTED_EDGE('',*,*,#10855,.T.);
#15178=ORIENTED_EDGE('',*,*,#10856,.T.);
#15179=ORIENTED_EDGE('',*,*,#10857,.T.);
#15180=ORIENTED_EDGE('',*,*,#10741,.T.);
#15181=ORIENTED_EDGE('',*,*,#10858,.T.);
#15182=ORIENTED_EDGE('',*,*,#10859,.T.);
#15183=ORIENTED_EDGE('',*,*,#10860,.T.);
#15184=ORIENTED_EDGE('',*,*,#10861,.T.);
#15185=ORIENTED_EDGE('',*,*,#10862,.T.);
#15186=ORIENTED_EDGE('',*,*,#10863,.T.);
#15187=ORIENTED_EDGE('',*,*,#10861,.F.);
#15188=ORIENTED_EDGE('',*,*,#10864,.F.);
#15189=ORIENTED_EDGE('',*,*,#10865,.F.);
#15190=ORIENTED_EDGE('',*,*,#10866,.T.);
#15191=ORIENTED_EDGE('',*,*,#10862,.F.);
#15192=ORIENTED_EDGE('',*,*,#10863,.F.);
#15193=ORIENTED_EDGE('',*,*,#10866,.F.);
#15194=ORIENTED_EDGE('',*,*,#10867,.F.);
#15195=ORIENTED_EDGE('',*,*,#10860,.F.);
#15196=ORIENTED_EDGE('',*,*,#10864,.T.);
#15197=ORIENTED_EDGE('',*,*,#10865,.T.);
#15198=ORIENTED_EDGE('',*,*,#10868,.T.);
#15199=ORIENTED_EDGE('',*,*,#10869,.T.);
#15200=ORIENTED_EDGE('',*,*,#10868,.F.);
#15201=ORIENTED_EDGE('',*,*,#10870,.T.);
#15202=ORIENTED_EDGE('',*,*,#10869,.F.);
#15203=ORIENTED_EDGE('',*,*,#10871,.F.);
#15204=ORIENTED_EDGE('',*,*,#10872,.F.);
#15205=ORIENTED_EDGE('',*,*,#10873,.F.);
#15206=ORIENTED_EDGE('',*,*,#10874,.F.);
#15207=ORIENTED_EDGE('',*,*,#10737,.F.);
#15208=ORIENTED_EDGE('',*,*,#10736,.T.);
#15209=ORIENTED_EDGE('',*,*,#10731,.F.);
#15210=ORIENTED_EDGE('',*,*,#10875,.F.);
#15211=ORIENTED_EDGE('',*,*,#10876,.T.);
#15212=ORIENTED_EDGE('',*,*,#10877,.T.);
#15213=ORIENTED_EDGE('',*,*,#10873,.T.);
#15214=ORIENTED_EDGE('',*,*,#10878,.T.);
#15215=ORIENTED_EDGE('',*,*,#10738,.T.);
#15216=ORIENTED_EDGE('',*,*,#10874,.T.);
#15217=ORIENTED_EDGE('',*,*,#10877,.F.);
#15218=ORIENTED_EDGE('',*,*,#10739,.F.);
#15219=ORIENTED_EDGE('',*,*,#10878,.F.);
#15220=ORIENTED_EDGE('',*,*,#10876,.F.);
#15221=ORIENTED_EDGE('',*,*,#10879,.F.);
#15222=ORIENTED_EDGE('',*,*,#10880,.F.);
#15223=ORIENTED_EDGE('',*,*,#10858,.F.);
#15224=ORIENTED_EDGE('',*,*,#10740,.T.);
#15225=ORIENTED_EDGE('',*,*,#10859,.F.);
#15226=ORIENTED_EDGE('',*,*,#10880,.T.);
#15227=ORIENTED_EDGE('',*,*,#10881,.F.);
#15228=ORIENTED_EDGE('',*,*,#10882,.T.);
#15229=ORIENTED_EDGE('',*,*,#10883,.F.);
#15230=ORIENTED_EDGE('',*,*,#10884,.F.);
#15231=ORIENTED_EDGE('',*,*,#10885,.F.);
#15232=ORIENTED_EDGE('',*,*,#10886,.F.);
#15233=ORIENTED_EDGE('',*,*,#10749,.F.);
#15234=ORIENTED_EDGE('',*,*,#10748,.T.);
#15235=ORIENTED_EDGE('',*,*,#10836,.F.);
#15236=ORIENTED_EDGE('',*,*,#10887,.F.);
#15237=ORIENTED_EDGE('',*,*,#10888,.T.);
#15238=ORIENTED_EDGE('',*,*,#10889,.T.);
#15239=ORIENTED_EDGE('',*,*,#10885,.T.);
#15240=ORIENTED_EDGE('',*,*,#10890,.T.);
#15241=ORIENTED_EDGE('',*,*,#10750,.T.);
#15242=ORIENTED_EDGE('',*,*,#10886,.T.);
#15243=ORIENTED_EDGE('',*,*,#10889,.F.);
#15244=ORIENTED_EDGE('',*,*,#10751,.F.);
#15245=ORIENTED_EDGE('',*,*,#10890,.F.);
#15246=ORIENTED_EDGE('',*,*,#10888,.F.);
#15247=ORIENTED_EDGE('',*,*,#10891,.F.);
#15248=ORIENTED_EDGE('',*,*,#10892,.F.);
#15249=ORIENTED_EDGE('',*,*,#10855,.F.);
#15250=ORIENTED_EDGE('',*,*,#10752,.T.);
#15251=ORIENTED_EDGE('',*,*,#10856,.F.);
#15252=ORIENTED_EDGE('',*,*,#10892,.T.);
#15253=ORIENTED_EDGE('',*,*,#10893,.F.);
#15254=ORIENTED_EDGE('',*,*,#10894,.T.);
#15255=ORIENTED_EDGE('',*,*,#10895,.F.);
#15256=ORIENTED_EDGE('',*,*,#10896,.F.);
#15257=ORIENTED_EDGE('',*,*,#10897,.F.);
#15258=ORIENTED_EDGE('',*,*,#10898,.F.);
#15259=ORIENTED_EDGE('',*,*,#10761,.F.);
#15260=ORIENTED_EDGE('',*,*,#10760,.T.);
#15261=ORIENTED_EDGE('',*,*,#10833,.F.);
#15262=ORIENTED_EDGE('',*,*,#10899,.F.);
#15263=ORIENTED_EDGE('',*,*,#10900,.T.);
#15264=ORIENTED_EDGE('',*,*,#10901,.T.);
#15265=ORIENTED_EDGE('',*,*,#10897,.T.);
#15266=ORIENTED_EDGE('',*,*,#10902,.T.);
#15267=ORIENTED_EDGE('',*,*,#10762,.T.);
#15268=ORIENTED_EDGE('',*,*,#10898,.T.);
#15269=ORIENTED_EDGE('',*,*,#10901,.F.);
#15270=ORIENTED_EDGE('',*,*,#10763,.F.);
#15271=ORIENTED_EDGE('',*,*,#10902,.F.);
#15272=ORIENTED_EDGE('',*,*,#10900,.F.);
#15273=ORIENTED_EDGE('',*,*,#10903,.F.);
#15274=ORIENTED_EDGE('',*,*,#10904,.F.);
#15275=ORIENTED_EDGE('',*,*,#10852,.F.);
#15276=ORIENTED_EDGE('',*,*,#10764,.T.);
#15277=ORIENTED_EDGE('',*,*,#10853,.F.);
#15278=ORIENTED_EDGE('',*,*,#10904,.T.);
#15279=ORIENTED_EDGE('',*,*,#10905,.F.);
#15280=ORIENTED_EDGE('',*,*,#10906,.T.);
#15281=ORIENTED_EDGE('',*,*,#10907,.F.);
#15282=ORIENTED_EDGE('',*,*,#10908,.F.);
#15283=ORIENTED_EDGE('',*,*,#10909,.F.);
#15284=ORIENTED_EDGE('',*,*,#10910,.F.);
#15285=ORIENTED_EDGE('',*,*,#10773,.F.);
#15286=ORIENTED_EDGE('',*,*,#10772,.T.);
#15287=ORIENTED_EDGE('',*,*,#10830,.F.);
#15288=ORIENTED_EDGE('',*,*,#10911,.F.);
#15289=ORIENTED_EDGE('',*,*,#10912,.T.);
#15290=ORIENTED_EDGE('',*,*,#10913,.T.);
#15291=ORIENTED_EDGE('',*,*,#10909,.T.);
#15292=ORIENTED_EDGE('',*,*,#10914,.T.);
#15293=ORIENTED_EDGE('',*,*,#10777,.T.);
#15294=ORIENTED_EDGE('',*,*,#10774,.T.);
#15295=ORIENTED_EDGE('',*,*,#10910,.T.);
#15296=ORIENTED_EDGE('',*,*,#10913,.F.);
#15297=ORIENTED_EDGE('',*,*,#10778,.F.);
#15298=ORIENTED_EDGE('',*,*,#10914,.F.);
#15299=ORIENTED_EDGE('',*,*,#10912,.F.);
#15300=ORIENTED_EDGE('',*,*,#10915,.F.);
#15301=ORIENTED_EDGE('',*,*,#10916,.F.);
#15302=ORIENTED_EDGE('',*,*,#10849,.F.);
#15303=ORIENTED_EDGE('',*,*,#10779,.T.);
#15304=ORIENTED_EDGE('',*,*,#10850,.F.);
#15305=ORIENTED_EDGE('',*,*,#10916,.T.);
#15306=ORIENTED_EDGE('',*,*,#10917,.F.);
#15307=ORIENTED_EDGE('',*,*,#10918,.T.);
#15308=ORIENTED_EDGE('',*,*,#10919,.F.);
#15309=ORIENTED_EDGE('',*,*,#10920,.F.);
#15310=ORIENTED_EDGE('',*,*,#10921,.F.);
#15311=ORIENTED_EDGE('',*,*,#10922,.F.);
#15312=ORIENTED_EDGE('',*,*,#10788,.F.);
#15313=ORIENTED_EDGE('',*,*,#10787,.T.);
#15314=ORIENTED_EDGE('',*,*,#10827,.F.);
#15315=ORIENTED_EDGE('',*,*,#10923,.F.);
#15316=ORIENTED_EDGE('',*,*,#10924,.T.);
#15317=ORIENTED_EDGE('',*,*,#10925,.T.);
#15318=ORIENTED_EDGE('',*,*,#10921,.T.);
#15319=ORIENTED_EDGE('',*,*,#10926,.T.);
#15320=ORIENTED_EDGE('',*,*,#10789,.T.);
#15321=ORIENTED_EDGE('',*,*,#10922,.T.);
#15322=ORIENTED_EDGE('',*,*,#10925,.F.);
#15323=ORIENTED_EDGE('',*,*,#10790,.F.);
#15324=ORIENTED_EDGE('',*,*,#10926,.F.);
#15325=ORIENTED_EDGE('',*,*,#10924,.F.);
#15326=ORIENTED_EDGE('',*,*,#10927,.F.);
#15327=ORIENTED_EDGE('',*,*,#10928,.F.);
#15328=ORIENTED_EDGE('',*,*,#10846,.F.);
#15329=ORIENTED_EDGE('',*,*,#10791,.T.);
#15330=ORIENTED_EDGE('',*,*,#10847,.F.);
#15331=ORIENTED_EDGE('',*,*,#10928,.T.);
#15332=ORIENTED_EDGE('',*,*,#10929,.F.);
#15333=ORIENTED_EDGE('',*,*,#10930,.T.);
#15334=ORIENTED_EDGE('',*,*,#10931,.F.);
#15335=ORIENTED_EDGE('',*,*,#10932,.F.);
#15336=ORIENTED_EDGE('',*,*,#10933,.F.);
#15337=ORIENTED_EDGE('',*,*,#10934,.F.);
#15338=ORIENTED_EDGE('',*,*,#10800,.F.);
#15339=ORIENTED_EDGE('',*,*,#10799,.T.);
#15340=ORIENTED_EDGE('',*,*,#10824,.F.);
#15341=ORIENTED_EDGE('',*,*,#10935,.F.);
#15342=ORIENTED_EDGE('',*,*,#10936,.T.);
#15343=ORIENTED_EDGE('',*,*,#10937,.T.);
#15344=ORIENTED_EDGE('',*,*,#10933,.T.);
#15345=ORIENTED_EDGE('',*,*,#10938,.T.);
#15346=ORIENTED_EDGE('',*,*,#10801,.T.);
#15347=ORIENTED_EDGE('',*,*,#10934,.T.);
#15348=ORIENTED_EDGE('',*,*,#10937,.F.);
#15349=ORIENTED_EDGE('',*,*,#10802,.F.);
#15350=ORIENTED_EDGE('',*,*,#10938,.F.);
#15351=ORIENTED_EDGE('',*,*,#10936,.F.);
#15352=ORIENTED_EDGE('',*,*,#10939,.F.);
#15353=ORIENTED_EDGE('',*,*,#10940,.F.);
#15354=ORIENTED_EDGE('',*,*,#10843,.F.);
#15355=ORIENTED_EDGE('',*,*,#10803,.T.);
#15356=ORIENTED_EDGE('',*,*,#10844,.F.);
#15357=ORIENTED_EDGE('',*,*,#10940,.T.);
#15358=ORIENTED_EDGE('',*,*,#10941,.F.);
#15359=ORIENTED_EDGE('',*,*,#10942,.T.);
#15360=ORIENTED_EDGE('',*,*,#10943,.F.);
#15361=ORIENTED_EDGE('',*,*,#10728,.F.);
#15362=ORIENTED_EDGE('',*,*,#10944,.F.);
#15363=ORIENTED_EDGE('',*,*,#10945,.F.);
#15364=ORIENTED_EDGE('',*,*,#10812,.F.);
#15365=ORIENTED_EDGE('',*,*,#10811,.T.);
#15366=ORIENTED_EDGE('',*,*,#10821,.F.);
#15367=ORIENTED_EDGE('',*,*,#10727,.F.);
#15368=ORIENTED_EDGE('',*,*,#10946,.T.);
#15369=ORIENTED_EDGE('',*,*,#10947,.T.);
#15370=ORIENTED_EDGE('',*,*,#10944,.T.);
#15371=ORIENTED_EDGE('',*,*,#10948,.T.);
#15372=ORIENTED_EDGE('',*,*,#10813,.T.);
#15373=ORIENTED_EDGE('',*,*,#10945,.T.);
#15374=ORIENTED_EDGE('',*,*,#10947,.F.);
#15375=ORIENTED_EDGE('',*,*,#10814,.F.);
#15376=ORIENTED_EDGE('',*,*,#10948,.F.);
#15377=ORIENTED_EDGE('',*,*,#10946,.F.);
#15378=ORIENTED_EDGE('',*,*,#10726,.F.);
#15379=ORIENTED_EDGE('',*,*,#10949,.F.);
#15380=ORIENTED_EDGE('',*,*,#10840,.F.);
#15381=ORIENTED_EDGE('',*,*,#10815,.T.);
#15382=ORIENTED_EDGE('',*,*,#10841,.F.);
#15383=ORIENTED_EDGE('',*,*,#10949,.T.);
#15384=ORIENTED_EDGE('',*,*,#10725,.F.);
#15385=ORIENTED_EDGE('',*,*,#10950,.T.);
#15386=ORIENTED_EDGE('',*,*,#10882,.F.);
#15387=ORIENTED_EDGE('',*,*,#10951,.F.);
#15388=ORIENTED_EDGE('',*,*,#10952,.F.);
#15389=ORIENTED_EDGE('',*,*,#10953,.F.);
#15390=ORIENTED_EDGE('',*,*,#10954,.F.);
#15391=ORIENTED_EDGE('',*,*,#10743,.F.);
#15392=ORIENTED_EDGE('',*,*,#10742,.T.);
#15393=ORIENTED_EDGE('',*,*,#10857,.F.);
#15394=ORIENTED_EDGE('',*,*,#10955,.F.);
#15395=ORIENTED_EDGE('',*,*,#10956,.T.);
#15396=ORIENTED_EDGE('',*,*,#10957,.T.);
#15397=ORIENTED_EDGE('',*,*,#10952,.T.);
#15398=ORIENTED_EDGE('',*,*,#10954,.T.);
#15399=ORIENTED_EDGE('',*,*,#10953,.T.);
#15400=ORIENTED_EDGE('',*,*,#10957,.F.);
#15401=ORIENTED_EDGE('',*,*,#10958,.T.);
#15402=ORIENTED_EDGE('',*,*,#10744,.T.);
#15403=ORIENTED_EDGE('',*,*,#10745,.F.);
#15404=ORIENTED_EDGE('',*,*,#10958,.F.);
#15405=ORIENTED_EDGE('',*,*,#10956,.F.);
#15406=ORIENTED_EDGE('',*,*,#10959,.F.);
#15407=ORIENTED_EDGE('',*,*,#10960,.F.);
#15408=ORIENTED_EDGE('',*,*,#10837,.F.);
#15409=ORIENTED_EDGE('',*,*,#10746,.T.);
#15410=ORIENTED_EDGE('',*,*,#10838,.F.);
#15411=ORIENTED_EDGE('',*,*,#10960,.T.);
#15412=ORIENTED_EDGE('',*,*,#10961,.F.);
#15413=ORIENTED_EDGE('',*,*,#10883,.T.);
#15414=ORIENTED_EDGE('',*,*,#10894,.F.);
#15415=ORIENTED_EDGE('',*,*,#10962,.F.);
#15416=ORIENTED_EDGE('',*,*,#10963,.F.);
#15417=ORIENTED_EDGE('',*,*,#10964,.F.);
#15418=ORIENTED_EDGE('',*,*,#10965,.F.);
#15419=ORIENTED_EDGE('',*,*,#10755,.F.);
#15420=ORIENTED_EDGE('',*,*,#10754,.T.);
#15421=ORIENTED_EDGE('',*,*,#10854,.F.);
#15422=ORIENTED_EDGE('',*,*,#10966,.F.);
#15423=ORIENTED_EDGE('',*,*,#10967,.T.);
#15424=ORIENTED_EDGE('',*,*,#10968,.T.);
#15425=ORIENTED_EDGE('',*,*,#10963,.T.);
#15426=ORIENTED_EDGE('',*,*,#10965,.T.);
#15427=ORIENTED_EDGE('',*,*,#10964,.T.);
#15428=ORIENTED_EDGE('',*,*,#10968,.F.);
#15429=ORIENTED_EDGE('',*,*,#10969,.T.);
#15430=ORIENTED_EDGE('',*,*,#10756,.T.);
#15431=ORIENTED_EDGE('',*,*,#10757,.F.);
#15432=ORIENTED_EDGE('',*,*,#10969,.F.);
#15433=ORIENTED_EDGE('',*,*,#10967,.F.);
#15434=ORIENTED_EDGE('',*,*,#10970,.F.);
#15435=ORIENTED_EDGE('',*,*,#10971,.F.);
#15436=ORIENTED_EDGE('',*,*,#10834,.F.);
#15437=ORIENTED_EDGE('',*,*,#10758,.T.);
#15438=ORIENTED_EDGE('',*,*,#10835,.F.);
#15439=ORIENTED_EDGE('',*,*,#10971,.T.);
#15440=ORIENTED_EDGE('',*,*,#10972,.F.);
#15441=ORIENTED_EDGE('',*,*,#10895,.T.);
#15442=ORIENTED_EDGE('',*,*,#10906,.F.);
#15443=ORIENTED_EDGE('',*,*,#10973,.F.);
#15444=ORIENTED_EDGE('',*,*,#10974,.F.);
#15445=ORIENTED_EDGE('',*,*,#10975,.F.);
#15446=ORIENTED_EDGE('',*,*,#10976,.F.);
#15447=ORIENTED_EDGE('',*,*,#10767,.F.);
#15448=ORIENTED_EDGE('',*,*,#10766,.T.);
#15449=ORIENTED_EDGE('',*,*,#10851,.F.);
#15450=ORIENTED_EDGE('',*,*,#10977,.F.);
#15451=ORIENTED_EDGE('',*,*,#10978,.T.);
#15452=ORIENTED_EDGE('',*,*,#10979,.T.);
#15453=ORIENTED_EDGE('',*,*,#10974,.T.);
#15454=ORIENTED_EDGE('',*,*,#10976,.T.);
#15455=ORIENTED_EDGE('',*,*,#10975,.T.);
#15456=ORIENTED_EDGE('',*,*,#10979,.F.);
#15457=ORIENTED_EDGE('',*,*,#10980,.T.);
#15458=ORIENTED_EDGE('',*,*,#10768,.T.);
#15459=ORIENTED_EDGE('',*,*,#10769,.F.);
#15460=ORIENTED_EDGE('',*,*,#10980,.F.);
#15461=ORIENTED_EDGE('',*,*,#10978,.F.);
#15462=ORIENTED_EDGE('',*,*,#10981,.F.);
#15463=ORIENTED_EDGE('',*,*,#10982,.F.);
#15464=ORIENTED_EDGE('',*,*,#10831,.F.);
#15465=ORIENTED_EDGE('',*,*,#10770,.T.);
#15466=ORIENTED_EDGE('',*,*,#10832,.F.);
#15467=ORIENTED_EDGE('',*,*,#10982,.T.);
#15468=ORIENTED_EDGE('',*,*,#10983,.F.);
#15469=ORIENTED_EDGE('',*,*,#10907,.T.);
#15470=ORIENTED_EDGE('',*,*,#10918,.F.);
#15471=ORIENTED_EDGE('',*,*,#10984,.F.);
#15472=ORIENTED_EDGE('',*,*,#10985,.F.);
#15473=ORIENTED_EDGE('',*,*,#10986,.F.);
#15474=ORIENTED_EDGE('',*,*,#10987,.F.);
#15475=ORIENTED_EDGE('',*,*,#10782,.F.);
#15476=ORIENTED_EDGE('',*,*,#10781,.T.);
#15477=ORIENTED_EDGE('',*,*,#10848,.F.);
#15478=ORIENTED_EDGE('',*,*,#10988,.F.);
#15479=ORIENTED_EDGE('',*,*,#10989,.T.);
#15480=ORIENTED_EDGE('',*,*,#10990,.T.);
#15481=ORIENTED_EDGE('',*,*,#10985,.T.);
#15482=ORIENTED_EDGE('',*,*,#10987,.T.);
#15483=ORIENTED_EDGE('',*,*,#10986,.T.);
#15484=ORIENTED_EDGE('',*,*,#10990,.F.);
#15485=ORIENTED_EDGE('',*,*,#10991,.T.);
#15486=ORIENTED_EDGE('',*,*,#10783,.T.);
#15487=ORIENTED_EDGE('',*,*,#10784,.F.);
#15488=ORIENTED_EDGE('',*,*,#10991,.F.);
#15489=ORIENTED_EDGE('',*,*,#10989,.F.);
#15490=ORIENTED_EDGE('',*,*,#10992,.F.);
#15491=ORIENTED_EDGE('',*,*,#10993,.F.);
#15492=ORIENTED_EDGE('',*,*,#10828,.F.);
#15493=ORIENTED_EDGE('',*,*,#10785,.T.);
#15494=ORIENTED_EDGE('',*,*,#10829,.F.);
#15495=ORIENTED_EDGE('',*,*,#10993,.T.);
#15496=ORIENTED_EDGE('',*,*,#10994,.F.);
#15497=ORIENTED_EDGE('',*,*,#10919,.T.);
#15498=ORIENTED_EDGE('',*,*,#10930,.F.);
#15499=ORIENTED_EDGE('',*,*,#10995,.F.);
#15500=ORIENTED_EDGE('',*,*,#10996,.F.);
#15501=ORIENTED_EDGE('',*,*,#10997,.F.);
#15502=ORIENTED_EDGE('',*,*,#10998,.F.);
#15503=ORIENTED_EDGE('',*,*,#10794,.F.);
#15504=ORIENTED_EDGE('',*,*,#10793,.T.);
#15505=ORIENTED_EDGE('',*,*,#10845,.F.);
#15506=ORIENTED_EDGE('',*,*,#10999,.F.);
#15507=ORIENTED_EDGE('',*,*,#11000,.T.);
#15508=ORIENTED_EDGE('',*,*,#11001,.T.);
#15509=ORIENTED_EDGE('',*,*,#10996,.T.);
#15510=ORIENTED_EDGE('',*,*,#10998,.T.);
#15511=ORIENTED_EDGE('',*,*,#10997,.T.);
#15512=ORIENTED_EDGE('',*,*,#11001,.F.);
#15513=ORIENTED_EDGE('',*,*,#11002,.T.);
#15514=ORIENTED_EDGE('',*,*,#10795,.T.);
#15515=ORIENTED_EDGE('',*,*,#10796,.F.);
#15516=ORIENTED_EDGE('',*,*,#11002,.F.);
#15517=ORIENTED_EDGE('',*,*,#11000,.F.);
#15518=ORIENTED_EDGE('',*,*,#11003,.F.);
#15519=ORIENTED_EDGE('',*,*,#11004,.F.);
#15520=ORIENTED_EDGE('',*,*,#10825,.F.);
#15521=ORIENTED_EDGE('',*,*,#10797,.T.);
#15522=ORIENTED_EDGE('',*,*,#10826,.F.);
#15523=ORIENTED_EDGE('',*,*,#11004,.T.);
#15524=ORIENTED_EDGE('',*,*,#11005,.F.);
#15525=ORIENTED_EDGE('',*,*,#10931,.T.);
#15526=ORIENTED_EDGE('',*,*,#10942,.F.);
#15527=ORIENTED_EDGE('',*,*,#11006,.F.);
#15528=ORIENTED_EDGE('',*,*,#11007,.F.);
#15529=ORIENTED_EDGE('',*,*,#11008,.F.);
#15530=ORIENTED_EDGE('',*,*,#11009,.F.);
#15531=ORIENTED_EDGE('',*,*,#10806,.F.);
#15532=ORIENTED_EDGE('',*,*,#10805,.T.);
#15533=ORIENTED_EDGE('',*,*,#10842,.F.);
#15534=ORIENTED_EDGE('',*,*,#11010,.F.);
#15535=ORIENTED_EDGE('',*,*,#11011,.F.);
#15536=ORIENTED_EDGE('',*,*,#11012,.T.);
#15537=ORIENTED_EDGE('',*,*,#11013,.T.);
#15538=ORIENTED_EDGE('',*,*,#11007,.T.);
#15539=ORIENTED_EDGE('',*,*,#11009,.T.);
#15540=ORIENTED_EDGE('',*,*,#11008,.T.);
#15541=ORIENTED_EDGE('',*,*,#11013,.F.);
#15542=ORIENTED_EDGE('',*,*,#11014,.T.);
#15543=ORIENTED_EDGE('',*,*,#10807,.T.);
#15544=ORIENTED_EDGE('',*,*,#10808,.F.);
#15545=ORIENTED_EDGE('',*,*,#11014,.F.);
#15546=ORIENTED_EDGE('',*,*,#11012,.F.);
#15547=ORIENTED_EDGE('',*,*,#11015,.F.);
#15548=ORIENTED_EDGE('',*,*,#10730,.F.);
#15549=ORIENTED_EDGE('',*,*,#11016,.F.);
#15550=ORIENTED_EDGE('',*,*,#10822,.F.);
#15551=ORIENTED_EDGE('',*,*,#10809,.T.);
#15552=ORIENTED_EDGE('',*,*,#10823,.F.);
#15553=ORIENTED_EDGE('',*,*,#11016,.T.);
#15554=ORIENTED_EDGE('',*,*,#10729,.F.);
#15555=ORIENTED_EDGE('',*,*,#10943,.T.);
#15556=ORIENTED_EDGE('',*,*,#10723,.T.);
#15557=ORIENTED_EDGE('',*,*,#11015,.T.);
#15558=ORIENTED_EDGE('',*,*,#11011,.T.);
#15559=ORIENTED_EDGE('',*,*,#11017,.T.);
#15560=ORIENTED_EDGE('',*,*,#11018,.F.);
#15561=ORIENTED_EDGE('',*,*,#11019,.F.);
#15562=ORIENTED_EDGE('',*,*,#11017,.F.);
#15563=ORIENTED_EDGE('',*,*,#11010,.T.);
#15564=ORIENTED_EDGE('',*,*,#11006,.T.);
#15565=ORIENTED_EDGE('',*,*,#10941,.T.);
#15566=ORIENTED_EDGE('',*,*,#10939,.T.);
#15567=ORIENTED_EDGE('',*,*,#10935,.T.);
#15568=ORIENTED_EDGE('',*,*,#10932,.T.);
#15569=ORIENTED_EDGE('',*,*,#11005,.T.);
#15570=ORIENTED_EDGE('',*,*,#11003,.T.);
#15571=ORIENTED_EDGE('',*,*,#10999,.T.);
#15572=ORIENTED_EDGE('',*,*,#10995,.T.);
#15573=ORIENTED_EDGE('',*,*,#10929,.T.);
#15574=ORIENTED_EDGE('',*,*,#10927,.T.);
#15575=ORIENTED_EDGE('',*,*,#10923,.T.);
#15576=ORIENTED_EDGE('',*,*,#10920,.T.);
#15577=ORIENTED_EDGE('',*,*,#10994,.T.);
#15578=ORIENTED_EDGE('',*,*,#10992,.T.);
#15579=ORIENTED_EDGE('',*,*,#10988,.T.);
#15580=ORIENTED_EDGE('',*,*,#10984,.T.);
#15581=ORIENTED_EDGE('',*,*,#10917,.T.);
#15582=ORIENTED_EDGE('',*,*,#10915,.T.);
#15583=ORIENTED_EDGE('',*,*,#10911,.T.);
#15584=ORIENTED_EDGE('',*,*,#10908,.T.);
#15585=ORIENTED_EDGE('',*,*,#10983,.T.);
#15586=ORIENTED_EDGE('',*,*,#10981,.T.);
#15587=ORIENTED_EDGE('',*,*,#10977,.T.);
#15588=ORIENTED_EDGE('',*,*,#10973,.T.);
#15589=ORIENTED_EDGE('',*,*,#10905,.T.);
#15590=ORIENTED_EDGE('',*,*,#10903,.T.);
#15591=ORIENTED_EDGE('',*,*,#10899,.T.);
#15592=ORIENTED_EDGE('',*,*,#10896,.T.);
#15593=ORIENTED_EDGE('',*,*,#10972,.T.);
#15594=ORIENTED_EDGE('',*,*,#10970,.T.);
#15595=ORIENTED_EDGE('',*,*,#10966,.T.);
#15596=ORIENTED_EDGE('',*,*,#10962,.T.);
#15597=ORIENTED_EDGE('',*,*,#10893,.T.);
#15598=ORIENTED_EDGE('',*,*,#10891,.T.);
#15599=ORIENTED_EDGE('',*,*,#10887,.T.);
#15600=ORIENTED_EDGE('',*,*,#10884,.T.);
#15601=ORIENTED_EDGE('',*,*,#10961,.T.);
#15602=ORIENTED_EDGE('',*,*,#10959,.T.);
#15603=ORIENTED_EDGE('',*,*,#10955,.T.);
#15604=ORIENTED_EDGE('',*,*,#10951,.T.);
#15605=ORIENTED_EDGE('',*,*,#10881,.T.);
#15606=ORIENTED_EDGE('',*,*,#10879,.T.);
#15607=ORIENTED_EDGE('',*,*,#10875,.T.);
#15608=ORIENTED_EDGE('',*,*,#10872,.T.);
#15609=ORIENTED_EDGE('',*,*,#11020,.T.);
#15610=ORIENTED_EDGE('',*,*,#11021,.T.);
#15611=ORIENTED_EDGE('',*,*,#11022,.T.);
#15612=ORIENTED_EDGE('',*,*,#11023,.T.);
#15613=ORIENTED_EDGE('',*,*,#10950,.F.);
#15614=ORIENTED_EDGE('',*,*,#10724,.F.);
#15615=ORIENTED_EDGE('',*,*,#11023,.F.);
#15616=ORIENTED_EDGE('',*,*,#11024,.F.);
#15617=ORIENTED_EDGE('',*,*,#11025,.F.);
#15618=ORIENTED_EDGE('',*,*,#11026,.F.);
#15619=ORIENTED_EDGE('',*,*,#10818,.F.);
#15620=ORIENTED_EDGE('',*,*,#10817,.T.);
#15621=ORIENTED_EDGE('',*,*,#10839,.F.);
#15622=ORIENTED_EDGE('',*,*,#11022,.F.);
#15623=ORIENTED_EDGE('',*,*,#11027,.T.);
#15624=ORIENTED_EDGE('',*,*,#11028,.T.);
#15625=ORIENTED_EDGE('',*,*,#11024,.T.);
#15626=ORIENTED_EDGE('',*,*,#11026,.T.);
#15627=ORIENTED_EDGE('',*,*,#11025,.T.);
#15628=ORIENTED_EDGE('',*,*,#11028,.F.);
#15629=ORIENTED_EDGE('',*,*,#11029,.T.);
#15630=ORIENTED_EDGE('',*,*,#10819,.T.);
#15631=ORIENTED_EDGE('',*,*,#10820,.F.);
#15632=ORIENTED_EDGE('',*,*,#11029,.F.);
#15633=ORIENTED_EDGE('',*,*,#11027,.F.);
#15634=ORIENTED_EDGE('',*,*,#11021,.F.);
#15635=ORIENTED_EDGE('',*,*,#11030,.F.);
#15636=ORIENTED_EDGE('',*,*,#10733,.F.);
#15637=ORIENTED_EDGE('',*,*,#10735,.T.);
#15638=ORIENTED_EDGE('',*,*,#10776,.F.);
#15639=ORIENTED_EDGE('',*,*,#11031,.T.);
#15640=ORIENTED_EDGE('',*,*,#10867,.T.);
#15641=ORIENTED_EDGE('',*,*,#11031,.F.);
#15642=ORIENTED_EDGE('',*,*,#10734,.F.);
#15643=ORIENTED_EDGE('',*,*,#11030,.T.);
#15644=ORIENTED_EDGE('',*,*,#11020,.F.);
#15645=ORIENTED_EDGE('',*,*,#10871,.T.);
#15646=ORIENTED_EDGE('',*,*,#11032,.F.);
#15647=ORIENTED_EDGE('',*,*,#11033,.T.);
#15648=ORIENTED_EDGE('',*,*,#11018,.T.);
#15649=ORIENTED_EDGE('',*,*,#11019,.T.);
#15650=ORIENTED_EDGE('',*,*,#11033,.F.);
#15651=ORIENTED_EDGE('',*,*,#11034,.F.);
#15652=ORIENTED_EDGE('',*,*,#11035,.T.);
#15653=ORIENTED_EDGE('',*,*,#11032,.T.);
#15654=ORIENTED_EDGE('',*,*,#11035,.F.);
#15655=ORIENTED_EDGE('',*,*,#10870,.F.);
#15656=ORIENTED_EDGE('',*,*,#11036,.T.);
#15657=ORIENTED_EDGE('',*,*,#11034,.T.);
#15658=ORIENTED_EDGE('',*,*,#11036,.F.);
#17314=CYLINDRICAL_SURFACE('',#19237,39.);
#17315=CYLINDRICAL_SURFACE('',#19297,3.525);
#17316=CYLINDRICAL_SURFACE('',#19365,8.7);
#17923=ADVANCED_FACE('',(#1895),#1082,.T.);
#17924=ADVANCED_FACE('',(#1896),#922,.T.);
#17925=ADVANCED_FACE('',(#1897),#17314,.T.);
#17926=ADVANCED_FACE('',(#1898),#923,.T.);
#17927=ADVANCED_FACE('',(#1899),#924,.T.);
#17928=ADVANCED_FACE('',(#1900),#925,.T.);
#17929=ADVANCED_FACE('',(#1901),#926,.T.);
#17930=ADVANCED_FACE('',(#1902),#927,.T.);
#17931=ADVANCED_FACE('',(#1903),#928,.T.);
#17932=ADVANCED_FACE('',(#1904),#929,.T.);
#17933=ADVANCED_FACE('',(#1905),#930,.T.);
#17934=ADVANCED_FACE('',(#1906),#931,.T.);
#17935=ADVANCED_FACE('',(#1907),#932,.T.);
#17936=ADVANCED_FACE('',(#1908),#933,.T.);
#17937=ADVANCED_FACE('',(#1909),#934,.T.);
#17938=ADVANCED_FACE('',(#1910),#935,.T.);
#17939=ADVANCED_FACE('',(#1911),#936,.F.);
#17940=ADVANCED_FACE('',(#1912),#17315,.F.);
#17941=ADVANCED_FACE('',(#1913,#241),#608,.T.);
#17942=ADVANCED_FACE('',(#1914),#937,.F.);
#17943=ADVANCED_FACE('',(#1915,#242),#609,.T.);
#17944=ADVANCED_FACE('',(#1916),#131,.F.);
#17945=ADVANCED_FACE('',(#1917),#610,.T.);
#17946=ADVANCED_FACE('',(#1918),#1083,.T.);
#17947=ADVANCED_FACE('',(#1919),#132,.T.);
#17948=ADVANCED_FACE('',(#1920),#938,.T.);
#17949=ADVANCED_FACE('',(#1921),#133,.F.);
#17950=ADVANCED_FACE('',(#1922),#611,.T.);
#17951=ADVANCED_FACE('',(#1923),#1084,.T.);
#17952=ADVANCED_FACE('',(#1924),#134,.T.);
#17953=ADVANCED_FACE('',(#1925),#939,.T.);
#17954=ADVANCED_FACE('',(#1926),#135,.F.);
#17955=ADVANCED_FACE('',(#1927),#612,.T.);
#17956=ADVANCED_FACE('',(#1928),#1085,.T.);
#17957=ADVANCED_FACE('',(#1929),#136,.T.);
#17958=ADVANCED_FACE('',(#1930),#940,.T.);
#17959=ADVANCED_FACE('',(#1931),#137,.F.);
#17960=ADVANCED_FACE('',(#1932),#613,.T.);
#17961=ADVANCED_FACE('',(#1933),#1086,.T.);
#17962=ADVANCED_FACE('',(#1934),#138,.T.);
#17963=ADVANCED_FACE('',(#1935),#941,.T.);
#17964=ADVANCED_FACE('',(#1936),#139,.F.);
#17965=ADVANCED_FACE('',(#1937),#614,.T.);
#17966=ADVANCED_FACE('',(#1938),#1087,.T.);
#17967=ADVANCED_FACE('',(#1939),#140,.T.);
#17968=ADVANCED_FACE('',(#1940),#942,.T.);
#17969=ADVANCED_FACE('',(#1941),#141,.F.);
#17970=ADVANCED_FACE('',(#1942),#615,.T.);
#17971=ADVANCED_FACE('',(#1943),#1088,.T.);
#17972=ADVANCED_FACE('',(#1944),#142,.T.);
#17973=ADVANCED_FACE('',(#1945),#943,.T.);
#17974=ADVANCED_FACE('',(#1946),#143,.F.);
#17975=ADVANCED_FACE('',(#1947),#616,.T.);
#17976=ADVANCED_FACE('',(#1948),#1089,.T.);
#17977=ADVANCED_FACE('',(#1949),#144,.T.);
#17978=ADVANCED_FACE('',(#1950),#944,.T.);
#17979=ADVANCED_FACE('',(#1951),#145,.F.);
#17980=ADVANCED_FACE('',(#1952),#617,.T.);
#17981=ADVANCED_FACE('',(#1953),#1090,.T.);
#17982=ADVANCED_FACE('',(#1954),#146,.T.);
#17983=ADVANCED_FACE('',(#1955),#945,.T.);
#17984=ADVANCED_FACE('',(#1956),#147,.F.);
#17985=ADVANCED_FACE('',(#1957),#618,.T.);
#17986=ADVANCED_FACE('',(#1958),#1091,.T.);
#17987=ADVANCED_FACE('',(#1959),#148,.T.);
#17988=ADVANCED_FACE('',(#1960),#946,.T.);
#17989=ADVANCED_FACE('',(#1961),#149,.F.);
#17990=ADVANCED_FACE('',(#1962),#619,.T.);
#17991=ADVANCED_FACE('',(#1963),#1092,.T.);
#17992=ADVANCED_FACE('',(#1964),#150,.T.);
#17993=ADVANCED_FACE('',(#1965),#947,.T.);
#17994=ADVANCED_FACE('',(#1966),#151,.F.);
#17995=ADVANCED_FACE('',(#1967),#620,.T.);
#17996=ADVANCED_FACE('',(#1968),#1093,.T.);
#17997=ADVANCED_FACE('',(#1969),#152,.T.);
#17998=ADVANCED_FACE('',(#1970),#948,.T.);
#17999=ADVANCED_FACE('',(#1971),#153,.F.);
#18000=ADVANCED_FACE('',(#1972),#621,.T.);
#18001=ADVANCED_FACE('',(#1973),#1094,.T.);
#18002=ADVANCED_FACE('',(#1974),#154,.T.);
#18003=ADVANCED_FACE('',(#1975),#949,.T.);
#18004=ADVANCED_FACE('',(#1976),#155,.F.);
#18005=ADVANCED_FACE('',(#1977),#622,.T.);
#18006=ADVANCED_FACE('',(#1978),#1095,.T.);
#18007=ADVANCED_FACE('',(#1979),#156,.T.);
#18008=ADVANCED_FACE('',(#1980),#950,.T.);
#18009=ADVANCED_FACE('',(#1981),#1096,.T.);
#18010=ADVANCED_FACE('',(#1982),#157,.F.);
#18011=ADVANCED_FACE('',(#1983),#623,.T.);
#18012=ADVANCED_FACE('',(#1984),#1097,.T.);
#18013=ADVANCED_FACE('',(#1985),#158,.T.);
#18014=ADVANCED_FACE('',(#1986),#951,.T.);
#18015=ADVANCED_FACE('',(#1987),#952,.T.);
#18016=ADVANCED_FACE('',(#1988),#953,.T.);
#18017=ADVANCED_FACE('',(#1989),#17316,.T.);
#18018=ADVANCED_FACE('',(#1990),#954,.T.);
#18303=CLOSED_SHELL('',(#17923,#17924,#17925,#17926,#17927,#17928,#17929,
#17930,#17931,#17932,#17933,#17934,#17935,#17936,#17937,#17938,#17939,#17940,
#17941,#17942,#17943,#17944,#17945,#17946,#17947,#17948,#17949,#17950,#17951,
#17952,#17953,#17954,#17955,#17956,#17957,#17958,#17959,#17960,#17961,#17962,
#17963,#17964,#17965,#17966,#17967,#17968,#17969,#17970,#17971,#17972,#17973,
#17974,#17975,#17976,#17977,#17978,#17979,#17980,#17981,#17982,#17983,#17984,
#17985,#17986,#17987,#17988,#17989,#17990,#17991,#17992,#17993,#17994,#17995,
#17996,#17997,#17998,#17999,#18000,#18001,#18002,#18003,#18004,#18005,#18006,
#18007,#18008,#18009,#18010,#18011,#18012,#18013,#18014,#18015,#18016,#18017,
#18018));
#19231=AXIS2_PLACEMENT_3D('',#47065,#22152,#22153);
#19232=AXIS2_PLACEMENT_3D('',#47376,#22154,#22155);
#19233=AXIS2_PLACEMENT_3D('',#47427,#22156,#22157);
#19234=AXIS2_PLACEMENT_3D('',#47480,#22158,#22159);
#19235=AXIS2_PLACEMENT_3D('',#47488,#22160,#22161);
#19236=AXIS2_PLACEMENT_3D('',#47494,#22162,#22163);
#19237=AXIS2_PLACEMENT_3D('',#47495,#22164,#22165);
#19238=AXIS2_PLACEMENT_3D('',#47514,#22166,#22167);
#19239=AXIS2_PLACEMENT_3D('',#47528,#22168,#22169);
#19240=AXIS2_PLACEMENT_3D('',#47542,#22170,#22171);
#19241=AXIS2_PLACEMENT_3D('',#47556,#22172,#22173);
#19242=AXIS2_PLACEMENT_3D('',#47570,#22174,#22175);
#19243=AXIS2_PLACEMENT_3D('',#47584,#22176,#22177);
#19244=AXIS2_PLACEMENT_3D('',#47598,#22178,#22179);
#19245=AXIS2_PLACEMENT_3D('',#47612,#22180,#22181);
#19246=AXIS2_PLACEMENT_3D('',#47626,#22182,#22183);
#19247=AXIS2_PLACEMENT_3D('',#47640,#22184,#22185);
#19248=AXIS2_PLACEMENT_3D('',#47654,#22186,#22187);
#19249=AXIS2_PLACEMENT_3D('',#47668,#22188,#22189);
#19250=AXIS2_PLACEMENT_3D('',#47682,#22190,#22191);
#19251=AXIS2_PLACEMENT_3D('',#47685,#22193,#22194);
#19252=AXIS2_PLACEMENT_3D('',#47687,#22195,#22196);
#19253=AXIS2_PLACEMENT_3D('',#47701,#22197,#22198);
#19254=AXIS2_PLACEMENT_3D('',#47715,#22199,#22200);
#19255=AXIS2_PLACEMENT_3D('',#47729,#22201,#22202);
#19256=AXIS2_PLACEMENT_3D('',#47743,#22203,#22204);
#19257=AXIS2_PLACEMENT_3D('',#47757,#22205,#22206);
#19258=AXIS2_PLACEMENT_3D('',#47771,#22207,#22208);
#19259=AXIS2_PLACEMENT_3D('',#47785,#22209,#22210);
#19260=AXIS2_PLACEMENT_3D('',#47799,#22211,#22212);
#19261=AXIS2_PLACEMENT_3D('',#47813,#22213,#22214);
#19262=AXIS2_PLACEMENT_3D('',#47827,#22215,#22216);
#19263=AXIS2_PLACEMENT_3D('',#47841,#22217,#22218);
#19264=AXIS2_PLACEMENT_3D('',#47855,#22219,#22220);
#19265=AXIS2_PLACEMENT_3D('',#47869,#22221,#22222);
#19266=AXIS2_PLACEMENT_3D('',#47883,#22223,#22224);
#19267=AXIS2_PLACEMENT_3D('',#47890,#22225,#22226);
#19268=AXIS2_PLACEMENT_3D('',#47901,#22227,#22228);
#19269=AXIS2_PLACEMENT_3D('',#47902,#22229,#22230);
#19270=AXIS2_PLACEMENT_3D('',#47913,#22231,#22232);
#19271=AXIS2_PLACEMENT_3D('',#47914,#22233,#22234);
#19272=AXIS2_PLACEMENT_3D('',#47925,#22235,#22236);
#19273=AXIS2_PLACEMENT_3D('',#47926,#22237,#22238);
#19274=AXIS2_PLACEMENT_3D('',#47937,#22239,#22240);
#19275=AXIS2_PLACEMENT_3D('',#47938,#22241,#22242);
#19276=AXIS2_PLACEMENT_3D('',#47949,#22243,#22244);
#19277=AXIS2_PLACEMENT_3D('',#47950,#22245,#22246);
#19278=AXIS2_PLACEMENT_3D('',#47961,#22247,#22248);
#19279=AXIS2_PLACEMENT_3D('',#47962,#22249,#22250);
#19280=AXIS2_PLACEMENT_3D('',#47973,#22251,#22252);
#19281=AXIS2_PLACEMENT_3D('',#47974,#22253,#22254);
#19282=AXIS2_PLACEMENT_3D('',#47985,#22255,#22256);
#19283=AXIS2_PLACEMENT_3D('',#47986,#22257,#22258);
#19284=AXIS2_PLACEMENT_3D('',#47997,#22259,#22260);
#19285=AXIS2_PLACEMENT_3D('',#47998,#22261,#22262);
#19286=AXIS2_PLACEMENT_3D('',#48009,#22263,#22264);
#19287=AXIS2_PLACEMENT_3D('',#48010,#22265,#22266);
#19288=AXIS2_PLACEMENT_3D('',#48021,#22267,#22268);
#19289=AXIS2_PLACEMENT_3D('',#48022,#22269,#22270);
#19290=AXIS2_PLACEMENT_3D('',#48033,#22271,#22272);
#19291=AXIS2_PLACEMENT_3D('',#48034,#22273,#22274);
#19292=AXIS2_PLACEMENT_3D('',#48045,#22275,#22276);
#19293=AXIS2_PLACEMENT_3D('',#48046,#22277,#22278);
#19294=AXIS2_PLACEMENT_3D('',#48048,#22279,#22280);
#19295=AXIS2_PLACEMENT_3D('',#48052,#22282,#22283);
#19296=AXIS2_PLACEMENT_3D('',#48053,#22284,#22285);
#19297=AXIS2_PLACEMENT_3D('',#48054,#22286,#22287);
#19298=AXIS2_PLACEMENT_3D('',#48057,#22288,#22289);
#19299=AXIS2_PLACEMENT_3D('',#48058,#22290,#22291);
#19300=AXIS2_PLACEMENT_3D('',#48060,#22293,#22294);
#19301=AXIS2_PLACEMENT_3D('',#48062,#22295,#22296);
#19302=AXIS2_PLACEMENT_3D('',#48063,#22297,#22298);
#19303=AXIS2_PLACEMENT_3D('',#48066,#22300,#22301);
#19304=AXIS2_PLACEMENT_3D('',#48067,#22302,#22303);
#19305=AXIS2_PLACEMENT_3D('',#48069,#22304,#22305);
#19306=AXIS2_PLACEMENT_3D('',#48245,#22306,#22307);
#19307=AXIS2_PLACEMENT_3D('',#48256,#22308,#22309);
#19308=AXIS2_PLACEMENT_3D('',#48533,#22310,#22311);
#19309=AXIS2_PLACEMENT_3D('',#48535,#22312,#22313);
#19310=AXIS2_PLACEMENT_3D('',#48715,#22314,#22315);
#19311=AXIS2_PLACEMENT_3D('',#48726,#22316,#22317);
#19312=AXIS2_PLACEMENT_3D('',#49003,#22318,#22319);
#19313=AXIS2_PLACEMENT_3D('',#49005,#22320,#22321);
#19314=AXIS2_PLACEMENT_3D('',#49185,#22322,#22323);
#19315=AXIS2_PLACEMENT_3D('',#49196,#22324,#22325);
#19316=AXIS2_PLACEMENT_3D('',#49473,#22326,#22327);
#19317=AXIS2_PLACEMENT_3D('',#49475,#22328,#22329);
#19318=AXIS2_PLACEMENT_3D('',#49655,#22330,#22331);
#19319=AXIS2_PLACEMENT_3D('',#49668,#22332,#22333);
#19320=AXIS2_PLACEMENT_3D('',#49945,#22334,#22335);
#19321=AXIS2_PLACEMENT_3D('',#49947,#22336,#22337);
#19322=AXIS2_PLACEMENT_3D('',#50127,#22338,#22339);
#19323=AXIS2_PLACEMENT_3D('',#50140,#22340,#22341);
#19324=AXIS2_PLACEMENT_3D('',#50417,#22342,#22343);
#19325=AXIS2_PLACEMENT_3D('',#50419,#22344,#22345);
#19326=AXIS2_PLACEMENT_3D('',#50599,#22346,#22347);
#19327=AXIS2_PLACEMENT_3D('',#50610,#22348,#22349);
#19328=AXIS2_PLACEMENT_3D('',#50887,#22350,#22351);
#19329=AXIS2_PLACEMENT_3D('',#50889,#22352,#22353);
#19330=AXIS2_PLACEMENT_3D('',#51039,#22354,#22355);
#19331=AXIS2_PLACEMENT_3D('',#51045,#22356,#22357);
#19332=AXIS2_PLACEMENT_3D('',#51307,#22358,#22359);
#19333=AXIS2_PLACEMENT_3D('',#51560,#22360,#22361);
#19334=AXIS2_PLACEMENT_3D('',#51573,#22362,#22363);
#19335=AXIS2_PLACEMENT_3D('',#52132,#22364,#22365);
#19336=AXIS2_PLACEMENT_3D('',#52133,#22366,#22367);
#19337=AXIS2_PLACEMENT_3D('',#52382,#22368,#22369);
#19338=AXIS2_PLACEMENT_3D('',#52395,#22370,#22371);
#19339=AXIS2_PLACEMENT_3D('',#52984,#22372,#22373);
#19340=AXIS2_PLACEMENT_3D('',#52985,#22374,#22375);
#19341=AXIS2_PLACEMENT_3D('',#53239,#22376,#22377);
#19342=AXIS2_PLACEMENT_3D('',#53252,#22378,#22379);
#19343=AXIS2_PLACEMENT_3D('',#53806,#22380,#22381);
#19344=AXIS2_PLACEMENT_3D('',#53807,#22382,#22383);
#19345=AXIS2_PLACEMENT_3D('',#54056,#22384,#22385);
#19346=AXIS2_PLACEMENT_3D('',#54069,#22386,#22387);
#19347=AXIS2_PLACEMENT_3D('',#54658,#22388,#22389);
#19348=AXIS2_PLACEMENT_3D('',#54659,#22390,#22391);
#19349=AXIS2_PLACEMENT_3D('',#54908,#22392,#22393);
#19350=AXIS2_PLACEMENT_3D('',#54921,#22394,#22395);
#19351=AXIS2_PLACEMENT_3D('',#55475,#22396,#22397);
#19352=AXIS2_PLACEMENT_3D('',#55476,#22398,#22399);
#19353=AXIS2_PLACEMENT_3D('',#55725,#22400,#22401);
#19354=AXIS2_PLACEMENT_3D('',#55743,#22402,#22403);
#19355=AXIS2_PLACEMENT_3D('',#56253,#22404,#22405);
#19356=AXIS2_PLACEMENT_3D('',#56534,#22406,#22407);
#19357=AXIS2_PLACEMENT_3D('',#56535,#22408,#22409);
#19358=AXIS2_PLACEMENT_3D('',#56537,#22410,#22411);
#19359=AXIS2_PLACEMENT_3D('',#56827,#22412,#22413);
#19360=AXIS2_PLACEMENT_3D('',#56833,#22414,#22415);
#19361=AXIS2_PLACEMENT_3D('',#57369,#22416,#22417);
#19362=AXIS2_PLACEMENT_3D('',#57371,#22419,#22420);
#19363=AXIS2_PLACEMENT_3D('',#57372,#22421,#22422);
#19364=AXIS2_PLACEMENT_3D('',#57374,#22423,#22424);
#19365=AXIS2_PLACEMENT_3D('',#57376,#22426,#22427);
#19366=AXIS2_PLACEMENT_3D('',#57378,#22428,#22429);
#19367=AXIS2_PLACEMENT_3D('',#57380,#22431,#22432);
#22152=DIRECTION('axis',(0.,0.,1.));
#22153=DIRECTION('refdir',(1.,0.,0.));
#22154=DIRECTION('center_axis',(1.,0.,0.));
#22155=DIRECTION('ref_axis',(0.,0.,-1.));
#22156=DIRECTION('center_axis',(1.,0.,0.));
#22157=DIRECTION('ref_axis',(0.,0.,-1.));
#22158=DIRECTION('center_axis',(-1.,0.,3.38602178801704E-15));
#22159=DIRECTION('ref_axis',(0.,1.,3.0434711729182E-17));
#22160=DIRECTION('center_axis',(1.,0.,0.));
#22161=DIRECTION('ref_axis',(0.,1.,0.));
#22162=DIRECTION('center_axis',(-1.,0.,0.));
#22163=DIRECTION('ref_axis',(0.,1.,6.12323399573677E-17));
#22164=DIRECTION('center_axis',(1.,0.,0.));
#22165=DIRECTION('ref_axis',(0.,1.,0.));
#22166=DIRECTION('center_axis',(1.,0.,0.));
#22167=DIRECTION('ref_axis',(0.,-0.78183148246803,-0.623489801858733));
#22168=DIRECTION('center_axis',(1.,0.,0.));
#22169=DIRECTION('ref_axis',(0.,1.,0.));
#22170=DIRECTION('center_axis',(1.,0.,0.));
#22171=DIRECTION('ref_axis',(0.,-0.78183148246803,-0.623489801858733));
#22172=DIRECTION('center_axis',(1.,0.,0.));
#22173=DIRECTION('ref_axis',(0.,1.,0.));
#22174=DIRECTION('center_axis',(1.,0.,0.));
#22175=DIRECTION('ref_axis',(0.,-0.974927912181824,0.222520933956315));
#22176=DIRECTION('center_axis',(1.,0.,0.));
#22177=DIRECTION('ref_axis',(0.,1.,0.));
#22178=DIRECTION('center_axis',(1.,0.,0.));
#22179=DIRECTION('ref_axis',(0.,-0.974927912181824,0.222520933956315));
#22180=DIRECTION('center_axis',(1.,0.,0.));
#22181=DIRECTION('ref_axis',(0.,-1.,0.));
#22182=DIRECTION('center_axis',(1.,0.,0.));
#22183=DIRECTION('ref_axis',(0.,-0.433883739117558,0.900968867902419));
#22184=DIRECTION('center_axis',(1.,0.,0.));
#22185=DIRECTION('ref_axis',(0.,-1.,0.));
#22186=DIRECTION('center_axis',(1.,0.,0.));
#22187=DIRECTION('ref_axis',(0.,-0.433883739117558,0.900968867902419));
#22188=DIRECTION('center_axis',(1.,0.,0.));
#22189=DIRECTION('ref_axis',(0.,-1.,0.));
#22190=DIRECTION('center_axis',(1.,0.,0.));
#22191=DIRECTION('ref_axis',(0.,0.433883739117558,0.900968867902419));
#22192=DIRECTION('',(-1.,0.,0.));
#22193=DIRECTION('center_axis',(1.,0.,0.));
#22194=DIRECTION('ref_axis',(0.,0.,-1.));
#22195=DIRECTION('center_axis',(1.,0.,0.));
#22196=DIRECTION('ref_axis',(0.,0.433883739117558,0.900968867902419));
#22197=DIRECTION('center_axis',(1.,0.,0.));
#22198=DIRECTION('ref_axis',(0.,-1.,0.));
#22199=DIRECTION('center_axis',(1.,0.,0.));
#22200=DIRECTION('ref_axis',(0.,0.433883739117558,0.900968867902419));
#22201=DIRECTION('center_axis',(1.,0.,0.));
#22202=DIRECTION('ref_axis',(0.,-1.,0.));
#22203=DIRECTION('center_axis',(1.,0.,0.));
#22204=DIRECTION('ref_axis',(0.,0.974927912181824,0.222520933956314));
#22205=DIRECTION('center_axis',(1.,0.,0.));
#22206=DIRECTION('ref_axis',(0.,-1.,0.));
#22207=DIRECTION('center_axis',(1.,0.,0.));
#22208=DIRECTION('ref_axis',(0.,0.974927912181824,0.222520933956314));
#22209=DIRECTION('center_axis',(1.,0.,0.));
#22210=DIRECTION('ref_axis',(0.,1.,0.));
#22211=DIRECTION('center_axis',(1.,0.,0.));
#22212=DIRECTION('ref_axis',(0.,0.78183148246803,-0.623489801858734));
#22213=DIRECTION('center_axis',(1.,0.,0.));
#22214=DIRECTION('ref_axis',(0.,1.,0.));
#22215=DIRECTION('center_axis',(1.,0.,0.));
#22216=DIRECTION('ref_axis',(0.,0.78183148246803,-0.623489801858734));
#22217=DIRECTION('center_axis',(1.,0.,0.));
#22218=DIRECTION('ref_axis',(0.,1.,0.));
#22219=DIRECTION('center_axis',(1.,0.,0.));
#22220=DIRECTION('ref_axis',(0.,0.,-1.));
#22221=DIRECTION('center_axis',(1.,0.,0.));
#22222=DIRECTION('ref_axis',(0.,1.,0.));
#22223=DIRECTION('center_axis',(1.,0.,0.));
#22224=DIRECTION('ref_axis',(0.,0.,-1.));
#22225=DIRECTION('center_axis',(-1.,0.,3.38602178801705E-15));
#22226=DIRECTION('ref_axis',(0.,1.,3.0434711729182E-17));
#22227=DIRECTION('center_axis',(-1.,0.,0.));
#22228=DIRECTION('ref_axis',(0.,1.,6.12323399573677E-17));
#22229=DIRECTION('center_axis',(-1.,0.,3.38602178801705E-15));
#22230=DIRECTION('ref_axis',(0.,1.,3.0434711729182E-17));
#22231=DIRECTION('center_axis',(-1.,0.,0.));
#22232=DIRECTION('ref_axis',(0.,1.,6.12323399573677E-17));
#22233=DIRECTION('center_axis',(-1.,0.,3.38602178801705E-15));
#22234=DIRECTION('ref_axis',(0.,-1.,-3.0434711729182E-17));
#22235=DIRECTION('center_axis',(-1.,0.,0.));
#22236=DIRECTION('ref_axis',(0.,-1.,-6.12323399573677E-17));
#22237=DIRECTION('center_axis',(-1.,0.,3.38602178801704E-15));
#22238=DIRECTION('ref_axis',(0.,-1.,-3.0434711729182E-17));
#22239=DIRECTION('center_axis',(-1.,0.,0.));
#22240=DIRECTION('ref_axis',(0.,-1.,-6.12323399573677E-17));
#22241=DIRECTION('center_axis',(-1.,0.,3.38602178801705E-15));
#22242=DIRECTION('ref_axis',(0.,-1.,-3.0434711729182E-17));
#22243=DIRECTION('center_axis',(-1.,0.,0.));
#22244=DIRECTION('ref_axis',(0.,-1.,-6.12323399573677E-17));
#22245=DIRECTION('center_axis',(-1.,0.,3.38602178801704E-15));
#22246=DIRECTION('ref_axis',(0.,1.,3.0434711729182E-17));
#22247=DIRECTION('center_axis',(-1.,0.,0.));
#22248=DIRECTION('ref_axis',(0.,1.,6.12323399573677E-17));
#22249=DIRECTION('center_axis',(-1.,0.,3.38602178801704E-15));
#22250=DIRECTION('ref_axis',(0.,1.,3.0434711729182E-17));
#22251=DIRECTION('center_axis',(-1.,0.,0.));
#22252=DIRECTION('ref_axis',(0.,1.,6.12323399573677E-17));
#22253=DIRECTION('center_axis',(-1.,0.,3.38602178801704E-15));
#22254=DIRECTION('ref_axis',(0.,1.,3.0434711729182E-17));
#22255=DIRECTION('center_axis',(-1.,0.,0.));
#22256=DIRECTION('ref_axis',(0.,1.,6.12323399573677E-17));
#22257=DIRECTION('center_axis',(-1.,0.,3.38602178801704E-15));
#22258=DIRECTION('ref_axis',(0.,-1.,-3.0434711729182E-17));
#22259=DIRECTION('center_axis',(-1.,0.,0.));
#22260=DIRECTION('ref_axis',(0.,-1.,-6.12323399573677E-17));
#22261=DIRECTION('center_axis',(-1.,0.,3.38602178801704E-15));
#22262=DIRECTION('ref_axis',(0.,-1.,-3.0434711729182E-17));
#22263=DIRECTION('center_axis',(-1.,0.,0.));
#22264=DIRECTION('ref_axis',(0.,-1.,-6.12323399573677E-17));
#22265=DIRECTION('center_axis',(-1.,0.,3.38602178801704E-15));
#22266=DIRECTION('ref_axis',(0.,-1.,-3.0434711729182E-17));
#22267=DIRECTION('center_axis',(-1.,0.,0.));
#22268=DIRECTION('ref_axis',(0.,-1.,-6.12323399573677E-17));
#22269=DIRECTION('center_axis',(-1.,0.,3.38602178801705E-15));
#22270=DIRECTION('ref_axis',(0.,1.,3.0434711729182E-17));
#22271=DIRECTION('center_axis',(-1.,0.,0.));
#22272=DIRECTION('ref_axis',(0.,1.,6.12323399573677E-17));
#22273=DIRECTION('center_axis',(-1.,0.,3.38602178801704E-15));
#22274=DIRECTION('ref_axis',(0.,1.,3.0434711729182E-17));
#22275=DIRECTION('center_axis',(-1.,0.,0.));
#22276=DIRECTION('ref_axis',(0.,1.,6.12323399573677E-17));
#22277=DIRECTION('center_axis',(-1.,0.,0.));
#22278=DIRECTION('ref_axis',(0.,-1.,0.));
#22279=DIRECTION('center_axis',(-1.,0.,0.));
#22280=DIRECTION('ref_axis',(0.,-1.,0.));
#22281=DIRECTION('',(0.707106781186548,-0.707106781186547,8.65956056235493E-17));
#22282=DIRECTION('center_axis',(1.,0.,0.));
#22283=DIRECTION('ref_axis',(0.,-1.,0.));
#22284=DIRECTION('center_axis',(1.,0.,0.));
#22285=DIRECTION('ref_axis',(0.,-1.,0.));
#22286=DIRECTION('center_axis',(1.,0.,0.));
#22287=DIRECTION('ref_axis',(0.,1.,0.));
#22288=DIRECTION('center_axis',(-1.,0.,0.));
#22289=DIRECTION('ref_axis',(0.,-1.,0.));
#22290=DIRECTION('center_axis',(-1.,0.,0.));
#22291=DIRECTION('ref_axis',(0.,-1.,0.));
#22292=DIRECTION('',(-1.,0.,0.));
#22293=DIRECTION('center_axis',(-1.,0.,0.));
#22294=DIRECTION('ref_axis',(0.,0.,1.));
#22295=DIRECTION('center_axis',(1.,0.,0.));
#22296=DIRECTION('ref_axis',(0.,0.,-1.));
#22297=DIRECTION('center_axis',(1.,0.,0.));
#22298=DIRECTION('ref_axis',(0.,-1.,0.));
#22299=DIRECTION('',(0.707106781186546,0.707106781186549,-8.65956056235496E-17));
#22300=DIRECTION('center_axis',(1.,0.,0.));
#22301=DIRECTION('ref_axis',(0.,-1.,0.));
#22302=DIRECTION('center_axis',(1.,0.,0.));
#22303=DIRECTION('ref_axis',(0.,0.,-1.));
#22304=DIRECTION('center_axis',(1.,0.,0.));
#22305=DIRECTION('ref_axis',(0.,0.,-1.));
#22306=DIRECTION('center_axis',(1.,0.,0.));
#22307=DIRECTION('ref_axis',(0.,-0.78183148246803,-0.623489801858733));
#22308=DIRECTION('center_axis',(1.,0.,0.));
#22309=DIRECTION('ref_axis',(0.,-0.78183148246803,-0.623489801858733));
#22310=DIRECTION('center_axis',(-1.,0.,0.));
#22311=DIRECTION('ref_axis',(0.,1.,0.));
#22312=DIRECTION('center_axis',(1.,0.,0.));
#22313=DIRECTION('ref_axis',(0.,0.,-1.));
#22314=DIRECTION('center_axis',(1.,0.,0.));
#22315=DIRECTION('ref_axis',(0.,-0.974927912181824,0.222520933956315));
#22316=DIRECTION('center_axis',(1.,0.,0.));
#22317=DIRECTION('ref_axis',(0.,-0.974927912181824,0.222520933956315));
#22318=DIRECTION('center_axis',(-1.,0.,0.));
#22319=DIRECTION('ref_axis',(0.,1.,0.));
#22320=DIRECTION('center_axis',(1.,0.,0.));
#22321=DIRECTION('ref_axis',(0.,0.,-1.));
#22322=DIRECTION('center_axis',(1.,0.,0.));
#22323=DIRECTION('ref_axis',(0.,-0.433883739117558,0.900968867902419));
#22324=DIRECTION('center_axis',(1.,0.,0.));
#22325=DIRECTION('ref_axis',(0.,-0.433883739117558,0.900968867902419));
#22326=DIRECTION('center_axis',(-1.,0.,0.));
#22327=DIRECTION('ref_axis',(0.,1.,0.));
#22328=DIRECTION('center_axis',(1.,0.,0.));
#22329=DIRECTION('ref_axis',(0.,0.,-1.));
#22330=DIRECTION('center_axis',(1.,0.,0.));
#22331=DIRECTION('ref_axis',(0.,0.433883739117558,0.900968867902419));
#22332=DIRECTION('center_axis',(1.,0.,0.));
#22333=DIRECTION('ref_axis',(0.,0.433883739117558,0.900968867902419));
#22334=DIRECTION('center_axis',(-1.,0.,0.));
#22335=DIRECTION('ref_axis',(0.,1.,0.));
#22336=DIRECTION('center_axis',(1.,0.,0.));
#22337=DIRECTION('ref_axis',(0.,0.,-1.));
#22338=DIRECTION('center_axis',(1.,0.,0.));
#22339=DIRECTION('ref_axis',(0.,0.974927912181824,0.222520933956314));
#22340=DIRECTION('center_axis',(1.,0.,0.));
#22341=DIRECTION('ref_axis',(0.,0.974927912181824,0.222520933956314));
#22342=DIRECTION('center_axis',(-1.,0.,0.));
#22343=DIRECTION('ref_axis',(0.,1.,0.));
#22344=DIRECTION('center_axis',(1.,0.,0.));
#22345=DIRECTION('ref_axis',(0.,0.,-1.));
#22346=DIRECTION('center_axis',(1.,0.,0.));
#22347=DIRECTION('ref_axis',(0.,0.78183148246803,-0.623489801858734));
#22348=DIRECTION('center_axis',(1.,0.,0.));
#22349=DIRECTION('ref_axis',(0.,0.78183148246803,-0.623489801858734));
#22350=DIRECTION('center_axis',(-1.,0.,0.));
#22351=DIRECTION('ref_axis',(0.,1.,0.));
#22352=DIRECTION('center_axis',(1.,0.,0.));
#22353=DIRECTION('ref_axis',(0.,0.,-1.));
#22354=DIRECTION('center_axis',(1.,0.,0.));
#22355=DIRECTION('ref_axis',(0.,0.,-1.));
#22356=DIRECTION('center_axis',(1.,0.,0.));
#22357=DIRECTION('ref_axis',(0.,0.,-1.));
#22358=DIRECTION('center_axis',(-1.,0.,0.));
#22359=DIRECTION('ref_axis',(0.,1.,0.));
#22360=DIRECTION('center_axis',(1.,0.,0.));
#22361=DIRECTION('ref_axis',(0.,-0.78183148246803,-0.623489801858733));
#22362=DIRECTION('center_axis',(1.,0.,0.));
#22363=DIRECTION('ref_axis',(0.,-0.78183148246803,-0.623489801858733));
#22364=DIRECTION('center_axis',(-1.,0.,0.));
#22365=DIRECTION('ref_axis',(0.,1.,0.));
#22366=DIRECTION('center_axis',(1.,0.,0.));
#22367=DIRECTION('ref_axis',(0.,0.,-1.));
#22368=DIRECTION('center_axis',(1.,0.,0.));
#22369=DIRECTION('ref_axis',(0.,-0.974927912181824,0.222520933956315));
#22370=DIRECTION('center_axis',(1.,0.,0.));
#22371=DIRECTION('ref_axis',(0.,-0.974927912181824,0.222520933956315));
#22372=DIRECTION('center_axis',(-1.,0.,0.));
#22373=DIRECTION('ref_axis',(0.,1.,0.));
#22374=DIRECTION('center_axis',(1.,0.,0.));
#22375=DIRECTION('ref_axis',(0.,0.,-1.));
#22376=DIRECTION('center_axis',(1.,0.,0.));
#22377=DIRECTION('ref_axis',(0.,-0.433883739117558,0.900968867902419));
#22378=DIRECTION('center_axis',(1.,0.,0.));
#22379=DIRECTION('ref_axis',(0.,-0.433883739117558,0.900968867902419));
#22380=DIRECTION('center_axis',(-1.,0.,0.));
#22381=DIRECTION('ref_axis',(0.,1.,0.));
#22382=DIRECTION('center_axis',(1.,0.,0.));
#22383=DIRECTION('ref_axis',(0.,0.,-1.));
#22384=DIRECTION('center_axis',(1.,0.,0.));
#22385=DIRECTION('ref_axis',(0.,0.433883739117558,0.900968867902419));
#22386=DIRECTION('center_axis',(1.,0.,0.));
#22387=DIRECTION('ref_axis',(0.,0.433883739117558,0.900968867902419));
#22388=DIRECTION('center_axis',(-1.,0.,0.));
#22389=DIRECTION('ref_axis',(0.,1.,0.));
#22390=DIRECTION('center_axis',(1.,0.,0.));
#22391=DIRECTION('ref_axis',(0.,0.,-1.));
#22392=DIRECTION('center_axis',(1.,0.,0.));
#22393=DIRECTION('ref_axis',(0.,0.974927912181824,0.222520933956314));
#22394=DIRECTION('center_axis',(1.,0.,0.));
#22395=DIRECTION('ref_axis',(0.,0.974927912181824,0.222520933956314));
#22396=DIRECTION('center_axis',(-1.,0.,0.));
#22397=DIRECTION('ref_axis',(0.,1.,0.));
#22398=DIRECTION('center_axis',(1.,0.,0.));
#22399=DIRECTION('ref_axis',(0.,0.,-1.));
#22400=DIRECTION('center_axis',(1.,0.,0.));
#22401=DIRECTION('ref_axis',(0.,0.78183148246803,-0.623489801858734));
#22402=DIRECTION('center_axis',(1.,0.,0.));
#22403=DIRECTION('ref_axis',(0.,0.78183148246803,-0.623489801858734));
#22404=DIRECTION('center_axis',(-1.,0.,0.));
#22405=DIRECTION('ref_axis',(0.,1.,0.));
#22406=DIRECTION('center_axis',(1.,0.,0.));
#22407=DIRECTION('ref_axis',(0.,0.,-1.));
#22408=DIRECTION('center_axis',(1.,0.,0.));
#22409=DIRECTION('ref_axis',(0.,0.,-1.));
#22410=DIRECTION('center_axis',(1.,0.,0.));
#22411=DIRECTION('ref_axis',(0.,0.,-1.));
#22412=DIRECTION('center_axis',(1.,0.,0.));
#22413=DIRECTION('ref_axis',(0.,0.,-1.));
#22414=DIRECTION('center_axis',(1.,0.,0.));
#22415=DIRECTION('ref_axis',(0.,0.,-1.));
#22416=DIRECTION('center_axis',(1.,0.,0.));
#22417=DIRECTION('ref_axis',(0.,1.,0.));
#22418=DIRECTION('',(-0.707106781186549,0.707106781186546,8.65956056235492E-17));
#22419=DIRECTION('center_axis',(-1.,0.,0.));
#22420=DIRECTION('ref_axis',(0.,1.,0.));
#22421=DIRECTION('center_axis',(-1.,0.,0.));
#22422=DIRECTION('ref_axis',(0.,1.,0.));
#22423=DIRECTION('center_axis',(1.,0.,0.));
#22424=DIRECTION('ref_axis',(0.,0.,-1.));
#22425=DIRECTION('',(-0.371390676354097,-0.928476690885262,-1.13705600757556E-16));
#22426=DIRECTION('center_axis',(1.,0.,0.));
#22427=DIRECTION('ref_axis',(0.,1.,0.));
#22428=DIRECTION('center_axis',(1.,0.,0.));
#22429=DIRECTION('ref_axis',(0.,0.,-1.));
#22430=DIRECTION('',(-1.,0.,0.));
#22431=DIRECTION('center_axis',(-1.,0.,0.));
#22432=DIRECTION('ref_axis',(0.,1.,0.));
#22433=DIRECTION('',(-0.707106781186548,-0.707106781186547,-8.65956056235493E-17));
#47065=CARTESIAN_POINT('',(0.,0.,0.));
#47066=CARTESIAN_POINT('Ctrl Pts',(27.,9.2,0.));
#47067=CARTESIAN_POINT('Ctrl Pts',(27.,9.2,9.2));
#47068=CARTESIAN_POINT('Ctrl Pts',(27.,0.,9.2));
#47069=CARTESIAN_POINT('Ctrl Pts',(27.,-9.2,9.2));
#47070=CARTESIAN_POINT('Ctrl Pts',(27.,-9.2,0.));
#47071=CARTESIAN_POINT('Ctrl Pts',(27.,-9.2,-9.2));
#47072=CARTESIAN_POINT('Ctrl Pts',(27.,0.,-9.2));
#47073=CARTESIAN_POINT('Ctrl Pts',(27.,9.2,-9.2));
#47074=CARTESIAN_POINT('Ctrl Pts',(27.,9.2,0.));
#47075=CARTESIAN_POINT('Ctrl Pts',(26.796570998452,9.22636560737002,0.));
#47076=CARTESIAN_POINT('Ctrl Pts',(26.796570998452,9.22636560737001,9.22636560737001));
#47077=CARTESIAN_POINT('Ctrl Pts',(26.796570998452,0.,9.22636560737002));
#47078=CARTESIAN_POINT('Ctrl Pts',(26.796570998452,-9.22636560737001,9.22636560737001));
#47079=CARTESIAN_POINT('Ctrl Pts',(26.796570998452,-9.22636560737002,0.));
#47080=CARTESIAN_POINT('Ctrl Pts',(26.796570998452,-9.22636560737001,-9.22636560737001));
#47081=CARTESIAN_POINT('Ctrl Pts',(26.796570998452,0.,-9.22636560737002));
#47082=CARTESIAN_POINT('Ctrl Pts',(26.796570998452,9.22636560737001,-9.22636560737001));
#47083=CARTESIAN_POINT('Ctrl Pts',(26.796570998452,9.22636560737002,0.));
#47084=CARTESIAN_POINT('Ctrl Pts',(26.3874085880356,9.28597940593777,0.));
#47085=CARTESIAN_POINT('Ctrl Pts',(26.3874085880356,9.28597940593777,9.28597940593777));
#47086=CARTESIAN_POINT('Ctrl Pts',(26.3874085880356,0.,9.28597940593777));
#47087=CARTESIAN_POINT('Ctrl Pts',(26.3874085880356,-9.28597940593777,9.28597940593777));
#47088=CARTESIAN_POINT('Ctrl Pts',(26.3874085880356,-9.28597940593777,0.));
#47089=CARTESIAN_POINT('Ctrl Pts',(26.3874085880356,-9.28597940593777,-9.28597940593777));
#47090=CARTESIAN_POINT('Ctrl Pts',(26.3874085880356,0.,-9.28597940593777));
#47091=CARTESIAN_POINT('Ctrl Pts',(26.3874085880356,9.28597940593777,-9.28597940593777));
#47092=CARTESIAN_POINT('Ctrl Pts',(26.3874085880356,9.28597940593777,0.));
#47093=CARTESIAN_POINT('Ctrl Pts',(25.7667517823113,9.39604887090672,0.));
#47094=CARTESIAN_POINT('Ctrl Pts',(25.7667517823113,9.39604887090672,9.39604887090672));
#47095=CARTESIAN_POINT('Ctrl Pts',(25.7667517823113,0.,9.39604887090672));
#47096=CARTESIAN_POINT('Ctrl Pts',(25.7667517823113,-9.39604887090672,9.39604887090672));
#47097=CARTESIAN_POINT('Ctrl Pts',(25.7667517823113,-9.39604887090672,0.));
#47098=CARTESIAN_POINT('Ctrl Pts',(25.7667517823113,-9.39604887090672,-9.39604887090672));
#47099=CARTESIAN_POINT('Ctrl Pts',(25.7667517823113,0.,-9.39604887090672));
#47100=CARTESIAN_POINT('Ctrl Pts',(25.7667517823113,9.39604887090672,-9.39604887090672));
#47101=CARTESIAN_POINT('Ctrl Pts',(25.7667517823113,9.39604887090672,0.));
#47102=CARTESIAN_POINT('Ctrl Pts',(24.9253466419639,9.58420457526839,0.));
#47103=CARTESIAN_POINT('Ctrl Pts',(24.9253466419639,9.58420457526839,9.58420457526839));
#47104=CARTESIAN_POINT('Ctrl Pts',(24.9253466419639,0.,9.58420457526839));
#47105=CARTESIAN_POINT('Ctrl Pts',(24.9253466419639,-9.58420457526839,9.58420457526839));
#47106=CARTESIAN_POINT('Ctrl Pts',(24.9253466419639,-9.58420457526839,0.));
#47107=CARTESIAN_POINT('Ctrl Pts',(24.9253466419639,-9.58420457526839,-9.58420457526839));
#47108=CARTESIAN_POINT('Ctrl Pts',(24.9253466419639,0.,-9.58420457526839));
#47109=CARTESIAN_POINT('Ctrl Pts',(24.9253466419639,9.58420457526839,-9.58420457526839));
#47110=CARTESIAN_POINT('Ctrl Pts',(24.9253466419639,9.58420457526839,0.));
#47111=CARTESIAN_POINT('Ctrl Pts',(23.8505404645239,9.89058631634017,0.));
#47112=CARTESIAN_POINT('Ctrl Pts',(23.8505404645239,9.89058631634017,9.89058631634017));
#47113=CARTESIAN_POINT('Ctrl Pts',(23.8505404645239,0.,9.89058631634017));
#47114=CARTESIAN_POINT('Ctrl Pts',(23.8505404645239,-9.89058631634017,9.89058631634017));
#47115=CARTESIAN_POINT('Ctrl Pts',(23.8505404645239,-9.89058631634017,0.));
#47116=CARTESIAN_POINT('Ctrl Pts',(23.8505404645239,-9.89058631634017,-9.89058631634017));
#47117=CARTESIAN_POINT('Ctrl Pts',(23.8505404645239,0.,-9.89058631634017));
#47118=CARTESIAN_POINT('Ctrl Pts',(23.8505404645239,9.89058631634017,-9.89058631634017));
#47119=CARTESIAN_POINT('Ctrl Pts',(23.8505404645239,9.89058631634017,0.));
#47120=CARTESIAN_POINT('Ctrl Pts',(22.7532142104752,10.273481509771,0.));
#47121=CARTESIAN_POINT('Ctrl Pts',(22.7532142104752,10.273481509771,10.273481509771));
#47122=CARTESIAN_POINT('Ctrl Pts',(22.7532142104752,0.,10.273481509771));
#47123=CARTESIAN_POINT('Ctrl Pts',(22.7532142104752,-10.273481509771,10.273481509771));
#47124=CARTESIAN_POINT('Ctrl Pts',(22.7532142104752,-10.273481509771,0.));
#47125=CARTESIAN_POINT('Ctrl Pts',(22.7532142104752,-10.273481509771,-10.273481509771));
#47126=CARTESIAN_POINT('Ctrl Pts',(22.7532142104752,0.,-10.273481509771));
#47127=CARTESIAN_POINT('Ctrl Pts',(22.7532142104752,10.273481509771,-10.273481509771));
#47128=CARTESIAN_POINT('Ctrl Pts',(22.7532142104752,10.273481509771,0.));
#47129=CARTESIAN_POINT('Ctrl Pts',(21.6347255505832,10.7430346646081,0.));
#47130=CARTESIAN_POINT('Ctrl Pts',(21.6347255505832,10.7430346646081,10.7430346646081));
#47131=CARTESIAN_POINT('Ctrl Pts',(21.6347255505832,0.,10.7430346646081));
#47132=CARTESIAN_POINT('Ctrl Pts',(21.6347255505832,-10.7430346646081,10.7430346646081));
#47133=CARTESIAN_POINT('Ctrl Pts',(21.6347255505832,-10.7430346646081,0.));
#47134=CARTESIAN_POINT('Ctrl Pts',(21.6347255505832,-10.7430346646081,-10.7430346646081));
#47135=CARTESIAN_POINT('Ctrl Pts',(21.6347255505832,0.,-10.7430346646081));
#47136=CARTESIAN_POINT('Ctrl Pts',(21.6347255505832,10.7430346646081,-10.7430346646081));
#47137=CARTESIAN_POINT('Ctrl Pts',(21.6347255505832,10.7430346646081,0.));
#47138=CARTESIAN_POINT('Ctrl Pts',(20.4975894383762,11.3145134298179,0.));
#47139=CARTESIAN_POINT('Ctrl Pts',(20.4975894383762,11.3145134298179,11.3145134298179));
#47140=CARTESIAN_POINT('Ctrl Pts',(20.4975894383762,0.,11.3145134298179));
#47141=CARTESIAN_POINT('Ctrl Pts',(20.4975894383762,-11.3145134298179,11.3145134298179));
#47142=CARTESIAN_POINT('Ctrl Pts',(20.4975894383762,-11.3145134298179,0.));
#47143=CARTESIAN_POINT('Ctrl Pts',(20.4975894383762,-11.3145134298179,-11.3145134298179));
#47144=CARTESIAN_POINT('Ctrl Pts',(20.4975894383762,0.,-11.3145134298179));
#47145=CARTESIAN_POINT('Ctrl Pts',(20.4975894383762,11.3145134298179,-11.3145134298179));
#47146=CARTESIAN_POINT('Ctrl Pts',(20.4975894383762,11.3145134298179,0.));
#47147=CARTESIAN_POINT('Ctrl Pts',(19.3456615791409,12.0038530129696,0.));
#47148=CARTESIAN_POINT('Ctrl Pts',(19.3456615791409,12.0038530129696,12.0038530129696));
#47149=CARTESIAN_POINT('Ctrl Pts',(19.3456615791409,0.,12.0038530129696));
#47150=CARTESIAN_POINT('Ctrl Pts',(19.3456615791409,-12.0038530129696,12.0038530129696));
#47151=CARTESIAN_POINT('Ctrl Pts',(19.3456615791409,-12.0038530129696,0.));
#47152=CARTESIAN_POINT('Ctrl Pts',(19.3456615791409,-12.0038530129696,-12.0038530129696));
#47153=CARTESIAN_POINT('Ctrl Pts',(19.3456615791409,0.,-12.0038530129696));
#47154=CARTESIAN_POINT('Ctrl Pts',(19.3456615791409,12.0038530129696,-12.0038530129696));
#47155=CARTESIAN_POINT('Ctrl Pts',(19.3456615791409,12.0038530129696,0.));
#47156=CARTESIAN_POINT('Ctrl Pts',(18.1843885347784,12.8237912132616,0.));
#47157=CARTESIAN_POINT('Ctrl Pts',(18.1843885347784,12.8237912132616,12.8237912132616));
#47158=CARTESIAN_POINT('Ctrl Pts',(18.1843885347784,0.,12.8237912132616));
#47159=CARTESIAN_POINT('Ctrl Pts',(18.1843885347784,-12.8237912132616,12.8237912132616));
#47160=CARTESIAN_POINT('Ctrl Pts',(18.1843885347784,-12.8237912132616,0.));
#47161=CARTESIAN_POINT('Ctrl Pts',(18.1843885347784,-12.8237912132616,-12.8237912132616));
#47162=CARTESIAN_POINT('Ctrl Pts',(18.1843885347784,0.,-12.8237912132616));
#47163=CARTESIAN_POINT('Ctrl Pts',(18.1843885347784,12.8237912132616,-12.8237912132616));
#47164=CARTESIAN_POINT('Ctrl Pts',(18.1843885347784,12.8237912132616,0.));
#47165=CARTESIAN_POINT('Ctrl Pts',(17.0210036637821,13.7799946040807,0.));
#47166=CARTESIAN_POINT('Ctrl Pts',(17.0210036637821,13.7799946040807,13.7799946040807));
#47167=CARTESIAN_POINT('Ctrl Pts',(17.0210036637821,0.,13.7799946040807));
#47168=CARTESIAN_POINT('Ctrl Pts',(17.0210036637821,-13.7799946040807,13.7799946040807));
#47169=CARTESIAN_POINT('Ctrl Pts',(17.0210036637821,-13.7799946040807,0.));
#47170=CARTESIAN_POINT('Ctrl Pts',(17.0210036637821,-13.7799946040807,-13.7799946040807));
#47171=CARTESIAN_POINT('Ctrl Pts',(17.0210036637821,0.,-13.7799946040807));
#47172=CARTESIAN_POINT('Ctrl Pts',(17.0210036637821,13.7799946040807,-13.7799946040807));
#47173=CARTESIAN_POINT('Ctrl Pts',(17.0210036637821,13.7799946040807,0.));
#47174=CARTESIAN_POINT('Ctrl Pts',(15.8649034353727,14.8662985491428,0.));
#47175=CARTESIAN_POINT('Ctrl Pts',(15.8649034353727,14.8662985491428,14.8662985491428));
#47176=CARTESIAN_POINT('Ctrl Pts',(15.8649034353727,0.,14.8662985491428));
#47177=CARTESIAN_POINT('Ctrl Pts',(15.8649034353727,-14.8662985491428,14.8662985491428));
#47178=CARTESIAN_POINT('Ctrl Pts',(15.8649034353727,-14.8662985491428,0.));
#47179=CARTESIAN_POINT('Ctrl Pts',(15.8649034353727,-14.8662985491428,-14.8662985491428));
#47180=CARTESIAN_POINT('Ctrl Pts',(15.8649034353727,0.,-14.8662985491428));
#47181=CARTESIAN_POINT('Ctrl Pts',(15.8649034353727,14.8662985491428,-14.8662985491428));
#47182=CARTESIAN_POINT('Ctrl Pts',(15.8649034353727,14.8662985491428,0.));
#47183=CARTESIAN_POINT('Ctrl Pts',(14.7267277676362,16.0674034956045,0.));
#47184=CARTESIAN_POINT('Ctrl Pts',(14.7267277676362,16.0674034956045,16.0674034956045));
#47185=CARTESIAN_POINT('Ctrl Pts',(14.7267277676362,0.,16.0674034956045));
#47186=CARTESIAN_POINT('Ctrl Pts',(14.7267277676362,-16.0674034956045,16.0674034956045));
#47187=CARTESIAN_POINT('Ctrl Pts',(14.7267277676362,-16.0674034956045,0.));
#47188=CARTESIAN_POINT('Ctrl Pts',(14.7267277676362,-16.0674034956045,-16.0674034956045));
#47189=CARTESIAN_POINT('Ctrl Pts',(14.7267277676362,0.,-16.0674034956045));
#47190=CARTESIAN_POINT('Ctrl Pts',(14.7267277676362,16.0674034956045,-16.0674034956045));
#47191=CARTESIAN_POINT('Ctrl Pts',(14.7267277676362,16.0674034956045,0.));
#47192=CARTESIAN_POINT('Ctrl Pts',(13.6172459538847,17.362757468191,0.));
#47193=CARTESIAN_POINT('Ctrl Pts',(13.6172459538847,17.362757468191,17.362757468191));
#47194=CARTESIAN_POINT('Ctrl Pts',(13.6172459538847,0.,17.362757468191));
#47195=CARTESIAN_POINT('Ctrl Pts',(13.6172459538847,-17.362757468191,17.362757468191));
#47196=CARTESIAN_POINT('Ctrl Pts',(13.6172459538847,-17.362757468191,0.));
#47197=CARTESIAN_POINT('Ctrl Pts',(13.6172459538847,-17.362757468191,-17.362757468191));
#47198=CARTESIAN_POINT('Ctrl Pts',(13.6172459538847,0.,-17.362757468191));
#47199=CARTESIAN_POINT('Ctrl Pts',(13.6172459538847,17.362757468191,-17.362757468191));
#47200=CARTESIAN_POINT('Ctrl Pts',(13.6172459538847,17.362757468191,0.));
#47201=CARTESIAN_POINT('Ctrl Pts',(12.5462580187496,18.7300247619529,0.));
#47202=CARTESIAN_POINT('Ctrl Pts',(12.5462580187496,18.7300247619529,18.7300247619529));
#47203=CARTESIAN_POINT('Ctrl Pts',(12.5462580187496,0.,18.7300247619529));
#47204=CARTESIAN_POINT('Ctrl Pts',(12.5462580187496,-18.7300247619529,18.7300247619529));
#47205=CARTESIAN_POINT('Ctrl Pts',(12.5462580187496,-18.7300247619529,0.));
#47206=CARTESIAN_POINT('Ctrl Pts',(12.5462580187496,-18.7300247619529,-18.7300247619529));
#47207=CARTESIAN_POINT('Ctrl Pts',(12.5462580187496,0.,-18.7300247619529));
#47208=CARTESIAN_POINT('Ctrl Pts',(12.5462580187496,18.7300247619529,-18.7300247619529));
#47209=CARTESIAN_POINT('Ctrl Pts',(12.5462580187496,18.7300247619529,0.));
#47210=CARTESIAN_POINT('Ctrl Pts',(11.5215838208076,20.1483844597128,0.));
#47211=CARTESIAN_POINT('Ctrl Pts',(11.5215838208076,20.1483844597128,20.1483844597128));
#47212=CARTESIAN_POINT('Ctrl Pts',(11.5215838208076,0.,20.1483844597128));
#47213=CARTESIAN_POINT('Ctrl Pts',(11.5215838208076,-20.1483844597128,20.1483844597128));
#47214=CARTESIAN_POINT('Ctrl Pts',(11.5215838208076,-20.1483844597128,0.));
#47215=CARTESIAN_POINT('Ctrl Pts',(11.5215838208076,-20.1483844597128,-20.1483844597128));
#47216=CARTESIAN_POINT('Ctrl Pts',(11.5215838208076,0.,-20.1483844597128));
#47217=CARTESIAN_POINT('Ctrl Pts',(11.5215838208076,20.1483844597128,-20.1483844597128));
#47218=CARTESIAN_POINT('Ctrl Pts',(11.5215838208076,20.1483844597128,0.));
#47219=CARTESIAN_POINT('Ctrl Pts',(10.5477031262524,21.602527086122,0.));
#47220=CARTESIAN_POINT('Ctrl Pts',(10.5477031262524,21.602527086122,21.602527086122));
#47221=CARTESIAN_POINT('Ctrl Pts',(10.5477031262524,0.,21.602527086122));
#47222=CARTESIAN_POINT('Ctrl Pts',(10.5477031262524,-21.602527086122,21.602527086122));
#47223=CARTESIAN_POINT('Ctrl Pts',(10.5477031262524,-21.602527086122,0.));
#47224=CARTESIAN_POINT('Ctrl Pts',(10.5477031262524,-21.602527086122,-21.602527086122));
#47225=CARTESIAN_POINT('Ctrl Pts',(10.5477031262524,0.,-21.602527086122));
#47226=CARTESIAN_POINT('Ctrl Pts',(10.5477031262524,21.602527086122,-21.602527086122));
#47227=CARTESIAN_POINT('Ctrl Pts',(10.5477031262524,21.602527086122,0.));
#47228=CARTESIAN_POINT('Ctrl Pts',(9.62553662153839,23.0838998256659,0.));
#47229=CARTESIAN_POINT('Ctrl Pts',(9.62553662153839,23.0838998256659,23.0838998256659));
#47230=CARTESIAN_POINT('Ctrl Pts',(9.62553662153839,0.,23.0838998256659));
#47231=CARTESIAN_POINT('Ctrl Pts',(9.62553662153839,-23.0838998256659,23.0838998256659));
#47232=CARTESIAN_POINT('Ctrl Pts',(9.62553662153839,-23.0838998256659,0.));
#47233=CARTESIAN_POINT('Ctrl Pts',(9.62553662153839,-23.0838998256659,-23.0838998256659));
#47234=CARTESIAN_POINT('Ctrl Pts',(9.62553662153839,0.,-23.0838998256659));
#47235=CARTESIAN_POINT('Ctrl Pts',(9.62553662153839,23.0838998256659,-23.0838998256659));
#47236=CARTESIAN_POINT('Ctrl Pts',(9.62553662153839,23.0838998256659,0.));
#47237=CARTESIAN_POINT('Ctrl Pts',(8.75359166551105,24.5886478127263,0.));
#47238=CARTESIAN_POINT('Ctrl Pts',(8.75359166551105,24.5886478127262,24.5886478127262));
#47239=CARTESIAN_POINT('Ctrl Pts',(8.75359166551105,0.,24.5886478127263));
#47240=CARTESIAN_POINT('Ctrl Pts',(8.75359166551105,-24.5886478127262,24.5886478127262));
#47241=CARTESIAN_POINT('Ctrl Pts',(8.75359166551105,-24.5886478127263,0.));
#47242=CARTESIAN_POINT('Ctrl Pts',(8.75359166551105,-24.5886478127262,-24.5886478127262));
#47243=CARTESIAN_POINT('Ctrl Pts',(8.75359166551105,0.,-24.5886478127263));
#47244=CARTESIAN_POINT('Ctrl Pts',(8.75359166551105,24.5886478127262,-24.5886478127262));
#47245=CARTESIAN_POINT('Ctrl Pts',(8.75359166551105,24.5886478127263,0.));
#47246=CARTESIAN_POINT('Ctrl Pts',(7.92870053877921,26.1164647205758,0.));
#47247=CARTESIAN_POINT('Ctrl Pts',(7.92870053877921,26.1164647205758,26.1164647205758));
#47248=CARTESIAN_POINT('Ctrl Pts',(7.92870053877921,0.,26.1164647205758));
#47249=CARTESIAN_POINT('Ctrl Pts',(7.92870053877921,-26.1164647205758,26.1164647205758));
#47250=CARTESIAN_POINT('Ctrl Pts',(7.92870053877921,-26.1164647205758,0.));
#47251=CARTESIAN_POINT('Ctrl Pts',(7.92870053877921,-26.1164647205758,-26.1164647205758));
#47252=CARTESIAN_POINT('Ctrl Pts',(7.92870053877921,0.,-26.1164647205758));
#47253=CARTESIAN_POINT('Ctrl Pts',(7.92870053877921,26.1164647205758,-26.1164647205758));
#47254=CARTESIAN_POINT('Ctrl Pts',(7.92870053877921,26.1164647205758,0.));
#47255=CARTESIAN_POINT('Ctrl Pts',(7.14689760675259,27.6690738550248,0.));
#47256=CARTESIAN_POINT('Ctrl Pts',(7.14689760675259,27.6690738550248,27.6690738550248));
#47257=CARTESIAN_POINT('Ctrl Pts',(7.1468976067526,0.,27.6690738550248));
#47258=CARTESIAN_POINT('Ctrl Pts',(7.1468976067526,-27.6690738550248,27.6690738550248));
#47259=CARTESIAN_POINT('Ctrl Pts',(7.1468976067526,-27.6690738550248,0.));
#47260=CARTESIAN_POINT('Ctrl Pts',(7.1468976067526,-27.6690738550248,-27.6690738550248));
#47261=CARTESIAN_POINT('Ctrl Pts',(7.1468976067526,0.,-27.6690738550248));
#47262=CARTESIAN_POINT('Ctrl Pts',(7.14689760675259,27.6690738550248,-27.6690738550248));
#47263=CARTESIAN_POINT('Ctrl Pts',(7.14689760675259,27.6690738550248,0.));
#47264=CARTESIAN_POINT('Ctrl Pts',(6.40416480933221,29.248955946805,0.));
#47265=CARTESIAN_POINT('Ctrl Pts',(6.40416480933221,29.248955946805,29.248955946805));
#47266=CARTESIAN_POINT('Ctrl Pts',(6.40416480933221,0.,29.248955946805));
#47267=CARTESIAN_POINT('Ctrl Pts',(6.40416480933221,-29.248955946805,29.248955946805));
#47268=CARTESIAN_POINT('Ctrl Pts',(6.40416480933221,-29.248955946805,0.));
#47269=CARTESIAN_POINT('Ctrl Pts',(6.40416480933221,-29.248955946805,-29.248955946805));
#47270=CARTESIAN_POINT('Ctrl Pts',(6.40416480933221,0.,-29.248955946805));
#47271=CARTESIAN_POINT('Ctrl Pts',(6.40416480933221,29.248955946805,-29.248955946805));
#47272=CARTESIAN_POINT('Ctrl Pts',(6.40416480933221,29.248955946805,0.));
#47273=CARTESIAN_POINT('Ctrl Pts',(5.69731071687183,30.8577859595634,0.));
#47274=CARTESIAN_POINT('Ctrl Pts',(5.69731071687183,30.8577859595634,30.8577859595634));
#47275=CARTESIAN_POINT('Ctrl Pts',(5.69731071687183,0.,30.8577859595634));
#47276=CARTESIAN_POINT('Ctrl Pts',(5.69731071687183,-30.8577859595634,30.8577859595634));
#47277=CARTESIAN_POINT('Ctrl Pts',(5.69731071687183,-30.8577859595634,0.));
#47278=CARTESIAN_POINT('Ctrl Pts',(5.69731071687183,-30.8577859595634,-30.8577859595634));
#47279=CARTESIAN_POINT('Ctrl Pts',(5.69731071687183,0.,-30.8577859595634));
#47280=CARTESIAN_POINT('Ctrl Pts',(5.69731071687183,30.8577859595634,-30.8577859595634));
#47281=CARTESIAN_POINT('Ctrl Pts',(5.69731071687183,30.8577859595634,0.));
#47282=CARTESIAN_POINT('Ctrl Pts',(5.02401496259691,32.4964011792533,0.));
#47283=CARTESIAN_POINT('Ctrl Pts',(5.02401496259691,32.4964011792533,32.4964011792533));
#47284=CARTESIAN_POINT('Ctrl Pts',(5.02401496259691,0.,32.4964011792533));
#47285=CARTESIAN_POINT('Ctrl Pts',(5.02401496259691,-32.4964011792533,32.4964011792533));
#47286=CARTESIAN_POINT('Ctrl Pts',(5.02401496259691,-32.4964011792533,0.));
#47287=CARTESIAN_POINT('Ctrl Pts',(5.02401496259691,-32.4964011792533,-32.4964011792533));
#47288=CARTESIAN_POINT('Ctrl Pts',(5.02401496259691,0.,-32.4964011792533));
#47289=CARTESIAN_POINT('Ctrl Pts',(5.02401496259691,32.4964011792533,-32.4964011792533));
#47290=CARTESIAN_POINT('Ctrl Pts',(5.02401496259691,32.4964011792533,0.));
#47291=CARTESIAN_POINT('Ctrl Pts',(4.38267277981043,34.1651137045816,0.));
#47292=CARTESIAN_POINT('Ctrl Pts',(4.38267277981043,34.1651137045815,34.1651137045815));
#47293=CARTESIAN_POINT('Ctrl Pts',(4.38267277981043,0.,34.1651137045816));
#47294=CARTESIAN_POINT('Ctrl Pts',(4.38267277981043,-34.1651137045815,34.1651137045815));
#47295=CARTESIAN_POINT('Ctrl Pts',(4.38267277981043,-34.1651137045816,0.));
#47296=CARTESIAN_POINT('Ctrl Pts',(4.38267277981043,-34.1651137045815,-34.1651137045815));
#47297=CARTESIAN_POINT('Ctrl Pts',(4.38267277981043,0.,-34.1651137045816));
#47298=CARTESIAN_POINT('Ctrl Pts',(4.38267277981043,34.1651137045815,-34.1651137045815));
#47299=CARTESIAN_POINT('Ctrl Pts',(4.38267277981043,34.1651137045816,0.));
#47300=CARTESIAN_POINT('Ctrl Pts',(3.89437496746067,35.5241326822989,0.));
#47301=CARTESIAN_POINT('Ctrl Pts',(3.89437496746067,35.5241326822989,35.5241326822989));
#47302=CARTESIAN_POINT('Ctrl Pts',(3.89437496746067,0.,35.5241326822989));
#47303=CARTESIAN_POINT('Ctrl Pts',(3.89437496746066,-35.5241326822989,35.5241326822989));
#47304=CARTESIAN_POINT('Ctrl Pts',(3.89437496746066,-35.5241326822989,0.));
#47305=CARTESIAN_POINT('Ctrl Pts',(3.89437496746066,-35.5241326822989,-35.5241326822989));
#47306=CARTESIAN_POINT('Ctrl Pts',(3.89437496746067,0.,-35.5241326822989));
#47307=CARTESIAN_POINT('Ctrl Pts',(3.89437496746067,35.5241326822989,-35.5241326822989));
#47308=CARTESIAN_POINT('Ctrl Pts',(3.89437496746067,35.5241326822989,0.));
#47309=CARTESIAN_POINT('Ctrl Pts',(3.5418673953418,36.5568488026925,0.));
#47310=CARTESIAN_POINT('Ctrl Pts',(3.5418673953418,36.5568488026925,36.5568488026925));
#47311=CARTESIAN_POINT('Ctrl Pts',(3.5418673953418,0.,36.5568488026925));
#47312=CARTESIAN_POINT('Ctrl Pts',(3.5418673953418,-36.5568488026925,36.5568488026925));
#47313=CARTESIAN_POINT('Ctrl Pts',(3.5418673953418,-36.5568488026925,0.));
#47314=CARTESIAN_POINT('Ctrl Pts',(3.5418673953418,-36.5568488026925,-36.5568488026925));
#47315=CARTESIAN_POINT('Ctrl Pts',(3.5418673953418,0.,-36.5568488026925));
#47316=CARTESIAN_POINT('Ctrl Pts',(3.5418673953418,36.5568488026925,-36.5568488026925));
#47317=CARTESIAN_POINT('Ctrl Pts',(3.5418673953418,36.5568488026925,0.));
#47318=CARTESIAN_POINT('Ctrl Pts',(3.31294245015623,37.2512891119684,0.));
#47319=CARTESIAN_POINT('Ctrl Pts',(3.31294245015623,37.2512891119684,37.2512891119684));
#47320=CARTESIAN_POINT('Ctrl Pts',(3.31294245015623,0.,37.2512891119684));
#47321=CARTESIAN_POINT('Ctrl Pts',(3.31294245015623,-37.2512891119684,37.2512891119684));
#47322=CARTESIAN_POINT('Ctrl Pts',(3.31294245015623,-37.2512891119684,0.));
#47323=CARTESIAN_POINT('Ctrl Pts',(3.31294245015623,-37.2512891119684,-37.2512891119684));
#47324=CARTESIAN_POINT('Ctrl Pts',(3.31294245015623,0.,-37.2512891119684));
#47325=CARTESIAN_POINT('Ctrl Pts',(3.31294245015623,37.2512891119684,-37.2512891119684));
#47326=CARTESIAN_POINT('Ctrl Pts',(3.31294245015623,37.2512891119684,0.));
#47327=CARTESIAN_POINT('Ctrl Pts',(3.2,37.6,0.));
#47328=CARTESIAN_POINT('Ctrl Pts',(3.2,37.6,37.6));
#47329=CARTESIAN_POINT('Ctrl Pts',(3.2,0.,37.6));
#47330=CARTESIAN_POINT('Ctrl Pts',(3.2,-37.6,37.6));
#47331=CARTESIAN_POINT('Ctrl Pts',(3.2,-37.6,0.));
#47332=CARTESIAN_POINT('Ctrl Pts',(3.2,-37.6,-37.6));
#47333=CARTESIAN_POINT('Ctrl Pts',(3.2,0.,-37.6));
#47334=CARTESIAN_POINT('Ctrl Pts',(3.2,37.6,-37.6));
#47335=CARTESIAN_POINT('Ctrl Pts',(3.2,37.6,0.));
#47336=CARTESIAN_POINT('',(11.1111871729018,20.775057671175,0.));
#47337=CARTESIAN_POINT('',(23.5150942984749,10.0178765673373,0.));
#47338=CARTESIAN_POINT('Ctrl Pts',(11.1111871729018,20.775057671175,0.));
#47339=CARTESIAN_POINT('Ctrl Pts',(11.1948689745378,20.6509039312648,0.));
#47340=CARTESIAN_POINT('Ctrl Pts',(11.4755829737079,20.2377304421578,0.));
#47341=CARTESIAN_POINT('Ctrl Pts',(11.9616798526703,19.5410850083761,0.));
#47342=CARTESIAN_POINT('Ctrl Pts',(12.6687572718921,18.5736371717314,0.));
#47343=CARTESIAN_POINT('Ctrl Pts',(13.6172459538847,17.362757468191,0.));
#47344=CARTESIAN_POINT('Ctrl Pts',(14.7267277676362,16.0674034956045,0.));
#47345=CARTESIAN_POINT('Ctrl Pts',(15.8649034353727,14.8662985491428,0.));
#47346=CARTESIAN_POINT('Ctrl Pts',(17.0210036637821,13.7799946040807,0.));
#47347=CARTESIAN_POINT('Ctrl Pts',(18.1843885347784,12.8237912132616,0.));
#47348=CARTESIAN_POINT('Ctrl Pts',(19.3456615791409,12.0038530129696,0.));
#47349=CARTESIAN_POINT('Ctrl Pts',(20.4975894383762,11.3145134298179,0.));
#47350=CARTESIAN_POINT('Ctrl Pts',(21.5658679574808,10.7776397148383,0.));
#47351=CARTESIAN_POINT('Ctrl Pts',(22.3939741610711,10.4247254993888,0.));
#47352=CARTESIAN_POINT('Ctrl Pts',(22.9904947752284,10.1993474973472,0.));
#47353=CARTESIAN_POINT('Ctrl Pts',(23.3627187655144,10.0693419338606,0.));
#47354=CARTESIAN_POINT('Ctrl Pts',(23.5150942984749,10.0178765673373,0.));
#47355=CARTESIAN_POINT('',(3.2,37.5892271801377,0.899999999999997));
#47356=CARTESIAN_POINT('Ctrl Pts',(11.1111871729018,20.775057671175,4.68375338513738E-16));
#47357=CARTESIAN_POINT('Ctrl Pts',(10.8408519694691,21.1761380241238,0.104779981433169));
#47358=CARTESIAN_POINT('Ctrl Pts',(10.5713373596261,21.5873718624941,0.200619231177909));
#47359=CARTESIAN_POINT('Ctrl Pts',(10.2958331164458,22.0215373473783,0.285388879148048));
#47360=CARTESIAN_POINT('Ctrl Pts',(9.71429910913615,22.9379733025773,0.464320544639868));
#47361=CARTESIAN_POINT('Ctrl Pts',(9.09451803370737,23.9735296287181,0.601171200169489));
#47362=CARTESIAN_POINT('Ctrl Pts',(8.43051482342505,25.1910871092345,0.711313606025344));
#47363=CARTESIAN_POINT('Ctrl Pts',(7.97885593463559,26.019276868217,0.786233118261289));
#47364=CARTESIAN_POINT('Ctrl Pts',(7.52255926008875,26.9071640425416,0.845450887989925));
#47365=CARTESIAN_POINT('Ctrl Pts',(7.10363554125515,27.7707039763416,0.894013240723397));
#47366=CARTESIAN_POINT('Ctrl Pts',(6.56327799557425,28.8845590727416,0.956652409994373));
#47367=CARTESIAN_POINT('Ctrl Pts',(6.08559840027184,29.9474764438374,0.961734555176139));
#47368=CARTESIAN_POINT('Ctrl Pts',(5.6170867083501,31.0600288611027,0.951686011835693));
#47369=CARTESIAN_POINT('Ctrl Pts',(5.04102956507642,32.4279643433598,0.939330855559837));
#47370=CARTESIAN_POINT('Ctrl Pts',(4.5010282050509,33.8266980954716,0.9));
#47371=CARTESIAN_POINT('Ctrl Pts',(4.,35.2340925362767,0.9));
#47372=CARTESIAN_POINT('Ctrl Pts',(3.72183418896969,36.0154637487543,0.9));
#47373=CARTESIAN_POINT('Ctrl Pts',(3.45538353518196,36.8005021100802,0.9));
#47374=CARTESIAN_POINT('Ctrl Pts',(3.2,37.5892271801377,0.9));
#47375=CARTESIAN_POINT('',(3.2,34.2572188230213,15.4984824583453));
#47376=CARTESIAN_POINT('Origin',(3.2,0.,0.));
#47377=CARTESIAN_POINT('',(15.,15.4997804972258,3.06084967694561));
#47378=CARTESIAN_POINT('Ctrl Pts',(3.2,34.2572188230213,15.4984824583453));
#47379=CARTESIAN_POINT('Ctrl Pts',(3.56152274835418,33.2512647221728,15.0140404956913));
#47380=CARTESIAN_POINT('Ctrl Pts',(3.95224584525374,32.2350723867225,14.5182294335367));
#47381=CARTESIAN_POINT('Ctrl Pts',(4.78767430123722,30.1964778916196,13.5611205349435));
#47382=CARTESIAN_POINT('Ctrl Pts',(5.21513946232063,29.2140021162723,13.1170571755916));
#47383=CARTESIAN_POINT('Ctrl Pts',(6.79548775402531,25.836168792914,11.5276347803711));
#47384=CARTESIAN_POINT('Ctrl Pts',(7.94016295939284,23.9218153262741,10.3912034265391));
#47385=CARTESIAN_POINT('Ctrl Pts',(9.46271935275732,21.5720888915642,8.90666589894935));
#47386=CARTESIAN_POINT('Ctrl Pts',(10.1385443659094,20.6585071274117,8.21538544795477));
#47387=CARTESIAN_POINT('Ctrl Pts',(11.5967860400733,18.9239680936141,6.63484019277982));
#47388=CARTESIAN_POINT('Ctrl Pts',(12.3997356677083,18.0341377754366,5.78619942648488));
#47389=CARTESIAN_POINT('Ctrl Pts',(13.6850585208097,16.7156528118604,4.43617268008764));
#47390=CARTESIAN_POINT('Ctrl Pts',(14.3457395898608,16.0917172728797,3.72217451879281));
#47391=CARTESIAN_POINT('Ctrl Pts',(15.,15.4997804972258,3.06084967694561));
#47392=CARTESIAN_POINT('',(15.,14.914658515121,5.2120013031819));
#47393=CARTESIAN_POINT('Ctrl Pts',(15.,15.4997804972258,3.06084967694561));
#47394=CARTESIAN_POINT('Ctrl Pts',(15.,15.3557790740222,3.79005584076192));
#47395=CARTESIAN_POINT('Ctrl Pts',(15.,15.1603519478033,4.50892518429681));
#47396=CARTESIAN_POINT('Ctrl Pts',(15.,14.914658515121,5.2120013031819));
#47397=CARTESIAN_POINT('',(3.2,33.4762280926097,17.1202264205697));
#47398=CARTESIAN_POINT('Ctrl Pts',(15.,14.914658515121,5.2120013031819));
#47399=CARTESIAN_POINT('Ctrl Pts',(14.4897165779508,15.3292352555695,5.70151627419433));
#47400=CARTESIAN_POINT('Ctrl Pts',(13.9833803026607,15.7672104557508,6.19304081265193));
#47401=CARTESIAN_POINT('Ctrl Pts',(13.4460287676664,16.2769406731723,6.70286203098642));
#47402=CARTESIAN_POINT('Ctrl Pts',(12.8282655681005,16.8629491788207,7.28897515532747));
#47403=CARTESIAN_POINT('Ctrl Pts',(12.1555414089416,17.5447613593883,7.96966355059842));
#47404=CARTESIAN_POINT('Ctrl Pts',(11.5904908073494,18.1719403594245,8.53563819264853));
#47405=CARTESIAN_POINT('Ctrl Pts',(11.1143368259575,18.7004483852033,9.01257083977716));
#47406=CARTESIAN_POINT('Ctrl Pts',(10.6953158949575,19.2030248825086,9.42802203261975));
#47407=CARTESIAN_POINT('Ctrl Pts',(10.2957959918397,19.7169417339605,9.81194913646659));
#47408=CARTESIAN_POINT('Ctrl Pts',(10.0450888109627,20.0394354170716,10.0528715063325));
#47409=CARTESIAN_POINT('Ctrl Pts',(9.80235305585738,20.365996759971,10.2821249831681));
#47410=CARTESIAN_POINT('Ctrl Pts',(9.5601010623963,20.7052519349419,10.5098647441811));
#47411=CARTESIAN_POINT('Ctrl Pts',(9.36613602949014,20.9768849573855,10.6922102002816));
#47412=CARTESIAN_POINT('Ctrl Pts',(9.15248571309183,21.2835959554689,10.8921233525791));
#47413=CARTESIAN_POINT('Ctrl Pts',(8.89022359845111,21.6785168619804,11.1382095281044));
#47414=CARTESIAN_POINT('Ctrl Pts',(8.39222406123487,22.4284171247353,11.605493190843));
#47415=CARTESIAN_POINT('Ctrl Pts',(7.76643777383336,23.4350262792015,12.1927153023679));
#47416=CARTESIAN_POINT('Ctrl Pts',(7.10363554123529,24.6326419147479,12.8547349765861));
#47417=CARTESIAN_POINT('Ctrl Pts',(6.23550018249919,26.2012734435196,13.7218453439034));
#47418=CARTESIAN_POINT('Ctrl Pts',(5.31040885825212,28.1564047394871,14.6002024056743));
#47419=CARTESIAN_POINT('Ctrl Pts',(4.46416616907914,30.2050861982221,15.5549203579907));
#47420=CARTESIAN_POINT('Ctrl Pts',(4.30741751126835,30.5845613453012,15.7317617765674));
#47421=CARTESIAN_POINT('Ctrl Pts',(4.15262292090198,30.9680620164154,15.9123572985204));
#47422=CARTESIAN_POINT('Ctrl Pts',(4.,31.3543250987725,16.098371795166));
#47423=CARTESIAN_POINT('Ctrl Pts',(3.7243497328338,32.0519498147649,16.4343301518407));
#47424=CARTESIAN_POINT('Ctrl Pts',(3.45587123478804,32.7642543119943,16.7773579185688));
#47425=CARTESIAN_POINT('Ctrl Pts',(3.2,33.4762280926097,17.1202264205697));
#47426=CARTESIAN_POINT('',(3.2,24.1401481407882,28.8273003894017));
#47427=CARTESIAN_POINT('Origin',(3.2,0.,0.));
#47428=CARTESIAN_POINT('Ctrl Pts',(3.2,24.1401481407882,28.8273003894017));
#47429=CARTESIAN_POINT('Ctrl Pts',(3.4517402012824,23.6554016427293,28.219447507015));
#47430=CARTESIAN_POINT('Ctrl Pts',(3.71840125357238,23.1649351015154,27.6044219173822));
#47431=CARTESIAN_POINT('Ctrl Pts',(4.,22.6717457083367,26.9859819793801));
#47432=CARTESIAN_POINT('Ctrl Pts',(4.62816481487921,21.5715837658681,25.6064225385185));
#47433=CARTESIAN_POINT('Ctrl Pts',(5.32582967773128,20.4257443465207,24.2662709294862));
#47434=CARTESIAN_POINT('Ctrl Pts',(6.03866109153771,19.4167181280198,22.9927130590511));
#47435=CARTESIAN_POINT('Ctrl Pts',(6.32798218739597,19.0071786974727,22.4758066046264));
#47436=CARTESIAN_POINT('Ctrl Pts',(6.6160411706376,18.6257941155792,21.9750548900751));
#47437=CARTESIAN_POINT('Ctrl Pts',(6.89476148100327,18.2850710138973,21.4951682830474));
#47438=CARTESIAN_POINT('Ctrl Pts',(7.65522892714578,17.3554336055655,20.185833695964));
#47439=CARTESIAN_POINT('Ctrl Pts',(8.3522670912656,16.6384040964243,19.1007390031585));
#47440=CARTESIAN_POINT('Ctrl Pts',(8.78926323660369,16.2240019202544,18.4274271814668));
#47441=CARTESIAN_POINT('Ctrl Pts',(8.99031958013673,16.0333407732816,18.1176450143445));
#47442=CARTESIAN_POINT('Ctrl Pts',(9.1827552232782,15.859968720011,17.8244630669136));
#47443=CARTESIAN_POINT('Ctrl Pts',(9.37496046323339,15.6959599143301,17.5328830843302));
#47444=CARTESIAN_POINT('Ctrl Pts',(9.48075233467205,15.6056876694659,17.3723942649893));
#47445=CARTESIAN_POINT('Ctrl Pts',(9.58626090989787,15.5184988415833,17.2127346999996));
#47446=CARTESIAN_POINT('Ctrl Pts',(9.69257910363365,15.433779824459,17.0518540733511));
#47447=CARTESIAN_POINT('Ctrl Pts',(10.0319880473342,15.1633238366068,16.5382606644157));
#47448=CARTESIAN_POINT('Ctrl Pts',(10.3788056747491,14.9187807821475,16.0114307331727));
#47449=CARTESIAN_POINT('Ctrl Pts',(10.7756849089348,14.6687048722873,15.4154473578682));
#47450=CARTESIAN_POINT('Ctrl Pts',(10.8890930409408,14.5972457498288,15.2451452723016));
#47451=CARTESIAN_POINT('Ctrl Pts',(11.057620352753,14.4933604902702,14.9923498534867));
#47452=CARTESIAN_POINT('Ctrl Pts',(11.2725125499177,14.3686609268079,14.6736882151435));
#47453=CARTESIAN_POINT('Ctrl Pts',(11.5968279597855,14.180464284174,14.1927639135076));
#47454=CARTESIAN_POINT('Ctrl Pts',(12.0255678846111,13.9481586925854,13.5614890403409));
#47455=CARTESIAN_POINT('Ctrl Pts',(12.532035905153,13.6869042147774,12.8549105632904));
#47456=CARTESIAN_POINT('Ctrl Pts',(13.0988763176265,13.3945074790411,12.0641059732044));
#47457=CARTESIAN_POINT('Ctrl Pts',(13.7495416915397,13.1167044041393,11.1526887031812));
#47458=CARTESIAN_POINT('Ctrl Pts',(14.4398764939332,12.8499149844562,10.2249013726919));
#47459=CARTESIAN_POINT('Ctrl Pts',(14.7901814035672,12.714534813517,9.75410306462509));
#47460=CARTESIAN_POINT('Ctrl Pts',(15.1459546150644,12.5820394706047,9.28856386081903));
#47461=CARTESIAN_POINT('Ctrl Pts',(15.4570717747561,12.4649063243577,8.89690991431743));
#47462=CARTESIAN_POINT('Ctrl Pts',(15.799823141116,12.3358631498765,8.46543282884673));
#47463=CARTESIAN_POINT('Ctrl Pts',(16.0676294503676,12.2436583506951,8.13029753852379));
#47464=CARTESIAN_POINT('Ctrl Pts',(16.3615307987862,12.1462490787105,7.7659519476552));
#47465=CARTESIAN_POINT('Ctrl Pts',(17.0296616033239,11.9248069668907,6.93767907967872));
#47466=CARTESIAN_POINT('Ctrl Pts',(17.7084691879561,11.7252415447452,6.11143371863158));
#47467=CARTESIAN_POINT('Ctrl Pts',(18.4207032016838,11.5097253054852,5.31931102580207));
#47468=CARTESIAN_POINT('Ctrl Pts',(18.8298642042877,11.3859165027133,4.8642559330424));
#47469=CARTESIAN_POINT('Ctrl Pts',(19.2113759273418,11.2794672006796,4.44103900795681));
#47470=CARTESIAN_POINT('Ctrl Pts',(19.5701113608397,11.1806982910754,4.04710221245386));
#47471=CARTESIAN_POINT('Ctrl Pts',(20.1215476022134,11.0288739905159,3.44155560187016));
#47472=CARTESIAN_POINT('Ctrl Pts',(20.6514912601619,10.888905473324,2.85828734179492));
#47473=CARTESIAN_POINT('Ctrl Pts',(21.3979544325339,10.6719534577984,2.10691159324049));
#47474=CARTESIAN_POINT('Ctrl Pts',(21.8015299361149,10.5546582955463,1.70068010409967));
#47475=CARTESIAN_POINT('Ctrl Pts',(22.2842895882516,10.4128463661915,1.22286894239258));
#47476=CARTESIAN_POINT('Ctrl Pts',(22.8110928915501,10.2470312028678,0.700625669077338));
#47477=CARTESIAN_POINT('Ctrl Pts',(23.0435286867255,10.1738703492856,0.470201847229612));
#47478=CARTESIAN_POINT('Ctrl Pts',(23.2793380077566,10.0975040749578,0.235994067598351));
#47479=CARTESIAN_POINT('Ctrl Pts',(23.5150942984749,10.0178765673373,2.74086309204336E-15));
#47480=CARTESIAN_POINT('Origin',(2.44847982464479,0.,-1.17996027893162E-15));
#47481=CARTESIAN_POINT('',(2.79695964929223,35.1047516110625,-15.9066327376731));
#47482=CARTESIAN_POINT('',(2.1,35.5189237522517,-16.106087528687));
#47483=CARTESIAN_POINT('Ctrl Pts',(2.09999999999999,35.5189237522517,-16.106087528687));
#47484=CARTESIAN_POINT('Ctrl Pts',(2.33231184614132,35.3808715864332,-16.0396051095574));
#47485=CARTESIAN_POINT('Ctrl Pts',(2.56464811456314,35.2428044741992,-15.9731154926135));
#47486=CARTESIAN_POINT('Ctrl Pts',(2.79695964929243,35.1047516110636,-15.9066327376736));
#47487=CARTESIAN_POINT('',(2.1,38.98961400168,-0.9));
#47488=CARTESIAN_POINT('Origin',(2.1,0.,0.));
#47489=CARTESIAN_POINT('',(2.79695964929243,38.5299176060057,-0.900000000000078));
#47490=CARTESIAN_POINT('Ctrl Pts',(2.79695964929245,38.5299176060072,-0.9));
#47491=CARTESIAN_POINT('Ctrl Pts',(2.56464811234863,38.6831447255779,-0.9));
#47492=CARTESIAN_POINT('Ctrl Pts',(2.33231184158428,38.8363876605392,-0.9));
#47493=CARTESIAN_POINT('Ctrl Pts',(2.09999999999999,38.98961400168,-0.9));
#47494=CARTESIAN_POINT('Origin',(2.79695964928958,0.,-2.35992055786324E-15));
#47495=CARTESIAN_POINT('Origin',(1.55,0.,0.));
#47496=CARTESIAN_POINT('',(2.6,38.98961400168,-0.899999999999993));
#47497=CARTESIAN_POINT('Ctrl Pts',(2.1,38.98961400168,-0.9));
#47498=CARTESIAN_POINT('Ctrl Pts',(2.26666666666667,38.98961400168,-0.9));
#47499=CARTESIAN_POINT('Ctrl Pts',(2.43346002867001,38.9896159908677,-0.899989754761565));
#47500=CARTESIAN_POINT('Ctrl Pts',(2.60034430332035,38.9896190555114,-0.899974049656302));
#47501=CARTESIAN_POINT('',(2.6,35.5189237522517,-16.106087528687));
#47502=CARTESIAN_POINT('Ctrl Pts',(2.59962081372057,35.5189106691499,-16.1061069197962));
#47503=CARTESIAN_POINT('Ctrl Pts',(2.43319306186644,35.5189185929367,-16.1060951831224));
#47504=CARTESIAN_POINT('Ctrl Pts',(2.26666666666667,35.5189237522517,-16.106087528687));
#47505=CARTESIAN_POINT('Ctrl Pts',(2.1,35.5189237522517,-16.106087528687));
#47506=CARTESIAN_POINT('',(6.,35.548403009865,-16.0409177869666));
#47507=CARTESIAN_POINT('Ctrl Pts',(2.6,35.5189237522517,-16.106087528687));
#47508=CARTESIAN_POINT('Ctrl Pts',(3.15786519714955,35.5189237522517,-16.106087528687));
#47509=CARTESIAN_POINT('Ctrl Pts',(3.71593098901213,35.5143077475111,-16.1162704800869));
#47510=CARTESIAN_POINT('Ctrl Pts',(4.82421019263741,35.5267242579696,-16.0888808412897));
#47511=CARTESIAN_POINT('Ctrl Pts',(5.40687161376251,35.548282527766,-16.0411847882857));
#47512=CARTESIAN_POINT('Ctrl Pts',(6.,35.548403009865,-16.0409177869666));
#47513=CARTESIAN_POINT('',(6.,34.7703877941326,-17.6640916167698));
#47514=CARTESIAN_POINT('Origin',(6.,0.,0.));
#47515=CARTESIAN_POINT('',(2.6,34.7379330218401,-17.7278314909114));
#47516=CARTESIAN_POINT('Ctrl Pts',(6.,34.7703877941326,-17.6640916167698));
#47517=CARTESIAN_POINT('Ctrl Pts',(5.46151291267476,34.7702417512009,-17.6643790908997));
#47518=CARTESIAN_POINT('Ctrl Pts',(4.90416494331291,34.7471941155784,-17.709679558335));
#47519=CARTESIAN_POINT('Ctrl Pts',(3.74812575287323,34.7329579415584,-17.7375836670634));
#47520=CARTESIAN_POINT('Ctrl Pts',(3.17396064416408,34.7379330218401,-17.7278314909114));
#47521=CARTESIAN_POINT('Ctrl Pts',(2.6,34.7379330218401,-17.7278314909114));
#47522=CARTESIAN_POINT('',(2.1,34.7379330218401,-17.7278314909114));
#47523=CARTESIAN_POINT('Ctrl Pts',(2.1,34.7379330218401,-17.7278314909114));
#47524=CARTESIAN_POINT('Ctrl Pts',(2.26666666666667,34.7379330218401,-17.7278314909114));
#47525=CARTESIAN_POINT('Ctrl Pts',(2.4335782958255,34.7379353669068,-17.727828473026));
#47526=CARTESIAN_POINT('Ctrl Pts',(2.60065276820886,34.7379392432415,-17.7278233384529));
#47527=CARTESIAN_POINT('',(2.1,25.0132750426772,-29.9221668941169));
#47528=CARTESIAN_POINT('Origin',(2.1,0.,0.));
#47529=CARTESIAN_POINT('',(2.6,25.0132750426772,-29.9221668941169));
#47530=CARTESIAN_POINT('Ctrl Pts',(2.59963671643924,25.0132558670369,-29.9221762868835));
#47531=CARTESIAN_POINT('Ctrl Pts',(2.43319919569241,25.013267470382,-29.9221706110259));
#47532=CARTESIAN_POINT('Ctrl Pts',(2.26666666666667,25.0132750426772,-29.9221668941169));
#47533=CARTESIAN_POINT('Ctrl Pts',(2.1,25.0132750426772,-29.9221668941169));
#47534=CARTESIAN_POINT('',(6.,25.0681110272506,-29.8762415562171));
#47535=CARTESIAN_POINT('Ctrl Pts',(2.6,25.0132750426772,-29.9221668941169));
#47536=CARTESIAN_POINT('Ctrl Pts',(3.15786555369928,25.0132750426772,-29.9221668941169));
#47537=CARTESIAN_POINT('Ctrl Pts',(3.71593170347639,25.0046979272054,-29.9293386252219));
#47538=CARTESIAN_POINT('Ctrl Pts',(4.82421093519821,25.027768809093,-29.9100486737611));
#47539=CARTESIAN_POINT('Ctrl Pts',(5.40687201153467,25.0678866292501,-29.8764298407435));
#47540=CARTESIAN_POINT('Ctrl Pts',(6.,25.0681110272506,-29.8762415562171));
#47541=CARTESIAN_POINT('',(6.,23.6628748086085,-31.0011024931715));
#47542=CARTESIAN_POINT('Origin',(6.,0.,0.));
#47543=CARTESIAN_POINT('',(2.6,23.6059783742347,-31.0444485374626));
#47544=CARTESIAN_POINT('Ctrl Pts',(6.,23.6628748086085,-31.0011024931715));
#47545=CARTESIAN_POINT('Ctrl Pts',(5.46151292711359,23.6626184981302,-31.0012981327543));
#47546=CARTESIAN_POINT('Ctrl Pts',(4.90416497508538,23.6221981620287,-31.0321124475678));
#47547=CARTESIAN_POINT('Ctrl Pts',(3.7481257854858,23.5972646702696,-31.0510763387916));
#47548=CARTESIAN_POINT('Ctrl Pts',(3.17396066044241,23.6059783742347,-31.0444485374626));
#47549=CARTESIAN_POINT('Ctrl Pts',(2.6,23.6059783742347,-31.0444485374626));
#47550=CARTESIAN_POINT('',(2.1,23.6059783742347,-31.0444485374626));
#47551=CARTESIAN_POINT('Ctrl Pts',(2.1,23.6059783742347,-31.0444485374626));
#47552=CARTESIAN_POINT('Ctrl Pts',(2.26666666666667,23.6059783742347,-31.0444485374626));
#47553=CARTESIAN_POINT('Ctrl Pts',(2.43346490340496,23.6059860909079,-31.0444445811933));
#47554=CARTESIAN_POINT('Ctrl Pts',(2.60035670167875,23.6059979144327,-31.0444385373999));
#47555=CARTESIAN_POINT('',(2.1,9.55344044321366,-37.8117941348724));
#47556=CARTESIAN_POINT('Origin',(2.1,0.,0.));
#47557=CARTESIAN_POINT('',(2.6,9.55344044321365,-37.8117941348724));
#47558=CARTESIAN_POINT('Ctrl Pts',(2.59961800914399,9.55341844221435,-37.8117958094788));
#47559=CARTESIAN_POINT('Ctrl Pts',(2.43319197104145,9.5534317600474,-37.8117948001723));
#47560=CARTESIAN_POINT('Ctrl Pts',(2.26666666666667,9.55344044321366,-37.8117941348724));
#47561=CARTESIAN_POINT('Ctrl Pts',(2.1,9.55344044321366,-37.8117941348724));
#47562=CARTESIAN_POINT('',(6.,9.62277221548328,-37.7942092772018));
#47563=CARTESIAN_POINT('Ctrl Pts',(2.6,9.55344044321366,-37.8117941348724));
#47564=CARTESIAN_POINT('Ctrl Pts',(3.15786519714955,9.55344044321366,-37.8117941348724));
#47565=CARTESIAN_POINT('Ctrl Pts',(3.71593098901213,9.54260105934372,-37.8145341633936));
#47566=CARTESIAN_POINT('Ctrl Pts',(4.82421019263741,9.57175670889429,-37.8071646217058));
#47567=CARTESIAN_POINT('Ctrl Pts',(5.40687161376251,9.62248834608612,-37.7942815531033));
#47568=CARTESIAN_POINT('Ctrl Pts',(6.,9.62277221548328,-37.7942092772018));
#47569=CARTESIAN_POINT('',(6.,7.86863926112478,-38.1979648172293));
#47570=CARTESIAN_POINT('Origin',(6.,0.,0.));
#47571=CARTESIAN_POINT('',(2.6,7.79857020128637,-38.2123318159938));
#47572=CARTESIAN_POINT('Ctrl Pts',(6.,7.86863926112478,-38.1979648172293));
#47573=CARTESIAN_POINT('Ctrl Pts',(5.46151291267476,7.86832344852115,-38.1980298734558));
#47574=CARTESIAN_POINT('Ctrl Pts',(4.90416494331291,7.81853615114211,-38.2082548857951));
#47575=CARTESIAN_POINT('Ctrl Pts',(3.74812575287323,7.78784373112913,-38.2145225239784));
#47576=CARTESIAN_POINT('Ctrl Pts',(3.17396064416408,7.79857020128638,-38.2123318159938));
#47577=CARTESIAN_POINT('Ctrl Pts',(2.6,7.79857020128638,-38.2123318159938));
#47578=CARTESIAN_POINT('',(2.1,7.79857020128638,-38.2123318159937));
#47579=CARTESIAN_POINT('Ctrl Pts',(2.1,7.79857020128638,-38.2123318159937));
#47580=CARTESIAN_POINT('Ctrl Pts',(2.26666666666667,7.79857020128638,-38.2123318159937));
#47581=CARTESIAN_POINT('Ctrl Pts',(2.43357876469311,7.7985739143114,-38.2123317838051));
#47582=CARTESIAN_POINT('Ctrl Pts',(2.60065399305178,7.79858017606306,-38.2123316380654));
#47583=CARTESIAN_POINT('',(2.1,-7.79857020128639,-38.2123318159937));
#47584=CARTESIAN_POINT('Origin',(2.1,0.,0.));
#47585=CARTESIAN_POINT('',(2.6,-7.79857020128639,-38.2123318159937));
#47586=CARTESIAN_POINT('Ctrl Pts',(2.59964466174317,-7.79859228682692,-38.2123216610868));
#47587=CARTESIAN_POINT('Ctrl Pts',(2.43320229863994,-7.79857892554184,-38.2123278118252));
#47588=CARTESIAN_POINT('Ctrl Pts',(2.26666666666667,-7.79857020128639,-38.2123318159937));
#47589=CARTESIAN_POINT('Ctrl Pts',(2.1,-7.79857020128639,-38.2123318159937));
#47590=CARTESIAN_POINT('',(6.,-7.72847464911698,-38.226570335278));
#47591=CARTESIAN_POINT('Ctrl Pts',(2.6,-7.79857020128639,-38.2123318159937));
#47592=CARTESIAN_POINT('Ctrl Pts',(3.15786555369928,-7.79857020128639,-38.2123318159937));
#47593=CARTESIAN_POINT('Ctrl Pts',(3.71593170347639,-7.80952503047415,-38.2100974582948));
#47594=CARTESIAN_POINT('Ctrl Pts',(4.82421093519821,-7.78005907955,-38.2161079120687));
#47595=CARTESIAN_POINT('Ctrl Pts',(5.40687201153467,-7.72876176575221,-38.2265122873386));
#47596=CARTESIAN_POINT('Ctrl Pts',(6.,-7.72847464911697,-38.226570335278));
#47597=CARTESIAN_POINT('',(6.,-9.48407679455226,-37.8292517419395));
#47598=CARTESIAN_POINT('Origin',(6.,0.,0.));
#47599=CARTESIAN_POINT('',(2.6,-9.55344044321367,-37.8117941348724));
#47600=CARTESIAN_POINT('Ctrl Pts',(6.,-9.48407679455225,-37.8292517419395));
#47601=CARTESIAN_POINT('Ctrl Pts',(5.46151292711359,-9.48438955870664,-37.8291733296231));
#47602=CARTESIAN_POINT('Ctrl Pts',(4.90416497508538,-9.53368282748551,-37.8167838493645));
#47603=CARTESIAN_POINT('Ctrl Pts',(3.7481257854858,-9.56405517251088,-37.8091138533209));
#47604=CARTESIAN_POINT('Ctrl Pts',(3.17396066044241,-9.55344044321367,-37.8117941348724));
#47605=CARTESIAN_POINT('Ctrl Pts',(2.6,-9.55344044321367,-37.8117941348724));
#47606=CARTESIAN_POINT('',(2.1,-9.55344044321367,-37.8117941348724));
#47607=CARTESIAN_POINT('Ctrl Pts',(2.1,-9.55344044321367,-37.8117941348724));
#47608=CARTESIAN_POINT('Ctrl Pts',(2.26666666666667,-9.55344044321367,-37.8117941348724));
#47609=CARTESIAN_POINT('Ctrl Pts',(2.43346068603049,-9.55343112836961,-37.8117982691431));
#47610=CARTESIAN_POINT('Ctrl Pts',(2.60034598551963,-9.55341685439516,-37.8118046211416));
#47611=CARTESIAN_POINT('',(2.1,-23.6059783742347,-31.0444485374626));
#47612=CARTESIAN_POINT('Origin',(2.1,0.,0.));
#47613=CARTESIAN_POINT('',(2.6,-23.6059783742347,-31.0444485374626));
#47614=CARTESIAN_POINT('Ctrl Pts',(2.59962088519067,-23.6059943926253,-31.0444314441149));
#47615=CARTESIAN_POINT('Ctrl Pts',(2.43319308967147,-23.6059846984282,-31.0444417950463));
#47616=CARTESIAN_POINT('Ctrl Pts',(2.26666666666667,-23.6059783742347,-31.0444485374626));
#47617=CARTESIAN_POINT('Ctrl Pts',(2.1,-23.6059783742347,-31.0444485374626));
#47618=CARTESIAN_POINT('',(6.,-23.5490023259382,-31.0876903203335));
#47619=CARTESIAN_POINT('Ctrl Pts',(2.6,-23.6059783742347,-31.0444485374626));
#47620=CARTESIAN_POINT('Ctrl Pts',(3.15786519714955,-23.6059783742347,-31.0444485374626));
#47621=CARTESIAN_POINT('Ctrl Pts',(3.71593098901213,-23.6148788600968,-31.0376823457423));
#47622=CARTESIAN_POINT('Ctrl Pts',(4.82421019263741,-23.5909388702326,-31.055882316366));
#47623=CARTESIAN_POINT('Ctrl Pts',(5.40687161376251,-23.5492358231876,-31.0875134455894));
#47624=CARTESIAN_POINT('Ctrl Pts',(6.,-23.5490023259382,-31.0876903203335));
#47625=CARTESIAN_POINT('',(6.,-24.9583551264995,-29.9679914138325));
#47626=CARTESIAN_POINT('Origin',(6.,0.,0.));
#47627=CARTESIAN_POINT('',(2.6,-25.0132750426772,-29.9221668941168));
#47628=CARTESIAN_POINT('Ctrl Pts',(6.,-24.9583551264995,-29.9679914138325));
#47629=CARTESIAN_POINT('Ctrl Pts',(5.46151291267476,-24.9586028954432,-29.9677850634902));
#47630=CARTESIAN_POINT('Ctrl Pts',(4.90416494331291,-24.9976390041765,-29.9352349778897));
#47631=CARTESIAN_POINT('Ctrl Pts',(3.74812575287323,-25.0216756519015,-29.9151464861394));
#47632=CARTESIAN_POINT('Ctrl Pts',(3.17396064416408,-25.0132750426772,-29.9221668941168));
#47633=CARTESIAN_POINT('Ctrl Pts',(2.6,-25.0132750426772,-29.9221668941168));
#47634=CARTESIAN_POINT('',(2.1,-25.0132750426772,-29.9221668941168));
#47635=CARTESIAN_POINT('Ctrl Pts',(2.1,-25.0132750426772,-29.9221668941168));
#47636=CARTESIAN_POINT('Ctrl Pts',(2.26666666666667,-25.0132750426772,-29.9221668941168));
#47637=CARTESIAN_POINT('Ctrl Pts',(2.43357825612586,-25.0132726154855,-29.9221698582808));
#47638=CARTESIAN_POINT('Ctrl Pts',(2.60065266451408,-25.0132684616017,-29.9221747898881));
#47639=CARTESIAN_POINT('',(2.1,-34.7379330218401,-17.7278314909114));
#47640=CARTESIAN_POINT('Origin',(2.1,0.,0.));
#47641=CARTESIAN_POINT('',(2.6,-34.7379330218401,-17.7278314909114));
#47642=CARTESIAN_POINT('Ctrl Pts',(2.59964387481778,-34.7379384978419,-17.727810026438));
#47643=CARTESIAN_POINT('Ctrl Pts',(2.43320198848801,-34.7379351912261,-17.7278230129461));
#47644=CARTESIAN_POINT('Ctrl Pts',(2.26666666666667,-34.7379330218401,-17.7278314909114));
#47645=CARTESIAN_POINT('Ctrl Pts',(2.1,-34.7379330218401,-17.7278314909114));
#47646=CARTESIAN_POINT('',(6.,-34.705361282547,-17.7915119719457));
#47647=CARTESIAN_POINT('Ctrl Pts',(2.6,-34.7379330218401,-17.7278314909114));
#47648=CARTESIAN_POINT('Ctrl Pts',(3.15786555369928,-34.7379330218401,-17.7278314909114));
#47649=CARTESIAN_POINT('Ctrl Pts',(3.71593170347639,-34.7430163549277,-17.7178735613284));
#47650=CARTESIAN_POINT('Ctrl Pts',(4.82421093519821,-34.7293437970088,-17.7446584260543));
#47651=CARTESIAN_POINT('Ctrl Pts',(5.40687201153467,-34.7054949131345,-17.7912513028229));
#47652=CARTESIAN_POINT('Ctrl Pts',(6.,-34.705361282547,-17.7915119719457));
#47653=CARTESIAN_POINT('',(6.,-35.4893251315053,-16.1712028529206));
#47654=CARTESIAN_POINT('Origin',(6.,0.,0.));
#47655=CARTESIAN_POINT('',(2.6,-35.5189237522517,-16.106087528687));
#47656=CARTESIAN_POINT('Ctrl Pts',(6.,-35.4893251315053,-16.1712028529206));
#47657=CARTESIAN_POINT('Ctrl Pts',(5.46151292711359,-35.4894588315483,-16.1709094347785));
#47658=CARTESIAN_POINT('Ctrl Pts',(4.90416497508538,-35.5105061962146,-16.1246456907818));
#47659=CARTESIAN_POINT('Ctrl Pts',(3.7481257854858,-35.5234463992192,-16.0961174709311));
#47660=CARTESIAN_POINT('Ctrl Pts',(3.17396066044241,-35.5189237522517,-16.106087528687));
#47661=CARTESIAN_POINT('Ctrl Pts',(2.6,-35.5189237522517,-16.106087528687));
#47662=CARTESIAN_POINT('',(2.1,-35.5189237522517,-16.106087528687));
#47663=CARTESIAN_POINT('Ctrl Pts',(2.1,-35.5189237522517,-16.106087528687));
#47664=CARTESIAN_POINT('Ctrl Pts',(2.26666666666667,-35.5189237522517,-16.106087528687));
#47665=CARTESIAN_POINT('Ctrl Pts',(2.43346396189077,-35.5189213983861,-16.1060969924349));
#47666=CARTESIAN_POINT('Ctrl Pts',(2.60035429878701,-35.5189178073564,-16.1061114988275));
#47667=CARTESIAN_POINT('',(2.1,-38.98961400168,-0.899999999999995));
#47668=CARTESIAN_POINT('Origin',(2.1,0.,0.));
#47669=CARTESIAN_POINT('',(2.6,-38.98961400168,-0.89999999999999));
#47670=CARTESIAN_POINT('Ctrl Pts',(2.59961881382767,-38.9896107068492,-0.899977798557519));
#47671=CARTESIAN_POINT('Ctrl Pts',(2.43319228396236,-38.9896127056027,-0.899991237216741));
#47672=CARTESIAN_POINT('Ctrl Pts',(2.26666666666667,-38.98961400168,-0.899999999999995));
#47673=CARTESIAN_POINT('Ctrl Pts',(2.1,-38.98961400168,-0.899999999999995));
#47674=CARTESIAN_POINT('',(6.,-38.9878978038234,-0.971506478939042));
#47675=CARTESIAN_POINT('Ctrl Pts',(2.6,-38.98961400168,-0.899999999999995));
#47676=CARTESIAN_POINT('Ctrl Pts',(3.15786519714955,-38.98961400168,-0.899999999999995));
#47677=CARTESIAN_POINT('Ctrl Pts',(3.71593098901213,-38.9898733421432,-0.888822668408729));
#47678=CARTESIAN_POINT('Ctrl Pts',(4.82421019263741,-38.9891763126199,-0.918887202252576));
#47679=CARTESIAN_POINT('Ctrl Pts',(5.40687161376251,-38.9879051007338,-0.971213643839228));
#47680=CARTESIAN_POINT('Ctrl Pts',(6.,-38.9878978038234,-0.971506478939041));
#47681=CARTESIAN_POINT('',(6.,-39.,-4.77612251667468E-15));
#47682=CARTESIAN_POINT('Origin',(6.,0.,0.));
#47683=CARTESIAN_POINT('',(0.499999999999998,-39.,-4.77612251667468E-15));
#47684=CARTESIAN_POINT('',(1.55,-39.,-4.77612251667468E-15));
#47685=CARTESIAN_POINT('Origin',(0.499999999999998,0.,0.));
#47686=CARTESIAN_POINT('',(6.,-38.9911990462069,0.828490759799985));
#47687=CARTESIAN_POINT('Origin',(6.,0.,0.));
#47688=CARTESIAN_POINT('',(2.6,-38.98961400168,0.90000000000001));
#47689=CARTESIAN_POINT('Ctrl Pts',(6.,-38.9911990462069,0.828490759799983));
#47690=CARTESIAN_POINT('Ctrl Pts',(5.46151291267476,-38.9911921964225,0.82881313069457));
#47691=CARTESIAN_POINT('Ctrl Pts',(4.90416494331291,-38.9900821304425,0.879627435876937));
#47692=CARTESIAN_POINT('Ctrl Pts',(3.74812575287323,-38.9893629198842,0.910945013542259));
#47693=CARTESIAN_POINT('Ctrl Pts',(3.17396064416408,-38.98961400168,0.900000000000005));
#47694=CARTESIAN_POINT('Ctrl Pts',(2.6,-38.98961400168,0.900000000000005));
#47695=CARTESIAN_POINT('',(2.1,-38.98961400168,0.900000000000005));
#47696=CARTESIAN_POINT('Ctrl Pts',(2.1,-38.98961400168,0.900000000000005));
#47697=CARTESIAN_POINT('Ctrl Pts',(2.26666666666667,-38.98961400168,0.900000000000005));
#47698=CARTESIAN_POINT('Ctrl Pts',(2.43357901978584,-38.9896147918638,0.899996432344951));
#47699=CARTESIAN_POINT('Ctrl Pts',(2.60065465957353,-38.9896160358867,0.899990387940704));
#47700=CARTESIAN_POINT('',(2.1,-35.5189237522517,16.106087528687));
#47701=CARTESIAN_POINT('Origin',(2.1,0.,0.));
#47702=CARTESIAN_POINT('',(2.6,-35.5189237522517,16.106087528687));
#47703=CARTESIAN_POINT('Ctrl Pts',(2.59964104784901,-35.5189096730421,16.1061056668086));
#47704=CARTESIAN_POINT('Ctrl Pts',(2.43320088693784,-35.5189181968381,16.1060946966857));
#47705=CARTESIAN_POINT('Ctrl Pts',(2.26666666666667,-35.5189237522517,16.106087528687));
#47706=CARTESIAN_POINT('Ctrl Pts',(2.1,-35.5189237522517,16.106087528687));
#47707=CARTESIAN_POINT('',(6.,-35.548403009865,16.0409177869666));
#47708=CARTESIAN_POINT('Ctrl Pts',(2.6,-35.5189237522517,16.106087528687));
#47709=CARTESIAN_POINT('Ctrl Pts',(3.15786555369928,-35.5189237522517,16.106087528687));
#47710=CARTESIAN_POINT('Ctrl Pts',(3.71593170347639,-35.5143077357431,16.1162705060734));
#47711=CARTESIAN_POINT('Ctrl Pts',(4.82421093519821,-35.5267242858117,16.0888807798457));
#47712=CARTESIAN_POINT('Ctrl Pts',(5.40687201153467,-35.5482825278469,16.0411847881066));
#47713=CARTESIAN_POINT('Ctrl Pts',(6.,-35.548403009865,16.0409177869666));
#47714=CARTESIAN_POINT('',(6.,-34.7703877941326,17.6640916167698));
#47715=CARTESIAN_POINT('Origin',(6.,0.,0.));
#47716=CARTESIAN_POINT('',(2.6,-34.7379330218401,17.7278314909114));
#47717=CARTESIAN_POINT('Ctrl Pts',(6.,-34.7703877941326,17.6640916167698));
#47718=CARTESIAN_POINT('Ctrl Pts',(5.46151292711359,-34.7702417512048,17.664379090892));
#47719=CARTESIAN_POINT('Ctrl Pts',(4.90416497508538,-34.7471941168769,17.7096795557888));
#47720=CARTESIAN_POINT('Ctrl Pts',(3.7481257854858,-34.7329579410662,17.7375836680294));
#47721=CARTESIAN_POINT('Ctrl Pts',(3.17396066044241,-34.7379330218401,17.7278314909114));
#47722=CARTESIAN_POINT('Ctrl Pts',(2.6,-34.7379330218401,17.7278314909114));
#47723=CARTESIAN_POINT('',(2.10000000000001,-34.7379330218401,17.7278314909114));
#47724=CARTESIAN_POINT('Ctrl Pts',(2.10000000000001,-34.7379330218401,17.7278314909114));
#47725=CARTESIAN_POINT('Ctrl Pts',(2.26666666666667,-34.7379330218401,17.7278314909114));
#47726=CARTESIAN_POINT('Ctrl Pts',(2.4334616795417,-34.7379389230122,17.7278236408502));
#47727=CARTESIAN_POINT('Ctrl Pts',(2.6003485284748,-34.7379479808194,17.7278116174341));
#47728=CARTESIAN_POINT('',(2.10000000000001,-25.0132750426772,29.9221668941169));
#47729=CARTESIAN_POINT('Origin',(2.10000000000001,0.,0.));
#47730=CARTESIAN_POINT('',(2.6,-25.0132750426772,29.9221668941169));
#47731=CARTESIAN_POINT('Ctrl Pts',(2.59962040969903,-25.0132550013658,29.9221785815268));
#47732=CARTESIAN_POINT('Ctrl Pts',(2.43319290469077,-25.0132671359778,29.9221715099518));
#47733=CARTESIAN_POINT('Ctrl Pts',(2.26666666666667,-25.0132750426772,29.9221668941169));
#47734=CARTESIAN_POINT('Ctrl Pts',(2.10000000000001,-25.0132750426772,29.9221668941169));
#47735=CARTESIAN_POINT('',(6.,-25.0681110272506,29.8762415562171));
#47736=CARTESIAN_POINT('Ctrl Pts',(2.6,-25.0132750426772,29.9221668941169));
#47737=CARTESIAN_POINT('Ctrl Pts',(3.15786519714955,-25.0132750426772,29.9221668941169));
#47738=CARTESIAN_POINT('Ctrl Pts',(3.71593098901213,-25.0046979490832,29.9293386069149));
#47739=CARTESIAN_POINT('Ctrl Pts',(4.82421019263741,-25.0277687573486,29.91004871704));
#47740=CARTESIAN_POINT('Ctrl Pts',(5.40687161376251,-25.0678866290996,29.8764298408698));
#47741=CARTESIAN_POINT('Ctrl Pts',(6.,-25.0681110272506,29.8762415562171));
#47742=CARTESIAN_POINT('',(6.,-23.6628748086085,31.0011024931715));
#47743=CARTESIAN_POINT('Origin',(6.,0.,0.));
#47744=CARTESIAN_POINT('',(2.6,-23.6059783742347,31.0444485374626));
#47745=CARTESIAN_POINT('Ctrl Pts',(6.,-23.6628748086085,31.0011024931715));
#47746=CARTESIAN_POINT('Ctrl Pts',(5.46151291267476,-23.6626184981234,31.0012981327595));
#47747=CARTESIAN_POINT('Ctrl Pts',(4.90416494331291,-23.6221981597541,31.0321124492985));
#47748=CARTESIAN_POINT('Ctrl Pts',(3.74812575287323,-23.5972646711323,31.0510763381348));
#47749=CARTESIAN_POINT('Ctrl Pts',(3.17396064416408,-23.6059783742347,31.0444485374626));
#47750=CARTESIAN_POINT('Ctrl Pts',(2.6,-23.6059783742347,31.0444485374626));
#47751=CARTESIAN_POINT('',(2.1,-23.6059783742347,31.0444485374626));
#47752=CARTESIAN_POINT('Ctrl Pts',(2.1,-23.6059783742347,31.0444485374626));
#47753=CARTESIAN_POINT('Ctrl Pts',(2.26666666666667,-23.6059783742347,31.0444485374626));
#47754=CARTESIAN_POINT('Ctrl Pts',(2.43357841627175,-23.6059817731134,31.0444468517412));
#47755=CARTESIAN_POINT('Ctrl Pts',(2.60065308282599,-23.6059874569122,31.0444439322163));
#47756=CARTESIAN_POINT('',(2.1,-9.55344044321367,37.8117941348724));
#47757=CARTESIAN_POINT('Origin',(2.1,0.,0.));
#47758=CARTESIAN_POINT('',(2.6,-9.55344044321366,37.8117941348724));
#47759=CARTESIAN_POINT('Ctrl Pts',(2.59964755923549,-9.55341505766335,37.8117946735604));
#47760=CARTESIAN_POINT('Ctrl Pts',(2.43320343087526,-9.5534304198444,37.8117943540172));
#47761=CARTESIAN_POINT('Ctrl Pts',(2.26666666666667,-9.55344044321366,37.8117941348724));
#47762=CARTESIAN_POINT('Ctrl Pts',(2.1,-9.55344044321366,37.8117941348724));
#47763=CARTESIAN_POINT('',(6.,-9.62277221548329,37.7942092772018));
#47764=CARTESIAN_POINT('Ctrl Pts',(2.6,-9.55344044321366,37.8117941348724));
#47765=CARTESIAN_POINT('Ctrl Pts',(3.15786555369928,-9.55344044321366,37.8117941348724));
#47766=CARTESIAN_POINT('Ctrl Pts',(3.71593170347639,-9.54260103168937,37.8145341703953));
#47767=CARTESIAN_POINT('Ctrl Pts',(4.82421093519821,-9.57175677429238,37.8071646051639));
#47768=CARTESIAN_POINT('Ctrl Pts',(5.40687201153467,-9.6224883462765,37.7942815530548));
#47769=CARTESIAN_POINT('Ctrl Pts',(6.,-9.62277221548328,37.7942092772018));
#47770=CARTESIAN_POINT('',(6.,-7.86863926112478,38.1979648172293));
#47771=CARTESIAN_POINT('Origin',(6.,0.,0.));
#47772=CARTESIAN_POINT('',(2.6,-7.79857020128639,38.2123318159937));
#47773=CARTESIAN_POINT('Ctrl Pts',(6.,-7.86863926112479,38.1979648172293));
#47774=CARTESIAN_POINT('Ctrl Pts',(5.46151292711359,-7.86832344852962,38.1980298734541));
#47775=CARTESIAN_POINT('Ctrl Pts',(4.90416497508538,-7.81853615394239,38.2082548852227));
#47776=CARTESIAN_POINT('Ctrl Pts',(3.7481257854858,-7.78784373006694,38.2145225241958));
#47777=CARTESIAN_POINT('Ctrl Pts',(3.17396066044241,-7.79857020128638,38.2123318159937));
#47778=CARTESIAN_POINT('Ctrl Pts',(2.6,-7.79857020128638,38.2123318159937));
#47779=CARTESIAN_POINT('',(2.1,-7.79857020128638,38.2123318159937));
#47780=CARTESIAN_POINT('Ctrl Pts',(2.1,-7.79857020128638,38.2123318159937));
#47781=CARTESIAN_POINT('Ctrl Pts',(2.26666666666667,-7.79857020128638,38.2123318159937));
#47782=CARTESIAN_POINT('Ctrl Pts',(2.43346449336972,-7.79857975198003,38.2123316464336));
#47783=CARTESIAN_POINT('Ctrl Pts',(2.60035565904183,-7.79859438653547,38.2123314033356));
#47784=CARTESIAN_POINT('',(2.1,7.79857020128639,38.2123318159937));
#47785=CARTESIAN_POINT('Origin',(2.1,0.,0.));
#47786=CARTESIAN_POINT('',(2.6,7.79857020128639,38.2123318159937));
#47787=CARTESIAN_POINT('Ctrl Pts',(2.59962016861433,7.79859172526737,38.2123234687558));
#47788=CARTESIAN_POINT('Ctrl Pts',(2.4331928109074,7.79857869688915,38.2123285258734));
#47789=CARTESIAN_POINT('Ctrl Pts',(2.26666666666667,7.79857020128638,38.2123318159937));
#47790=CARTESIAN_POINT('Ctrl Pts',(2.1,7.79857020128638,38.2123318159937));
#47791=CARTESIAN_POINT('',(6.,7.72847464911697,38.226570335278));
#47792=CARTESIAN_POINT('Ctrl Pts',(2.6,7.79857020128639,38.2123318159937));
#47793=CARTESIAN_POINT('Ctrl Pts',(3.15786519714955,7.79857020128639,38.2123318159937));
#47794=CARTESIAN_POINT('Ctrl Pts',(3.71593098901213,7.80952500252052,38.2100974639853));
#47795=CARTESIAN_POINT('Ctrl Pts',(4.82421019263741,7.78005914564888,38.2161078985973));
#47796=CARTESIAN_POINT('Ctrl Pts',(5.4068716137625,7.72876176594476,38.2265122872997));
#47797=CARTESIAN_POINT('Ctrl Pts',(6.,7.72847464911697,38.226570335278));
#47798=CARTESIAN_POINT('',(6.,9.48407679455224,37.8292517419395));
#47799=CARTESIAN_POINT('Origin',(6.,0.,0.));
#47800=CARTESIAN_POINT('',(2.6,9.55344044321367,37.8117941348724));
#47801=CARTESIAN_POINT('Ctrl Pts',(6.,9.48407679455224,37.8292517419395));
#47802=CARTESIAN_POINT('Ctrl Pts',(5.46151291267476,9.48438955871503,37.829173329621));
#47803=CARTESIAN_POINT('Ctrl Pts',(4.90416494331291,9.53368283025682,37.8167838486652));
#47804=CARTESIAN_POINT('Ctrl Pts',(3.74812575287323,9.56405517145952,37.8091138535859));
#47805=CARTESIAN_POINT('Ctrl Pts',(3.17396064416408,9.55344044321367,37.8117941348724));
#47806=CARTESIAN_POINT('Ctrl Pts',(2.6,9.55344044321367,37.8117941348724));
#47807=CARTESIAN_POINT('',(2.1,9.55344044321367,37.8117941348724));
#47808=CARTESIAN_POINT('Ctrl Pts',(2.1,9.55344044321367,37.8117941348724));
#47809=CARTESIAN_POINT('Ctrl Pts',(2.26666666666667,9.55344044321367,37.8117941348724));
#47810=CARTESIAN_POINT('Ctrl Pts',(2.43357853708729,9.55343703309769,37.8117957327629));
#47811=CARTESIAN_POINT('Ctrl Pts',(2.60065339842836,9.55343124887636,37.8117983430894));
#47812=CARTESIAN_POINT('',(2.1,23.6059783742347,31.0444485374626));
#47813=CARTESIAN_POINT('Origin',(2.1,0.,0.));
#47814=CARTESIAN_POINT('',(2.6,23.6059783742347,31.0444485374626));
#47815=CARTESIAN_POINT('Ctrl Pts',(2.59963809215921,23.6059921558338,31.0444315655759));
#47816=CARTESIAN_POINT('Ctrl Pts',(2.43319973276619,23.6059838236274,31.0444418375603));
#47817=CARTESIAN_POINT('Ctrl Pts',(2.26666666666667,23.6059783742347,31.0444485374626));
#47818=CARTESIAN_POINT('Ctrl Pts',(2.1,23.6059783742347,31.0444485374626));
#47819=CARTESIAN_POINT('',(6.,23.5490023259382,31.0876903203335));
#47820=CARTESIAN_POINT('Ctrl Pts',(2.6,23.6059783742347,31.0444485374626));
#47821=CARTESIAN_POINT('Ctrl Pts',(3.15786555369928,23.6059783742347,31.0444485374626));
#47822=CARTESIAN_POINT('Ctrl Pts',(3.71593170347639,23.6148788828132,31.0376823284867));
#47823=CARTESIAN_POINT('Ctrl Pts',(4.82421093519821,23.5909388165246,31.0558823571826));
#47824=CARTESIAN_POINT('Ctrl Pts',(5.40687201153467,23.549235823031,31.087513445708));
#47825=CARTESIAN_POINT('Ctrl Pts',(6.,23.5490023259382,31.0876903203335));
#47826=CARTESIAN_POINT('',(6.,24.9583551264995,29.9679914138325));
#47827=CARTESIAN_POINT('Origin',(6.,0.,0.));
#47828=CARTESIAN_POINT('',(2.6,25.0132750426772,29.9221668941169));
#47829=CARTESIAN_POINT('Ctrl Pts',(6.,24.9583551264995,29.9679914138325));
#47830=CARTESIAN_POINT('Ctrl Pts',(5.46151292711359,24.9586028954365,29.9677850634957));
#47831=CARTESIAN_POINT('Ctrl Pts',(4.90416497508538,24.9976390019831,29.9352349797221));
#47832=CARTESIAN_POINT('Ctrl Pts',(3.7481257854858,25.0216756527337,29.9151464854446));
#47833=CARTESIAN_POINT('Ctrl Pts',(3.17396066044241,25.0132750426772,29.9221668941169));
#47834=CARTESIAN_POINT('Ctrl Pts',(2.6,25.0132750426772,29.9221668941169));
#47835=CARTESIAN_POINT('',(2.1,25.0132750426772,29.9221668941169));
#47836=CARTESIAN_POINT('Ctrl Pts',(2.1,25.0132750426772,29.9221668941169));
#47837=CARTESIAN_POINT('Ctrl Pts',(2.26666666666667,25.0132750426772,29.9221668941169));
#47838=CARTESIAN_POINT('Ctrl Pts',(2.43357395784791,25.0132711380509,29.9221719829006));
#47839=CARTESIAN_POINT('Ctrl Pts',(2.60064121585505,25.0132646768699,29.9221802322046));
#47840=CARTESIAN_POINT('',(2.1,34.7379330218401,17.7278314909114));
#47841=CARTESIAN_POINT('Origin',(2.1,0.,0.));
#47842=CARTESIAN_POINT('',(2.6,34.7379330218401,17.7278314909114));
#47843=CARTESIAN_POINT('Ctrl Pts',(2.59961936767386,34.7379397798986,17.7278098133928));
#47844=CARTESIAN_POINT('Ctrl Pts',(2.43319249936566,34.7379356930243,17.7278229371174));
#47845=CARTESIAN_POINT('Ctrl Pts',(2.26666666666667,34.7379330218401,17.7278314909114));
#47846=CARTESIAN_POINT('Ctrl Pts',(2.1,34.7379330218401,17.7278314909114));
#47847=CARTESIAN_POINT('',(6.,34.705361282547,17.7915119719457));
#47848=CARTESIAN_POINT('Ctrl Pts',(2.6,34.7379330218401,17.7278314909114));
#47849=CARTESIAN_POINT('Ctrl Pts',(3.15786519714955,34.7379330218401,17.7278314909114));
#47850=CARTESIAN_POINT('Ctrl Pts',(3.71593098901213,34.7430163419479,17.7178735867313));
#47851=CARTESIAN_POINT('Ctrl Pts',(4.82421019263741,34.7293438276883,17.7446583659768));
#47852=CARTESIAN_POINT('Ctrl Pts',(5.40687161376251,34.7054949132241,17.7912513026481));
#47853=CARTESIAN_POINT('Ctrl Pts',(6.,34.705361282547,17.7915119719457));
#47854=CARTESIAN_POINT('',(6.,35.4893251315053,16.1712028529206));
#47855=CARTESIAN_POINT('Origin',(6.,0.,0.));
#47856=CARTESIAN_POINT('',(2.6,35.5189237522517,16.106087528687));
#47857=CARTESIAN_POINT('Ctrl Pts',(6.,35.4893251315053,16.1712028529206));
#47858=CARTESIAN_POINT('Ctrl Pts',(5.46151291267476,35.4894588315519,16.1709094347706));
#47859=CARTESIAN_POINT('Ctrl Pts',(4.90416494331291,35.5105061973958,16.1246456881791));
#47860=CARTESIAN_POINT('Ctrl Pts',(3.74812575287323,35.5234463987708,16.0961174719183));
#47861=CARTESIAN_POINT('Ctrl Pts',(3.17396064416408,35.5189237522517,16.106087528687));
#47862=CARTESIAN_POINT('Ctrl Pts',(2.6,35.5189237522517,16.106087528687));
#47863=CARTESIAN_POINT('',(2.1,35.5189237522517,16.106087528687));
#47864=CARTESIAN_POINT('Ctrl Pts',(2.1,35.5189237522517,16.106087528687));
#47865=CARTESIAN_POINT('Ctrl Pts',(2.26666666666667,35.5189237522517,16.106087528687));
#47866=CARTESIAN_POINT('Ctrl Pts',(2.43357876746602,35.5189228948792,16.1060911408517));
#47867=CARTESIAN_POINT('Ctrl Pts',(2.60065400029651,35.5189213597892,16.1060972122346));
#47868=CARTESIAN_POINT('',(2.1,38.98961400168,0.9));
#47869=CARTESIAN_POINT('Origin',(2.1,0.,0.));
#47870=CARTESIAN_POINT('',(2.6,38.98961400168,0.899999999999996));
#47871=CARTESIAN_POINT('Ctrl Pts',(2.59964719237566,38.9896088955429,0.899975267580465));
#47872=CARTESIAN_POINT('Ctrl Pts',(2.43320328750148,38.9896119918161,0.899990232939572));
#47873=CARTESIAN_POINT('Ctrl Pts',(2.26666666666667,38.98961400168,0.9));
#47874=CARTESIAN_POINT('Ctrl Pts',(2.1,38.98961400168,0.9));
#47875=CARTESIAN_POINT('',(6.,38.9878978038234,0.971506478939047));
#47876=CARTESIAN_POINT('Ctrl Pts',(2.6,38.98961400168,0.9));
#47877=CARTESIAN_POINT('Ctrl Pts',(3.15786555369928,38.98961400168,0.9));
#47878=CARTESIAN_POINT('Ctrl Pts',(3.71593170347639,38.9898733428157,0.888822639889713));
#47879=CARTESIAN_POINT('Ctrl Pts',(4.82421093519821,38.9891763110452,0.918887269691915));
#47880=CARTESIAN_POINT('Ctrl Pts',(5.40687201153467,38.9879051007289,0.971213644035619));
#47881=CARTESIAN_POINT('Ctrl Pts',(6.,38.9878978038234,0.971506478939046));
#47882=CARTESIAN_POINT('',(6.,38.9911990462069,-0.82849075979999));
#47883=CARTESIAN_POINT('Origin',(6.,0.,0.));
#47884=CARTESIAN_POINT('Ctrl Pts',(6.,38.9911990462069,-0.828490759799977));
#47885=CARTESIAN_POINT('Ctrl Pts',(5.46151292711359,38.9911921964227,-0.828813130685921));
#47886=CARTESIAN_POINT('Ctrl Pts',(4.90416497508538,38.9900821305076,-0.879627433019496));
#47887=CARTESIAN_POINT('Ctrl Pts',(3.7481257854858,38.9893629198599,-0.910945014626199));
#47888=CARTESIAN_POINT('Ctrl Pts',(3.17396066044241,38.98961400168,-0.9));
#47889=CARTESIAN_POINT('Ctrl Pts',(2.6,38.98961400168,-0.9));
#47890=CARTESIAN_POINT('Origin',(2.44847982464479,0.,-1.17996027893162E-15));
#47891=CARTESIAN_POINT('',(2.79695964929223,34.3237608806509,17.5283766998975));
#47892=CARTESIAN_POINT('Ctrl Pts',(2.09999999999999,34.7379330218402,17.7278314909114));
#47893=CARTESIAN_POINT('Ctrl Pts',(2.33231184706804,34.599880855471,17.6613490715166));
#47894=CARTESIAN_POINT('Ctrl Pts',(2.56464811501599,34.4618137435185,17.5948594547083));
#47895=CARTESIAN_POINT('Ctrl Pts',(2.79695964929243,34.323760880652,17.528376699898));
#47896=CARTESIAN_POINT('',(2.79695964929243,24.7266590280231,29.5627617796016));
#47897=CARTESIAN_POINT('Ctrl Pts',(2.79695964929244,24.726659028024,29.5627617796028));
#47898=CARTESIAN_POINT('Ctrl Pts',(2.56464811249614,24.8221945743839,29.6825595655751));
#47899=CARTESIAN_POINT('Ctrl Pts',(2.3323118418722,24.9177399814814,29.8023697165212));
#47900=CARTESIAN_POINT('Ctrl Pts',(2.09999999999999,25.0132750426772,29.9221668941169));
#47901=CARTESIAN_POINT('Origin',(2.79695964928958,0.,-2.35992055786324E-15));
#47902=CARTESIAN_POINT('Origin',(2.44847982464479,0.,-1.17996027893162E-15));
#47903=CARTESIAN_POINT('',(2.79695964929224,7.69627812998458,37.7641609687218));
#47904=CARTESIAN_POINT('Ctrl Pts',(2.1,7.7985702012864,38.2123318159938));
#47905=CARTESIAN_POINT('Ctrl Pts',(2.3323118422578,7.7644741326502,38.0629471787011));
#47906=CARTESIAN_POINT('Ctrl Pts',(2.56464811269316,7.73037437168869,37.9135463642742));
#47907=CARTESIAN_POINT('Ctrl Pts',(2.79695964929243,7.69627812998494,37.764160968723));
#47908=CARTESIAN_POINT('',(2.79695964929243,-7.69627812998452,37.7641609687216));
#47909=CARTESIAN_POINT('Ctrl Pts',(2.79695964929243,-7.69627812998494,37.764160968723));
#47910=CARTESIAN_POINT('Ctrl Pts',(2.56464811432525,-7.73037437144915,37.9135463632247));
#47911=CARTESIAN_POINT('Ctrl Pts',(2.33231184565996,-7.76447413215086,38.0629471765134));
#47912=CARTESIAN_POINT('Ctrl Pts',(2.1,-7.7985702012864,38.2123318159938));
#47913=CARTESIAN_POINT('Origin',(2.79695964928958,0.,-2.35992055786324E-15));
#47914=CARTESIAN_POINT('Origin',(2.4484798246448,0.,-1.17996027893162E-15));
#47915=CARTESIAN_POINT('',(2.79695964929224,-24.7266590280233,29.5627617796018));
#47916=CARTESIAN_POINT('Ctrl Pts',(2.10000000000001,-25.0132750426772,29.9221668941169));
#47917=CARTESIAN_POINT('Ctrl Pts',(2.33231184323714,-24.9177399809201,29.8023697158173));
#47918=CARTESIAN_POINT('Ctrl Pts',(2.5646481131599,-24.8221945741109,29.6825595652328));
#47919=CARTESIAN_POINT('Ctrl Pts',(2.79695964929245,-24.726659028024,29.5627617796028));
#47920=CARTESIAN_POINT('',(2.79695964929243,-34.3237608806506,17.5283766998975));
#47921=CARTESIAN_POINT('Ctrl Pts',(2.79695964929245,-34.323760880652,17.528376699898));
#47922=CARTESIAN_POINT('Ctrl Pts',(2.56464811314235,-34.4618137446319,17.5948594552445));
#47923=CARTESIAN_POINT('Ctrl Pts',(2.33231184320826,-34.5998808577647,17.6613490726212));
#47924=CARTESIAN_POINT('Ctrl Pts',(2.09999999999999,-34.7379330218402,17.7278314909114));
#47925=CARTESIAN_POINT('Origin',(2.79695964928959,0.,-2.35992055786324E-15));
#47926=CARTESIAN_POINT('Origin',(2.44847982464479,0.,-1.17996027893162E-15));
#47927=CARTESIAN_POINT('',(2.79695964929223,-38.529917606006,-0.900000000000067));
#47928=CARTESIAN_POINT('Ctrl Pts',(2.1,-38.98961400168,-0.899999999999995));
#47929=CARTESIAN_POINT('Ctrl Pts',(2.33231184677866,-38.8363876571131,-0.899999999999995));
#47930=CARTESIAN_POINT('Ctrl Pts',(2.56464811488244,-38.6831447239067,-0.899999999999995));
#47931=CARTESIAN_POINT('Ctrl Pts',(2.79695964929244,-38.5299176060072,-0.899999999999995));
#47932=CARTESIAN_POINT('',(2.79695964929243,-35.1047516110623,-15.906632737673));
#47933=CARTESIAN_POINT('Ctrl Pts',(2.79695964929244,-35.1047516110636,-15.9066327376736));
#47934=CARTESIAN_POINT('Ctrl Pts',(2.56464811161146,-35.2428044759532,-15.9731154934582));
#47935=CARTESIAN_POINT('Ctrl Pts',(2.33231184003613,-35.3808715900613,-16.0396051113046));
#47936=CARTESIAN_POINT('Ctrl Pts',(2.09999999999999,-35.5189237522517,-16.106087528687));
#47937=CARTESIAN_POINT('Origin',(2.79695964928958,0.,-2.35992055786324E-15));
#47938=CARTESIAN_POINT('Origin',(2.44847982464479,0.,-1.17996027893162E-15));
#47939=CARTESIAN_POINT('',(2.79695964929223,-23.3193623595807,-30.6850434229476));
#47940=CARTESIAN_POINT('Ctrl Pts',(2.1,-23.6059783742347,-31.0444485374625));
#47941=CARTESIAN_POINT('Ctrl Pts',(2.3323118390093,-23.5104433142162,-30.9246513613431));
#47942=CARTESIAN_POINT('Ctrl Pts',(2.56464811110358,-23.4148979065141,-30.8048412096388));
#47943=CARTESIAN_POINT('Ctrl Pts',(2.79695964929244,-23.3193623595815,-30.6850434229485));
#47944=CARTESIAN_POINT('',(2.79695964929243,-9.45114837191197,-37.3636232876002));
#47945=CARTESIAN_POINT('Ctrl Pts',(2.79695964929244,-9.45114837191219,-37.3636232876015));
#47946=CARTESIAN_POINT('Ctrl Pts',(2.56464811107789,-9.48524461385302,-37.5130086841914));
#47947=CARTESIAN_POINT('Ctrl Pts',(2.33231183894366,-9.51934437506386,-37.6624094997107));
#47948=CARTESIAN_POINT('Ctrl Pts',(2.09999999999998,-9.55344044321365,-37.8117941348723));
#47949=CARTESIAN_POINT('Origin',(2.79695964928958,0.,-2.35992055786324E-15));
#47950=CARTESIAN_POINT('Origin',(2.44847982464479,0.,-1.17996027893162E-15));
#47951=CARTESIAN_POINT('',(2.79695964929223,9.451148371912,-37.3636232876004));
#47952=CARTESIAN_POINT('Ctrl Pts',(2.09999999999999,9.55344044321364,-37.8117941348723));
#47953=CARTESIAN_POINT('Ctrl Pts',(2.33231183759833,9.5193443752613,-37.6624095005758));
#47954=CARTESIAN_POINT('Ctrl Pts',(2.56464811043332,9.48524461394761,-37.5130086846059));
#47955=CARTESIAN_POINT('Ctrl Pts',(2.79695964929243,9.45114837191218,-37.3636232876015));
#47956=CARTESIAN_POINT('',(2.79695964929243,23.3193623595806,-30.6850434229474));
#47957=CARTESIAN_POINT('Ctrl Pts',(2.79695964929244,23.3193623595815,-30.6850434229485));
#47958=CARTESIAN_POINT('Ctrl Pts',(2.56464811252804,23.4148979059282,-30.8048412089043));
#47959=CARTESIAN_POINT('Ctrl Pts',(2.33231184190073,23.5104433130272,-30.9246513598521));
#47960=CARTESIAN_POINT('Ctrl Pts',(2.09999999999999,23.6059783742347,-31.0444485374625));
#47961=CARTESIAN_POINT('Origin',(2.79695964928958,0.,-2.35992055786324E-15));
#47962=CARTESIAN_POINT('Origin',(2.44847982464479,0.,-1.17996027893162E-15));
#47963=CARTESIAN_POINT('',(2.79695964929222,38.529917606006,0.900000000000072));
#47964=CARTESIAN_POINT('Ctrl Pts',(2.09999999999999,38.98961400168,0.9));
#47965=CARTESIAN_POINT('Ctrl Pts',(2.33231184201649,38.8363876602541,0.9));
#47966=CARTESIAN_POINT('Ctrl Pts',(2.56464811257203,38.6831447254306,0.9));
#47967=CARTESIAN_POINT('Ctrl Pts',(2.79695964929222,38.5299176060073,0.9));
#47968=CARTESIAN_POINT('',(2.79695964929053,35.1047516110643,15.906632737674));
#47969=CARTESIAN_POINT('Ctrl Pts',(2.79695964929223,35.1047516110637,15.9066327376737));
#47970=CARTESIAN_POINT('Ctrl Pts',(2.56464811186606,35.242804475802,15.9731154933853));
#47971=CARTESIAN_POINT('Ctrl Pts',(2.33231184056647,35.3808715897462,16.0396051111529));
#47972=CARTESIAN_POINT('Ctrl Pts',(2.09999999999999,35.5189237522518,16.1060875286871));
#47973=CARTESIAN_POINT('Origin',(2.79695964928958,0.,-2.35992055786324E-15));
#47974=CARTESIAN_POINT('Origin',(2.44847982464479,0.,-1.17996027893162E-15));
#47975=CARTESIAN_POINT('',(2.79695964929222,23.3193623595807,30.6850434229476));
#47976=CARTESIAN_POINT('Ctrl Pts',(2.09999999999999,23.6059783742348,31.0444485374626));
#47977=CARTESIAN_POINT('Ctrl Pts',(2.3323118440126,23.5104433121588,30.9246513587632));
#47978=CARTESIAN_POINT('Ctrl Pts',(2.56464811353468,23.4148979055144,30.8048412083852));
#47979=CARTESIAN_POINT('Ctrl Pts',(2.79695964929222,23.3193623595817,30.6850434229487));
#47980=CARTESIAN_POINT('',(2.79695964929053,9.4511483719124,37.3636232876023));
#47981=CARTESIAN_POINT('Ctrl Pts',(2.79695964929223,9.45114837191225,37.3636232876018));
#47982=CARTESIAN_POINT('Ctrl Pts',(2.5646481138253,9.48524461344982,37.5130086824249));
#47983=CARTESIAN_POINT('Ctrl Pts',(2.33231184461174,9.519344374232,37.6624094960661));
#47984=CARTESIAN_POINT('Ctrl Pts',(2.09999999999999,9.55344044321369,37.8117941348725));
#47985=CARTESIAN_POINT('Origin',(2.79695964928958,0.,-2.35992055786324E-15));
#47986=CARTESIAN_POINT('Origin',(2.44847982464479,0.,-1.17996027893162E-15));
#47987=CARTESIAN_POINT('',(2.79695964929222,-9.451148371912,37.3636232876004));
#47988=CARTESIAN_POINT('Ctrl Pts',(2.1,-9.55344044321368,37.8117941348725));
#47989=CARTESIAN_POINT('Ctrl Pts',(2.33231184276064,-9.51934437450368,37.6624094972564));
#47990=CARTESIAN_POINT('Ctrl Pts',(2.56464811294314,-9.48524461357928,37.5130086829921));
#47991=CARTESIAN_POINT('Ctrl Pts',(2.79695964929223,-9.45114837191225,37.3636232876018));
#47992=CARTESIAN_POINT('',(2.79695964929053,-23.319362359582,30.6850434229491));
#47993=CARTESIAN_POINT('Ctrl Pts',(2.79695964929223,-23.3193623595817,30.6850434229487));
#47994=CARTESIAN_POINT('Ctrl Pts',(2.56464811276728,-23.41489790583,30.804841208781));
#47995=CARTESIAN_POINT('Ctrl Pts',(2.33231184241615,-23.5104433128153,30.9246513595864));
#47996=CARTESIAN_POINT('Ctrl Pts',(2.09999999999999,-23.6059783742348,31.0444485374626));
#47997=CARTESIAN_POINT('Origin',(2.79695964928958,0.,-2.35992055786324E-15));
#47998=CARTESIAN_POINT('Origin',(2.44847982464479,0.,-1.17996027893162E-15));
#47999=CARTESIAN_POINT('',(2.79695964929221,-35.1047516110625,15.9066327376731));
#48000=CARTESIAN_POINT('Ctrl Pts',(2.1,-35.5189237522518,16.1060875286871));
#48001=CARTESIAN_POINT('Ctrl Pts',(2.33231184336733,-35.3808715880817,16.0396051103513));
#48002=CARTESIAN_POINT('Ctrl Pts',(2.56464811322855,-35.2428044749923,15.9731154929954));
#48003=CARTESIAN_POINT('Ctrl Pts',(2.79695964929223,-35.1047516110637,15.9066327376737));
#48004=CARTESIAN_POINT('',(2.79695964929053,-38.529917606008,0.900000000000031));
#48005=CARTESIAN_POINT('Ctrl Pts',(2.79695964929223,-38.5299176060073,0.900000000000005));
#48006=CARTESIAN_POINT('Ctrl Pts',(2.56464811248588,-38.6831447254874,0.900000000000005));
#48007=CARTESIAN_POINT('Ctrl Pts',(2.33231184184216,-38.8363876603691,0.900000000000005));
#48008=CARTESIAN_POINT('Ctrl Pts',(2.09999999999999,-38.98961400168,0.900000000000005));
#48009=CARTESIAN_POINT('Origin',(2.79695964928958,0.,-2.35992055786324E-15));
#48010=CARTESIAN_POINT('Origin',(2.4484798246448,0.,-1.17996027893162E-15));
#48011=CARTESIAN_POINT('',(2.79695964929222,-34.3237608806509,-17.5283766998976));
#48012=CARTESIAN_POINT('Ctrl Pts',(2.1,-34.7379330218401,-17.7278314909114));
#48013=CARTESIAN_POINT('Ctrl Pts',(2.33231184115668,-34.5998808589838,-17.6613490732083));
#48014=CARTESIAN_POINT('Ctrl Pts',(2.56464811214891,-34.4618137452222,-17.5948594555287));
#48015=CARTESIAN_POINT('Ctrl Pts',(2.79695964929223,-34.3237608806521,-17.528376699898));
#48016=CARTESIAN_POINT('',(2.79695964929053,-24.7266590280245,-29.5627617796034));
#48017=CARTESIAN_POINT('Ctrl Pts',(2.79695964929223,-24.726659028024,-29.5627617796028));
#48018=CARTESIAN_POINT('Ctrl Pts',(2.56464811356494,-24.8221945739443,-29.6825595650238));
#48019=CARTESIAN_POINT('Ctrl Pts',(2.332311844067,-24.9177399805788,-29.8023697153893));
#48020=CARTESIAN_POINT('Ctrl Pts',(2.09999999999999,-25.0132750426772,-29.9221668941168));
#48021=CARTESIAN_POINT('Origin',(2.79695964928959,0.,-2.35992055786324E-15));
#48022=CARTESIAN_POINT('Origin',(2.44847982464479,0.,-1.17996027893162E-15));
#48023=CARTESIAN_POINT('',(2.79695964929221,-7.69627812998459,-37.7641609687218));
#48024=CARTESIAN_POINT('Ctrl Pts',(2.1,-7.79857020128637,-38.2123318159937));
#48025=CARTESIAN_POINT('Ctrl Pts',(2.33231183932665,-7.76447413308037,-38.0629471805858));
#48026=CARTESIAN_POINT('Ctrl Pts',(2.56464811125653,-7.73037437189952,-37.9135463651979));
#48027=CARTESIAN_POINT('Ctrl Pts',(2.79695964929222,-7.69627812998494,-37.764160968723));
#48028=CARTESIAN_POINT('',(2.79695964929052,7.69627812998506,-37.7641609687237));
#48029=CARTESIAN_POINT('Ctrl Pts',(2.79695964929222,7.69627812998493,-37.764160968723));
#48030=CARTESIAN_POINT('Ctrl Pts',(2.56464811136644,7.73037437188337,-37.9135463651272));
#48031=CARTESIAN_POINT('Ctrl Pts',(2.33231183953305,7.76447413305006,-38.062947180453));
#48032=CARTESIAN_POINT('Ctrl Pts',(2.1,7.79857020128636,-38.2123318159937));
#48033=CARTESIAN_POINT('Origin',(2.79695964928958,0.,-2.35992055786324E-15));
#48034=CARTESIAN_POINT('Origin',(2.44847982464479,0.,-1.17996027893162E-15));
#48035=CARTESIAN_POINT('',(2.79695964929221,24.7266590280233,-29.5627617796018));
#48036=CARTESIAN_POINT('Ctrl Pts',(2.09999999999998,25.0132750426771,-29.9221668941168));
#48037=CARTESIAN_POINT('Ctrl Pts',(2.33231183679977,24.9177399835673,-29.8023697191368));
#48038=CARTESIAN_POINT('Ctrl Pts',(2.56464811003171,24.8221945753973,-29.6825595668458));
#48039=CARTESIAN_POINT('Ctrl Pts',(2.79695964929221,24.726659028024,-29.5627617796029));
#48040=CARTESIAN_POINT('',(2.79695964929052,34.3237608806527,-17.5283766998984));
#48041=CARTESIAN_POINT('Ctrl Pts',(2.79695964929223,34.3237608806521,-17.5283766998981));
#48042=CARTESIAN_POINT('Ctrl Pts',(2.56464811211474,34.4618137452426,-17.5948594555385));
#48043=CARTESIAN_POINT('Ctrl Pts',(2.33231184104411,34.5998808590507,-17.6613490732405));
#48044=CARTESIAN_POINT('Ctrl Pts',(2.09999999999998,34.7379330218401,-17.7278314909114));
#48045=CARTESIAN_POINT('Origin',(2.79695964928958,0.,-2.35992055786324E-15));
#48046=CARTESIAN_POINT('Origin',(0.15,0.,0.));
#48047=CARTESIAN_POINT('',(0.,3.825,-4.68427400673863E-16));
#48048=CARTESIAN_POINT('Origin',(0.,0.,0.));
#48049=CARTESIAN_POINT('',(0.3,3.525,4.31687996699442E-16));
#48050=CARTESIAN_POINT('',(0.15,3.675,-4.50057698686652E-16));
#48051=CARTESIAN_POINT('',(0.3,-3.525,-4.31687996699442E-16));
#48052=CARTESIAN_POINT('Origin',(0.3,0.,0.));
#48053=CARTESIAN_POINT('Origin',(0.3,0.,0.));
#48054=CARTESIAN_POINT('Origin',(15.5,0.,0.));
#48055=CARTESIAN_POINT('',(30.7,3.525,-4.31687996699442E-16));
#48056=CARTESIAN_POINT('',(30.7,-3.525,-4.31687996699442E-16));
#48057=CARTESIAN_POINT('Origin',(30.7,0.,0.));
#48058=CARTESIAN_POINT('Origin',(30.7,0.,0.));
#48059=CARTESIAN_POINT('',(15.5,-3.525,-4.31687996699442E-16));
#48060=CARTESIAN_POINT('Origin',(0.,38.5,0.));
#48061=CARTESIAN_POINT('',(-1.76941794549634E-15,-38.5,-4.71489017671731E-15));
#48062=CARTESIAN_POINT('Origin',(0.,0.,0.));
#48063=CARTESIAN_POINT('Origin',(30.85,0.,0.));
#48064=CARTESIAN_POINT('',(31.,3.825,4.68427400673863E-16));
#48065=CARTESIAN_POINT('',(30.85,3.675,-4.50057698686652E-16));
#48066=CARTESIAN_POINT('Origin',(31.,0.,0.));
#48067=CARTESIAN_POINT('Origin',(31.,3.525,0.));
#48068=CARTESIAN_POINT('',(31.,-8.1,-9.91963907309356E-16));
#48069=CARTESIAN_POINT('Origin',(31.,0.,0.));
#48070=CARTESIAN_POINT('Ctrl Pts',(2.09999999999999,14.6112236547299,-6.03746982408084));
#48071=CARTESIAN_POINT('Ctrl Pts',(2.73333333333332,14.6112236547299,-6.03746982408084));
#48072=CARTESIAN_POINT('Ctrl Pts',(3.36597343453743,14.6111769235222,-6.03754613131406));
#48073=CARTESIAN_POINT('Ctrl Pts',(4.12348633489348,14.6111625044228,-6.03756948056199));
#48074=CARTESIAN_POINT('Ctrl Pts',(4.36308027105789,14.6119257809318,-6.03577528532447));
#48075=CARTESIAN_POINT('Ctrl Pts',(4.85756641340223,14.6154583824993,-6.02750324329286));
#48076=CARTESIAN_POINT('Ctrl Pts',(5.73898730352466,14.6238809423774,-6.00782933213849));
#48077=CARTESIAN_POINT('Ctrl Pts',(6.52605696873204,14.624130981059,-6.00728042336119));
#48078=CARTESIAN_POINT('Ctrl Pts',(7.12756844447777,14.6083641562831,-6.04373935409524));
#48079=CARTESIAN_POINT('Ctrl Pts',(7.25506380614844,14.6049954548641,-6.05175896636988));
#48080=CARTESIAN_POINT('Ctrl Pts',(7.51732261094449,14.5977124647127,-6.06955193187746));
#48081=CARTESIAN_POINT('Ctrl Pts',(7.84589041574969,14.587687697552,-6.09468228112985));
#48082=CARTESIAN_POINT('Ctrl Pts',(8.24416928267873,14.5733864041206,-6.13057543333643));
#48083=CARTESIAN_POINT('Ctrl Pts',(8.77646956832262,14.5502471322405,-6.18743923585914));
#48084=CARTESIAN_POINT('Ctrl Pts',(9.44114040292177,14.5118316236054,-6.2778654600114));
#48085=CARTESIAN_POINT('Ctrl Pts',(9.96389116987696,14.4664252137994,-6.37698251721559));
#48086=CARTESIAN_POINT('Ctrl Pts',(11.1189200235608,14.3421195663292,-6.63780334583202));
#48087=CARTESIAN_POINT('Ctrl Pts',(12.080462017836,14.1753483064828,-7.00505140121598));
#48088=CARTESIAN_POINT('Ctrl Pts',(13.000848435547,13.9645576242428,-7.40476609777859));
#48089=CARTESIAN_POINT('Ctrl Pts',(13.2108249725339,13.9139023822834,-7.49752063559415));
#48090=CARTESIAN_POINT('Ctrl Pts',(13.3144480846626,13.8882765069648,-7.54353000870038));
#48091=CARTESIAN_POINT('Ctrl Pts',(13.3733279376354,13.8735399120439,-7.56972314538053));
#48092=CARTESIAN_POINT('Ctrl Pts',(13.4026071886664,13.866154080108,-7.58276112712036));
#48093=CARTESIAN_POINT('Ctrl Pts',(13.6877972600753,13.7939115032282,-7.70979028654145));
#48094=CARTESIAN_POINT('Ctrl Pts',(14.2465878522009,13.6358858928993,-7.98289947471341));
#48095=CARTESIAN_POINT('Ctrl Pts',(14.7537307590314,13.4638747656086,-8.2672884323285));
#48096=CARTESIAN_POINT('Ctrl Pts',(14.9999999999997,13.3740441878645,-8.41111991756525));
#48097=CARTESIAN_POINT('Ctrl Pts',(2.09999999999999,21.5804981880614,-9.39369555083498));
#48098=CARTESIAN_POINT('Ctrl Pts',(2.73333333333332,21.5804981880614,-9.39369555083498));
#48099=CARTESIAN_POINT('Ctrl Pts',(3.36558891350101,21.5804658214384,-9.39375443622592));
#48100=CARTESIAN_POINT('Ctrl Pts',(4.12268626532888,21.5804565789739,-9.39377109990644));
#48101=CARTESIAN_POINT('Ctrl Pts',(4.35700014090232,21.5816310465459,-9.39115328711438));
#48102=CARTESIAN_POINT('Ctrl Pts',(4.84800441917692,21.5871007298261,-9.37899529561417));
#48103=CARTESIAN_POINT('Ctrl Pts',(5.73069087778663,21.6002069847704,-9.34990650206829));
#48104=CARTESIAN_POINT('Ctrl Pts',(6.53595444290035,21.600798556951,-9.34867422602377));
#48105=CARTESIAN_POINT('Ctrl Pts',(7.15870824265195,21.5757953532485,-9.40377866208819));
#48106=CARTESIAN_POINT('Ctrl Pts',(7.28653324723265,21.57054842124,-9.41564402172901));
#48107=CARTESIAN_POINT('Ctrl Pts',(7.55249732957637,21.559112869562,-9.44216595644569));
#48108=CARTESIAN_POINT('Ctrl Pts',(7.88542376807474,21.5433748133556,-9.47959115917565));
#48109=CARTESIAN_POINT('Ctrl Pts',(8.29077837198509,21.5208373497423,-9.53321806687483));
#48110=CARTESIAN_POINT('Ctrl Pts',(8.83404956052536,21.4843659597635,-9.61829685598639));
#48111=CARTESIAN_POINT('Ctrl Pts',(9.5159951101198,21.4237193349165,-9.75404701204542));
#48112=CARTESIAN_POINT('Ctrl Pts',(10.0563165509726,21.3519772919284,-9.90350937303449));
#48113=CARTESIAN_POINT('Ctrl Pts',(11.2545453599662,21.1552727776615,-10.2981908568203));
#48114=CARTESIAN_POINT('Ctrl Pts',(12.2342091233032,20.8928382426908,-10.8482812877152));
#48115=CARTESIAN_POINT('Ctrl Pts',(13.1608025627428,20.5657221228123,-11.4401088273015));
#48116=CARTESIAN_POINT('Ctrl Pts',(13.3719027697888,20.4872597464373,-11.5772900925882));
#48117=CARTESIAN_POINT('Ctrl Pts',(13.4759508814436,20.4476142846892,-11.645264020493));
#48118=CARTESIAN_POINT('Ctrl Pts',(13.5350545696212,20.4248270188077,-11.6839493266396));
#48119=CARTESIAN_POINT('Ctrl Pts',(13.5644244680613,20.4134100716287,-11.7031984428001));
#48120=CARTESIAN_POINT('Ctrl Pts',(13.8509114235667,20.3017947915021,-11.8907413232488));
#48121=CARTESIAN_POINT('Ctrl Pts',(14.415914571976,20.056573473436,-12.2967435659359));
#48122=CARTESIAN_POINT('Ctrl Pts',(14.9236315787721,19.7920103236355,-12.7155432366557));
#48123=CARTESIAN_POINT('Ctrl Pts',(15.169681381964,19.6539784037027,-12.9272062682979));
#48124=CARTESIAN_POINT('Ctrl Pts',(2.09999999999999,28.5497727213929,-12.7499212775891));
#48125=CARTESIAN_POINT('Ctrl Pts',(2.73333333333333,28.5497727213929,-12.7499212775891));
#48126=CARTESIAN_POINT('Ctrl Pts',(3.36511943232413,28.5497117328892,-12.7500211136887));
#48127=CARTESIAN_POINT('Ctrl Pts',(4.12177605163342,28.5496942241346,-12.7500491269374));
#48128=CARTESIAN_POINT('Ctrl Pts',(4.35079752926905,28.5512513366179,-12.7466643375223));
#48129=CARTESIAN_POINT('Ctrl Pts',(4.83833431769655,28.5586001656638,-12.7307346947286));
#48130=CARTESIAN_POINT('Ctrl Pts',(5.72217414447527,28.5763905635329,-12.6922206715534));
#48131=CARTESIAN_POINT('Ctrl Pts',(6.54572412381037,28.5774814580578,-12.6899292527909));
#48132=CARTESIAN_POINT('Ctrl Pts',(7.18904210034709,28.5423219642133,-12.7655627019458));
#48133=CARTESIAN_POINT('Ctrl Pts',(7.31718028521341,28.5351786226866,-12.7813084572508));
#48134=CARTESIAN_POINT('Ctrl Pts',(7.58671228378742,28.5194164265744,-12.8169133627186));
#48135=CARTESIAN_POINT('Ctrl Pts',(7.92374360970041,28.4977092314406,-12.8671381009231));
#48136=CARTESIAN_POINT('Ctrl Pts',(8.33571576942014,28.4664978281724,-12.9393795360026));
#48137=CARTESIAN_POINT('Ctrl Pts',(8.88882961906569,28.4158479121591,-13.0543369931349));
#48138=CARTESIAN_POINT('Ctrl Pts',(9.58537985183176,28.3313660942903,-13.2385440053529));
#48139=CARTESIAN_POINT('Ctrl Pts',(10.1375678596739,28.2311944046601,-13.4422863994001));
#48140=CARTESIAN_POINT('Ctrl Pts',(11.3565453181114,27.957090325248,-13.9798088000628));
#48141=CARTESIAN_POINT('Ctrl Pts',(12.3228303493508,27.6006442853792,-14.7079674952598));
#48142=CARTESIAN_POINT('Ctrl Pts',(13.2438483912537,27.1599995484332,-15.4865968272217));
#48143=CARTESIAN_POINT('Ctrl Pts',(13.4536944920046,27.0542012023204,-15.6672854112189));
#48144=CARTESIAN_POINT('Ctrl Pts',(13.5572580689388,27.0007587325336,-15.7568001585971));
#48145=CARTESIAN_POINT('Ctrl Pts',(13.6160973314722,26.9700347789253,-15.8077582507674));
#48146=CARTESIAN_POINT('Ctrl Pts',(13.6453544897111,26.9546407543076,-15.8331157119274));
#48147=CARTESIAN_POINT('Ctrl Pts',(13.9304416541416,26.8041428578028,-16.0801826875383));
#48148=CARTESIAN_POINT('Ctrl Pts',(14.483478725475,26.4781781617783,-16.6086828302805));
#48149=CARTESIAN_POINT('Ctrl Pts',(14.98335392639,26.1263733010219,-17.1544773738691));
#48150=CARTESIAN_POINT('Ctrl Pts',(15.2260186760796,25.9428548705627,-17.4304534957912));
#48151=CARTESIAN_POINT('Ctrl Pts',(2.09999999999999,35.5190472547244,-16.1061470043432));
#48152=CARTESIAN_POINT('Ctrl Pts',(2.73333333333332,35.5190472547244,-16.1061470043432));
#48153=CARTESIAN_POINT('Ctrl Pts',(3.36464113820893,35.5189727539756,-16.1062575345791));
#48154=CARTESIAN_POINT('Ctrl Pts',(4.12085892726248,35.5189516907951,-16.1062875245081));
#48155=CARTESIAN_POINT('Ctrl Pts',(4.34457524717165,35.5208691650184,-16.1021819509952));
#48156=CARTESIAN_POINT('Ctrl Pts',(4.82871845463999,35.5300474198351,-16.0825848866187));
#48157=CARTESIAN_POINT('Ctrl Pts',(5.71350765111191,35.5525576262045,-16.0345705772587));
#48158=CARTESIAN_POINT('Ctrl Pts',(6.55584676521418,35.554338196091,-16.0308300205147));
#48159=CARTESIAN_POINT('Ctrl Pts',(7.21833787782939,35.5083038396895,-16.1284788337185));
#48160=CARTESIAN_POINT('Ctrl Pts',(7.346759957141,35.4992519242509,-16.1481285109658));
#48161=CARTESIAN_POINT('Ctrl Pts',(7.61957159600264,35.4790301677304,-16.1930875893086));
#48162=CARTESIAN_POINT('Ctrl Pts',(7.96026026202707,35.4511934320212,-16.2564362933882));
#48163=CARTESIAN_POINT('Ctrl Pts',(8.37794277256449,35.4110314107648,-16.3478471230923));
#48164=CARTESIAN_POINT('Ctrl Pts',(8.9389782770839,35.3458167429133,-16.4934464019928));
#48165=CARTESIAN_POINT('Ctrl Pts',(9.64589477564363,35.2370478008634,-16.7269630290823));
#48166=CARTESIAN_POINT('Ctrl Pts',(10.2035813464951,35.108934215722,-16.9839479337664));
#48167=CARTESIAN_POINT('Ctrl Pts',(11.4269751522422,34.7615504456458,-17.6561879421533));
#48168=CARTESIAN_POINT('Ctrl Pts',(12.379460225573,34.3187345767276,-18.5489901686144));
#48169=CARTESIAN_POINT('Ctrl Pts',(13.2972790827102,33.7671525002472,-19.5115445485323));
#48170=CARTESIAN_POINT('Ctrl Pts',(13.5062482901107,33.6346179543458,-19.7350483549094));
#48171=CARTESIAN_POINT('Ctrl Pts',(13.609520849881,33.5676140087591,-19.8458826806856));
#48172=CARTESIAN_POINT('Ctrl Pts',(13.6681938694708,33.5290848496294,-19.9089910815554));
#48173=CARTESIAN_POINT('Ctrl Pts',(13.6973863580761,33.5097717745622,-19.9404093800206));
#48174=CARTESIAN_POINT('Ctrl Pts',(13.9814817294285,33.3210758935383,-20.246334342403));
#48175=CARTESIAN_POINT('Ctrl Pts',(14.5280929602068,32.9176301874376,-20.8932115622066));
#48176=CARTESIAN_POINT('Ctrl Pts',(15.0243070371674,32.4796582872443,-21.5656339098325));
#48177=CARTESIAN_POINT('Ctrl Pts',(15.2656150130537,32.2510375008716,-21.9059812809209));
#48178=CARTESIAN_POINT('',(3.2,34.2572188230213,-15.4984824583453));
#48179=CARTESIAN_POINT('Ctrl Pts',(3.19847278576198,34.2571711264119,-15.4985541028447));
#48180=CARTESIAN_POINT('Ctrl Pts',(3.06436527352304,34.5398342174301,-15.634660914804));
#48181=CARTESIAN_POINT('Ctrl Pts',(2.93026063537424,34.8224448608797,-15.7707419629102));
#48182=CARTESIAN_POINT('Ctrl Pts',(2.79626448778338,35.1047282825352,-15.9066674709291));
#48183=CARTESIAN_POINT('',(15.,13.3740441878754,-8.41111991757311));
#48184=CARTESIAN_POINT('Ctrl Pts',(15.,13.3740441878754,-8.4111199175731));
#48185=CARTESIAN_POINT('Ctrl Pts',(14.489716577952,14.0152467731085,-8.4300414728713));
#48186=CARTESIAN_POINT('Ctrl Pts',(13.9833803026617,14.6726092024603,-8.46600373582148));
#48187=CARTESIAN_POINT('Ctrl Pts',(13.4460287676664,15.3890150736474,-8.54665853696435));
#48188=CARTESIAN_POINT('Ctrl Pts',(12.8282655681106,16.2126270936056,-8.63938287991053));
#48189=CARTESIAN_POINT('Ctrl Pts',(12.15554140896,17.1699136521334,-8.74804283511199));
#48190=CARTESIAN_POINT('Ctrl Pts',(11.5904908073768,18.0034501560149,-8.88551170505054));
#48191=CARTESIAN_POINT('Ctrl Pts',(11.1143368259707,18.7058504788506,-9.00135327668543));
#48192=CARTESIAN_POINT('Ctrl Pts',(10.6953158949628,19.3440146215797,-9.13525382272217));
#48193=CARTESIAN_POINT('Ctrl Pts',(10.2957959918397,19.9646028342318,-9.29767556265455));
#48194=CARTESIAN_POINT('Ctrl Pts',(10.0450888109117,20.3540350504866,-9.39959863637766));
#48195=CARTESIAN_POINT('Ctrl Pts',(9.80235305575949,20.7368803031962,-9.51197737039024));
#48196=CARTESIAN_POINT('Ctrl Pts',(9.56010106225058,21.126456560068,-9.63522432833226));
#48197=CARTESIAN_POINT('Ctrl Pts',(9.36613602928155,21.4383803977775,-9.73390504469829));
#48198=CARTESIAN_POINT('Ctrl Pts',(9.15248571275793,21.7859099736338,-9.84905754737758));
#48199=CARTESIAN_POINT('Ctrl Pts',(8.89022359798878,22.224537051038,-10.0043869244452));
#48200=CARTESIAN_POINT('Ctrl Pts',(8.39222406084267,23.0574292959559,-10.2993359602714));
#48201=CARTESIAN_POINT('Ctrl Pts',(7.76643777362598,24.1441485719301,-10.7202076897158));
#48202=CARTESIAN_POINT('Ctrl Pts',(7.10363554123529,25.4084375301613,-11.2437787818133));
#48203=CARTESIAN_POINT('Ctrl Pts',(6.23550018248562,27.0643974751934,-11.9295498243014));
#48204=CARTESIAN_POINT('Ctrl Pts',(5.31040885822318,28.970129103298,-12.9104863534632));
#48205=CARTESIAN_POINT('Ctrl Pts',(4.4641661690363,30.9938896521179,-13.9169531085495));
#48206=CARTESIAN_POINT('Ctrl Pts',(4.30741751124025,31.3687487247947,-14.1033799043044));
#48207=CARTESIAN_POINT('Ctrl Pts',(4.15262292088818,31.7490527468619,-14.2906133363129));
#48208=CARTESIAN_POINT('Ctrl Pts',(4.,32.1353158291841,-14.4766278329416));
#48209=CARTESIAN_POINT('Ctrl Pts',(3.72434973283399,32.832940545176,-14.8125861896161));
#48210=CARTESIAN_POINT('Ctrl Pts',(3.45587123478805,33.5452450424059,-15.1556139563445));
#48211=CARTESIAN_POINT('Ctrl Pts',(3.2,34.2572188230213,-15.4984824583453));
#48212=CARTESIAN_POINT('',(15.,25.5672208319352,-16.8130074326712));
#48213=CARTESIAN_POINT('Ctrl Pts',(15.,25.5672208319352,-16.8130074326712));
#48214=CARTESIAN_POINT('Ctrl Pts',(15.,21.9230552541059,-14.3215404573318));
#48215=CARTESIAN_POINT('Ctrl Pts',(15.,17.6025615780812,-11.3562169657429));
#48216=CARTESIAN_POINT('Ctrl Pts',(15.,13.3740441878754,-8.4111199175731));
#48217=CARTESIAN_POINT('Ctrl Pts',(6.,35.548403009865,-16.0409177869666));
#48218=CARTESIAN_POINT('Ctrl Pts',(6.38595465246567,35.0644728080463,-15.8087503789144));
#48219=CARTESIAN_POINT('Ctrl Pts',(6.7702364866826,34.6013428262183,-15.6121364414844));
#48220=CARTESIAN_POINT('Ctrl Pts',(7.13915213286206,34.1637499212586,-15.4654822405443));
#48221=CARTESIAN_POINT('Ctrl Pts',(8.10667920093238,33.0161082185314,-15.0808633973879));
#48222=CARTESIAN_POINT('Ctrl Pts',(8.9801988874737,32.1046384518045,-14.8985993430622));
#48223=CARTESIAN_POINT('Ctrl Pts',(9.46656009721077,31.5983922040242,-14.8470136927622));
#48224=CARTESIAN_POINT('Ctrl Pts',(9.65648624874913,31.4007008593061,-14.8268692736762));
#48225=CARTESIAN_POINT('Ctrl Pts',(9.79228848853731,31.2605649744979,-14.8192547892488));
#48226=CARTESIAN_POINT('Ctrl Pts',(9.9459382572782,31.1021220893961,-14.8158457576554));
#48227=CARTESIAN_POINT('Ctrl Pts',(10.1065740866009,30.9364752130151,-14.812281726146));
#48228=CARTESIAN_POINT('Ctrl Pts',(10.2660951669675,30.7723740544135,-14.8158872980242));
#48229=CARTESIAN_POINT('Ctrl Pts',(10.4261869573616,30.6070683865717,-14.8277509886845));
#48230=CARTESIAN_POINT('Ctrl Pts',(10.8065549509411,30.2143125491269,-14.855938369198));
#48231=CARTESIAN_POINT('Ctrl Pts',(11.1894211925257,29.814522907984,-14.9318211767803));
#48232=CARTESIAN_POINT('Ctrl Pts',(11.6023503255242,29.3751640250925,-15.0597901114669));
#48233=CARTESIAN_POINT('Ctrl Pts',(11.7531893954247,29.2146704198904,-15.1065359415422));
#48234=CARTESIAN_POINT('Ctrl Pts',(11.9080270687775,29.0488883179913,-15.160381650937));
#48235=CARTESIAN_POINT('Ctrl Pts',(12.0681766131679,28.8762440451095,-15.2218090966442));
#48236=CARTESIAN_POINT('Ctrl Pts',(12.1838435903474,28.7515528307349,-15.2661746737544));
#48237=CARTESIAN_POINT('Ctrl Pts',(12.3100865410161,28.615150802675,-15.3162188040206));
#48238=CARTESIAN_POINT('Ctrl Pts',(12.5127093730712,28.3942307654713,-15.40558106561));
#48239=CARTESIAN_POINT('Ctrl Pts',(12.7975492664042,28.0836693188959,-15.5312033205206));
#48240=CARTESIAN_POINT('Ctrl Pts',(13.1874566943566,27.6537578160352,-15.7216404803685));
#48241=CARTESIAN_POINT('Ctrl Pts',(13.6431584568239,27.1503653567254,-15.9585907359883));
#48242=CARTESIAN_POINT('Ctrl Pts',(14.069523646534,26.6793796395533,-16.1802869175923));
#48243=CARTESIAN_POINT('Ctrl Pts',(14.53311408767,26.1415317826733,-16.4743245564268));
#48244=CARTESIAN_POINT('Ctrl Pts',(15.,25.5672208319352,-16.8130074326712));
#48245=CARTESIAN_POINT('Origin',(15.,5.29966331579923,-6.64556760097826));
#48246=CARTESIAN_POINT('',(15.,12.0570237116074,-10.2098078054769));
#48247=CARTESIAN_POINT('Ctrl Pts',(15.,12.0570237116074,-10.2098078054769));
#48248=CARTESIAN_POINT('Ctrl Pts',(15.,12.5369574853615,-9.64304171150107));
#48249=CARTESIAN_POINT('Ctrl Pts',(15.,12.9772113127979,-9.04210133960708));
#48250=CARTESIAN_POINT('Ctrl Pts',(15.,13.3740441878754,-8.41111991757311));
#48251=CARTESIAN_POINT('',(15.,23.7252887774277,-19.3253893215031));
#48252=CARTESIAN_POINT('Ctrl Pts',(15.,12.0570237116074,-10.2098078054769));
#48253=CARTESIAN_POINT('Ctrl Pts',(15.,16.2510705543726,-13.4474144076022));
#48254=CARTESIAN_POINT('Ctrl Pts',(15.,20.4525997527948,-16.7472443383594));
#48255=CARTESIAN_POINT('Ctrl Pts',(15.,23.7252887774277,-19.325389321503));
#48256=CARTESIAN_POINT('Origin',(15.,0.,0.));
#48257=CARTESIAN_POINT('Ctrl Pts',(15.,19.0787879368772,-23.9240433635217));
#48258=CARTESIAN_POINT('Ctrl Pts',(15.,43.0028313003989,-4.84525542664447));
#48259=CARTESIAN_POINT('Ctrl Pts',(15.,23.9240433635217,19.0787879368772));
#48260=CARTESIAN_POINT('Ctrl Pts',(15.,4.84525542664447,43.0028313003989));
#48261=CARTESIAN_POINT('Ctrl Pts',(15.,-19.0787879368772,23.9240433635217));
#48262=CARTESIAN_POINT('Ctrl Pts',(15.,-43.0028313003989,4.84525542664447));
#48263=CARTESIAN_POINT('Ctrl Pts',(15.,-23.9240433635217,-19.0787879368772));
#48264=CARTESIAN_POINT('Ctrl Pts',(15.,-4.84525542664447,-43.0028313003989));
#48265=CARTESIAN_POINT('Ctrl Pts',(15.,19.0787879368772,-23.9240433635217));
#48266=CARTESIAN_POINT('Ctrl Pts',(14.7843073131059,19.1634046954076,-24.0301494226203));
#48267=CARTESIAN_POINT('Ctrl Pts',(14.7843073131059,43.1935541180279,-4.86674472721276));
#48268=CARTESIAN_POINT('Ctrl Pts',(14.7843073131059,24.0301494226203,19.1634046954076));
#48269=CARTESIAN_POINT('Ctrl Pts',(14.7843073131059,4.86674472721276,43.1935541180279));
#48270=CARTESIAN_POINT('Ctrl Pts',(14.7843073131059,-19.1634046954076,24.0301494226203));
#48271=CARTESIAN_POINT('Ctrl Pts',(14.7843073131059,-43.1935541180279,4.86674472721276));
#48272=CARTESIAN_POINT('Ctrl Pts',(14.7843073131059,-24.0301494226203,-19.1634046954076));
#48273=CARTESIAN_POINT('Ctrl Pts',(14.7843073131059,-4.86674472721276,-43.1935541180279));
#48274=CARTESIAN_POINT('Ctrl Pts',(14.7843073131059,19.1634046954076,-24.0301494226203));
#48275=CARTESIAN_POINT('Ctrl Pts',(14.3560298066371,19.3343909497437,-24.2445594038433));
#48276=CARTESIAN_POINT('Ctrl Pts',(14.3560298066371,43.578950353587,-4.91016845409964));
#48277=CARTESIAN_POINT('Ctrl Pts',(14.3560298066371,24.2445594038433,19.3343909497437));
#48278=CARTESIAN_POINT('Ctrl Pts',(14.3560298066371,4.91016845409964,43.578950353587));
#48279=CARTESIAN_POINT('Ctrl Pts',(14.3560298066371,-19.3343909497437,24.2445594038433));
#48280=CARTESIAN_POINT('Ctrl Pts',(14.3560298066371,-43.578950353587,4.91016845409964));
#48281=CARTESIAN_POINT('Ctrl Pts',(14.3560298066371,-24.2445594038433,-19.3343909497437));
#48282=CARTESIAN_POINT('Ctrl Pts',(14.3560298066371,-4.91016845409964,-43.578950353587));
#48283=CARTESIAN_POINT('Ctrl Pts',(14.3560298066371,19.3343909497437,-24.2445594038433));
#48284=CARTESIAN_POINT('Ctrl Pts',(13.722936818686,19.5961283568486,-24.5727677312355));
#48285=CARTESIAN_POINT('Ctrl Pts',(13.722936818686,44.1688960880841,-4.97663937438695));
#48286=CARTESIAN_POINT('Ctrl Pts',(13.722936818686,24.5727677312355,19.5961283568486));
#48287=CARTESIAN_POINT('Ctrl Pts',(13.722936818686,4.97663937438695,44.1688960880841));
#48288=CARTESIAN_POINT('Ctrl Pts',(13.722936818686,-19.5961283568486,24.5727677312355));
#48289=CARTESIAN_POINT('Ctrl Pts',(13.722936818686,-44.1688960880841,4.97663937438695));
#48290=CARTESIAN_POINT('Ctrl Pts',(13.722936818686,-24.5727677312355,-19.5961283568486));
#48291=CARTESIAN_POINT('Ctrl Pts',(13.722936818686,-4.97663937438695,-44.1688960880841));
#48292=CARTESIAN_POINT('Ctrl Pts',(13.722936818686,19.5961283568486,-24.5727677312355));
#48293=CARTESIAN_POINT('Ctrl Pts',(12.8977690042853,19.9558022366521,-25.0237845110024));
#48294=CARTESIAN_POINT('Ctrl Pts',(12.8977690042853,44.9795867476544,-5.06798227435031));
#48295=CARTESIAN_POINT('Ctrl Pts',(12.8977690042853,25.0237845110024,19.9558022366521));
#48296=CARTESIAN_POINT('Ctrl Pts',(12.8977690042853,5.06798227435031,44.9795867476544));
#48297=CARTESIAN_POINT('Ctrl Pts',(12.8977690042853,-19.9558022366521,25.0237845110024));
#48298=CARTESIAN_POINT('Ctrl Pts',(12.8977690042853,-44.9795867476544,5.06798227435031));
#48299=CARTESIAN_POINT('Ctrl Pts',(12.8977690042853,-25.0237845110024,-19.9558022366521));
#48300=CARTESIAN_POINT('Ctrl Pts',(12.8977690042853,-5.06798227435031,-44.9795867476544));
#48301=CARTESIAN_POINT('Ctrl Pts',(12.8977690042853,19.9558022366521,-25.0237845110024));
#48302=CARTESIAN_POINT('Ctrl Pts',(11.9000549946031,20.4244261094473,-25.6114202607695));
#48303=CARTESIAN_POINT('Ctrl Pts',(11.9000549946031,46.0358463702168,-5.18699415132219));
#48304=CARTESIAN_POINT('Ctrl Pts',(11.9000549946031,25.6114202607695,20.4244261094473));
#48305=CARTESIAN_POINT('Ctrl Pts',(11.9000549946031,5.18699415132219,46.0358463702168));
#48306=CARTESIAN_POINT('Ctrl Pts',(11.9000549946031,-20.4244261094473,25.6114202607695));
#48307=CARTESIAN_POINT('Ctrl Pts',(11.9000549946031,-46.0358463702168,5.18699415132219));
#48308=CARTESIAN_POINT('Ctrl Pts',(11.9000549946031,-25.6114202607695,-20.4244261094473));
#48309=CARTESIAN_POINT('Ctrl Pts',(11.9000549946031,-5.18699415132219,-46.0358463702168));
#48310=CARTESIAN_POINT('Ctrl Pts',(11.9000549946031,20.4244261094473,-25.6114202607695));
#48311=CARTESIAN_POINT('Ctrl Pts',(10.9391333834985,20.9137997124663,-26.2250753492544));
#48312=CARTESIAN_POINT('Ctrl Pts',(10.9391333834985,47.1388750617207,-5.3112756367881));
#48313=CARTESIAN_POINT('Ctrl Pts',(10.9391333834985,26.2250753492544,20.9137997124663));
#48314=CARTESIAN_POINT('Ctrl Pts',(10.9391333834985,5.3112756367881,47.1388750617207));
#48315=CARTESIAN_POINT('Ctrl Pts',(10.9391333834985,-20.9137997124663,26.2250753492544));
#48316=CARTESIAN_POINT('Ctrl Pts',(10.9391333834985,-47.1388750617207,5.3112756367881));
#48317=CARTESIAN_POINT('Ctrl Pts',(10.9391333834985,-26.2250753492544,-20.9137997124663));
#48318=CARTESIAN_POINT('Ctrl Pts',(10.9391333834985,-5.3112756367881,-47.1388750617207));
#48319=CARTESIAN_POINT('Ctrl Pts',(10.9391333834985,20.9137997124663,-26.2250753492544));
#48320=CARTESIAN_POINT('Ctrl Pts',(10.0180552497783,21.4256437560905,-26.8669074790281));
#48321=CARTESIAN_POINT('Ctrl Pts',(10.0180552497783,48.2925512351186,-5.44126372293756));
#48322=CARTESIAN_POINT('Ctrl Pts',(10.0180552497783,26.8669074790281,21.4256437560905));
#48323=CARTESIAN_POINT('Ctrl Pts',(10.0180552497783,5.44126372293756,48.2925512351186));
#48324=CARTESIAN_POINT('Ctrl Pts',(10.0180552497783,-21.4256437560905,26.8669074790281));
#48325=CARTESIAN_POINT('Ctrl Pts',(10.0180552497783,-48.2925512351186,5.44126372293756));
#48326=CARTESIAN_POINT('Ctrl Pts',(10.0180552497783,-26.8669074790281,-21.4256437560905));
#48327=CARTESIAN_POINT('Ctrl Pts',(10.0180552497783,-5.44126372293756,-48.2925512351186));
#48328=CARTESIAN_POINT('Ctrl Pts',(10.0180552497783,21.4256437560905,-26.8669074790281));
#48329=CARTESIAN_POINT('Ctrl Pts',(9.13857394886632,21.9609470764246,-27.5381566113461));
#48330=CARTESIAN_POINT('Ctrl Pts',(9.13857394886632,49.4991036877707,-5.57720953492157));
#48331=CARTESIAN_POINT('Ctrl Pts',(9.13857394886632,27.5381566113461,21.9609470764246));
#48332=CARTESIAN_POINT('Ctrl Pts',(9.13857394886632,5.57720953492157,49.4991036877707));
#48333=CARTESIAN_POINT('Ctrl Pts',(9.13857394886632,-21.9609470764246,27.5381566113461));
#48334=CARTESIAN_POINT('Ctrl Pts',(9.13857394886632,-49.4991036877707,5.57720953492157));
#48335=CARTESIAN_POINT('Ctrl Pts',(9.13857394886632,-27.5381566113461,-21.9609470764246));
#48336=CARTESIAN_POINT('Ctrl Pts',(9.13857394886632,-5.57720953492157,-49.4991036877707));
#48337=CARTESIAN_POINT('Ctrl Pts',(9.13857394886632,21.9609470764246,-27.5381566113461));
#48338=CARTESIAN_POINT('Ctrl Pts',(8.29915429043693,22.5188438754702,-28.2377370698584));
#48339=CARTESIAN_POINT('Ctrl Pts',(8.29915429043693,50.7565809453286,-5.71889319438814));
#48340=CARTESIAN_POINT('Ctrl Pts',(8.29915429043693,28.2377370698584,22.5188438754702));
#48341=CARTESIAN_POINT('Ctrl Pts',(8.29915429043693,5.71889319438814,50.7565809453286));
#48342=CARTESIAN_POINT('Ctrl Pts',(8.29915429043693,-22.5188438754702,28.2377370698584));
#48343=CARTESIAN_POINT('Ctrl Pts',(8.29915429043693,-50.7565809453286,5.71889319438814));
#48344=CARTESIAN_POINT('Ctrl Pts',(8.29915429043693,-28.2377370698584,-22.5188438754702));
#48345=CARTESIAN_POINT('Ctrl Pts',(8.29915429043693,-5.71889319438814,-50.7565809453286));
#48346=CARTESIAN_POINT('Ctrl Pts',(8.29915429043693,22.5188438754702,-28.2377370698584));
#48347=CARTESIAN_POINT('Ctrl Pts',(7.4968190344241,23.0976550855257,-28.9635433702624));
#48348=CARTESIAN_POINT('Ctrl Pts',(7.4968190344241,52.0611984557881,-5.86588828473677));
#48349=CARTESIAN_POINT('Ctrl Pts',(7.4968190344241,28.9635433702624,23.0976550855257));
#48350=CARTESIAN_POINT('Ctrl Pts',(7.4968190344241,5.86588828473677,52.0611984557881));
#48351=CARTESIAN_POINT('Ctrl Pts',(7.4968190344241,-23.0976550855257,28.9635433702624));
#48352=CARTESIAN_POINT('Ctrl Pts',(7.4968190344241,-52.0611984557881,5.86588828473677));
#48353=CARTESIAN_POINT('Ctrl Pts',(7.4968190344241,-28.9635433702624,-23.0976550855257));
#48354=CARTESIAN_POINT('Ctrl Pts',(7.4968190344241,-5.86588828473677,-52.0611984557881));
#48355=CARTESIAN_POINT('Ctrl Pts',(7.4968190344241,23.0976550855257,-28.9635433702624));
#48356=CARTESIAN_POINT('Ctrl Pts',(6.88220761950379,23.5760760069919,-29.5634642304892));
#48357=CARTESIAN_POINT('Ctrl Pts',(6.88220761950379,53.1395402374811,-5.98738822349725));
#48358=CARTESIAN_POINT('Ctrl Pts',(6.88220761950379,29.5634642304892,23.5760760069919));
#48359=CARTESIAN_POINT('Ctrl Pts',(6.88220761950379,5.98738822349725,53.1395402374811));
#48360=CARTESIAN_POINT('Ctrl Pts',(6.88220761950379,-23.5760760069919,29.5634642304892));
#48361=CARTESIAN_POINT('Ctrl Pts',(6.88220761950379,-53.1395402374811,5.98738822349725));
#48362=CARTESIAN_POINT('Ctrl Pts',(6.88220761950379,-29.5634642304892,-23.5760760069919));
#48363=CARTESIAN_POINT('Ctrl Pts',(6.88220761950379,-5.98738822349725,-53.1395402374811));
#48364=CARTESIAN_POINT('Ctrl Pts',(6.88220761950379,23.5760760069919,-29.5634642304892));
#48365=CARTESIAN_POINT('Ctrl Pts',(6.43560997955544,23.9429907960904,-30.0235608233205));
#48366=CARTESIAN_POINT('Ctrl Pts',(6.43560997955544,53.9665516194108,-6.08057002723013));
#48367=CARTESIAN_POINT('Ctrl Pts',(6.43560997955544,30.0235608233205,23.9429907960904));
#48368=CARTESIAN_POINT('Ctrl Pts',(6.43560997955544,6.08057002723013,53.9665516194108));
#48369=CARTESIAN_POINT('Ctrl Pts',(6.43560997955544,-23.9429907960904,30.0235608233205));
#48370=CARTESIAN_POINT('Ctrl Pts',(6.43560997955544,-53.9665516194108,6.08057002723013));
#48371=CARTESIAN_POINT('Ctrl Pts',(6.43560997955544,-30.0235608233205,-23.9429907960904));
#48372=CARTESIAN_POINT('Ctrl Pts',(6.43560997955544,-6.08057002723013,-53.9665516194108));
#48373=CARTESIAN_POINT('Ctrl Pts',(6.43560997955544,23.9429907960904,-30.0235608233205));
#48374=CARTESIAN_POINT('Ctrl Pts',(6.14415685965718,24.1911416066824,-30.3347320975618));
#48375=CARTESIAN_POINT('Ctrl Pts',(6.14415685965718,54.5258737042442,-6.14359049087936));
#48376=CARTESIAN_POINT('Ctrl Pts',(6.14415685965718,30.3347320975618,24.1911416066824));
#48377=CARTESIAN_POINT('Ctrl Pts',(6.14415685965718,6.14359049087936,54.5258737042442));
#48378=CARTESIAN_POINT('Ctrl Pts',(6.14415685965718,-24.1911416066824,30.3347320975618));
#48379=CARTESIAN_POINT('Ctrl Pts',(6.14415685965718,-54.5258737042442,6.14359049087936));
#48380=CARTESIAN_POINT('Ctrl Pts',(6.14415685965718,-30.3347320975618,-24.1911416066824));
#48381=CARTESIAN_POINT('Ctrl Pts',(6.14415685965718,-6.14359049087936,-54.5258737042442));
#48382=CARTESIAN_POINT('Ctrl Pts',(6.14415685965718,24.1911416066824,-30.3347320975618));
#48383=CARTESIAN_POINT('Ctrl Pts',(6.,24.3161022724906,-30.4914278162532));
#48384=CARTESIAN_POINT('Ctrl Pts',(6.,54.8075300887437,-6.17532554376256));
#48385=CARTESIAN_POINT('Ctrl Pts',(6.,30.4914278162532,24.3161022724906));
#48386=CARTESIAN_POINT('Ctrl Pts',(6.,6.17532554376256,54.8075300887437));
#48387=CARTESIAN_POINT('Ctrl Pts',(6.,-24.3161022724906,30.4914278162532));
#48388=CARTESIAN_POINT('Ctrl Pts',(6.,-54.8075300887437,6.17532554376256));
#48389=CARTESIAN_POINT('Ctrl Pts',(6.,-30.4914278162532,-24.3161022724906));
#48390=CARTESIAN_POINT('Ctrl Pts',(6.,-6.17532554376256,-54.8075300887437));
#48391=CARTESIAN_POINT('Ctrl Pts',(6.,24.3161022724906,-30.4914278162532));
#48392=CARTESIAN_POINT('Ctrl Pts',(15.,23.7252887774277,-19.325389321503));
#48393=CARTESIAN_POINT('Ctrl Pts',(14.0108432136945,25.1521740518353,-18.5591233494113));
#48394=CARTESIAN_POINT('Ctrl Pts',(13.3692319443824,26.0528643724611,-18.0122505544342));
#48395=CARTESIAN_POINT('Ctrl Pts',(12.3476991724842,27.2927306683407,-17.513207272874));
#48396=CARTESIAN_POINT('Ctrl Pts',(12.0250187050191,27.6843780505438,-17.3555701183851));
#48397=CARTESIAN_POINT('Ctrl Pts',(11.6666317570709,28.1212453396965,-17.1859329169356));
#48398=CARTESIAN_POINT('Ctrl Pts',(11.3593868751765,28.4924330909458,-17.0579748855819));
#48399=CARTESIAN_POINT('Ctrl Pts',(10.6767716809131,29.3171120810883,-16.7736866790818));
#48400=CARTESIAN_POINT('Ctrl Pts',(10.1321636914397,29.9604578402936,-16.6234350371559));
#48401=CARTESIAN_POINT('Ctrl Pts',(9.56604173138329,30.6013476901181,-16.6023045952485));
#48402=CARTESIAN_POINT('Ctrl Pts',(9.34563078589195,30.8508683724488,-16.5940777801661));
#48403=CARTESIAN_POINT('Ctrl Pts',(9.1222295109871,31.1000191408333,-16.6060902380637));
#48404=CARTESIAN_POINT('Ctrl Pts',(8.88860711505303,31.3611956288477,-16.6356564204087));
#48405=CARTESIAN_POINT('Ctrl Pts',(8.75830600700764,31.506864821425,-16.6521467329269));
#48406=CARTESIAN_POINT('Ctrl Pts',(8.62340343546576,31.6574103159489,-16.6721496821304));
#48407=CARTESIAN_POINT('Ctrl Pts',(8.40819516300444,31.9000796698313,-16.7185585110703));
#48408=CARTESIAN_POINT('Ctrl Pts',(8.02443006829152,32.3328140926836,-16.8013159647219));
#48409=CARTESIAN_POINT('Ctrl Pts',(7.46417034513354,32.9699846210684,-16.9702026704623));
#48410=CARTESIAN_POINT('Ctrl Pts',(6.85957019142019,33.7100854539055,-17.2206111851372));
#48411=CARTESIAN_POINT('Ctrl Pts',(6.58024553736739,34.0520112834421,-17.3362996633883));
#48412=CARTESIAN_POINT('Ctrl Pts',(6.28976782192772,34.4070814189946,-17.4897602383325));
#48413=CARTESIAN_POINT('Ctrl Pts',(6.,34.7703877941326,-17.6640916167698));
#48414=CARTESIAN_POINT('Ctrl Pts',(2.09999999999998,13.8279757475969,-7.65812678728599));
#48415=CARTESIAN_POINT('Ctrl Pts',(2.73333333333332,13.8279757475969,-7.65812678728599));
#48416=CARTESIAN_POINT('Ctrl Pts',(3.36803303381851,13.8280015254532,-7.6580866539697));
#48417=CARTESIAN_POINT('Ctrl Pts',(4.25276872116174,13.8280168460333,-7.65806146044593));
#48418=CARTESIAN_POINT('Ctrl Pts',(4.77266573001516,13.8321785569649,-7.65073620619348));
#48419=CARTESIAN_POINT('Ctrl Pts',(5.76856597158111,13.844291616205,-7.62951788897893));
#48420=CARTESIAN_POINT('Ctrl Pts',(6.48508033865307,13.8440136699914,-7.630113273714));
#48421=CARTESIAN_POINT('Ctrl Pts',(6.99865791044875,13.827042724761,-7.65945876128045));
#48422=CARTESIAN_POINT('Ctrl Pts',(7.1247971738976,13.8228379227586,-7.66695269622797));
#48423=CARTESIAN_POINT('Ctrl Pts',(7.37169992327966,13.8141335684726,-7.68281784902541));
#48424=CARTESIAN_POINT('Ctrl Pts',(7.68210776228461,13.8021317972921,-7.70522099931852));
#48425=CARTESIAN_POINT('Ctrl Pts',(8.05073533832202,13.7852894828728,-7.73671249396138));
#48426=CARTESIAN_POINT('Ctrl Pts',(8.41503452625175,13.7653021081082,-7.77346916765258));
#48427=CARTESIAN_POINT('Ctrl Pts',(9.01074252234631,13.7255238371934,-7.84464976675126));
#48428=CARTESIAN_POINT('Ctrl Pts',(9.4630926264689,13.6818268405885,-7.91857147136531));
#48429=CARTESIAN_POINT('Ctrl Pts',(10.2678436967056,13.5747717426652,-8.08902421601531));
#48430=CARTESIAN_POINT('Ctrl Pts',(10.9804887503285,13.44484280776,-8.3071906299572));
#48431=CARTESIAN_POINT('Ctrl Pts',(11.7910213121199,13.2470722117918,-8.62018274307134));
#48432=CARTESIAN_POINT('Ctrl Pts',(12.2471503020159,13.1229490575071,-8.80658382774348));
#48433=CARTESIAN_POINT('Ctrl Pts',(12.4732466492024,13.0574621913427,-8.90089570339079));
#48434=CARTESIAN_POINT('Ctrl Pts',(12.8351179681746,12.9496826084397,-9.0521331140034));
#48435=CARTESIAN_POINT('Ctrl Pts',(13.2802512961797,12.802233799643,-9.25581954461894));
#48436=CARTESIAN_POINT('Ctrl Pts',(14.1612564878,12.4620169214753,-9.71481371470994));
#48437=CARTESIAN_POINT('Ctrl Pts',(14.7820737708942,12.1693147416513,-10.0825472947651));
#48438=CARTESIAN_POINT('Ctrl Pts',(15.1979896574214,11.9574529826808,-10.325659137886));
#48439=CARTESIAN_POINT('Ctrl Pts',(2.09999999999998,20.7979970457138,-11.014712137007));
#48440=CARTESIAN_POINT('Ctrl Pts',(2.73333333333332,20.7979970457138,-11.014712137007));
#48441=CARTESIAN_POINT('Ctrl Pts',(3.36871863447842,20.7979957888325,-11.0147100539278));
#48442=CARTESIAN_POINT('Ctrl Pts',(4.25415249655759,20.7980011101394,-11.014697259023));
#48443=CARTESIAN_POINT('Ctrl Pts',(4.78309467008275,20.8040276778098,-11.0036065611137));
#48444=CARTESIAN_POINT('Ctrl Pts',(5.77493400902691,20.821446583213,-10.9717244397128));
#48445=CARTESIAN_POINT('Ctrl Pts',(6.47496358572727,20.820810958958,-10.973026983233));
#48446=CARTESIAN_POINT('Ctrl Pts',(6.96726482620541,20.7970302031018,-11.0159800673788));
#48447=CARTESIAN_POINT('Ctrl Pts',(7.09308276047564,20.7909913536982,-11.0272323285292));
#48448=CARTESIAN_POINT('Ctrl Pts',(7.33628215808622,20.7786039277912,-11.0508651505887));
#48449=CARTESIAN_POINT('Ctrl Pts',(7.64235751563798,20.7615171715808,-11.0842742543889));
#48450=CARTESIAN_POINT('Ctrl Pts',(8.00391288520119,20.7376501778544,-11.1310547409347));
#48451=CARTESIAN_POINT('Ctrl Pts',(8.36000598692249,20.7093493502994,-11.1855823927471));
#48452=CARTESIAN_POINT('Ctrl Pts',(8.93967288853338,20.6532251446613,-11.2907675094849));
#48453=CARTESIAN_POINT('Ctrl Pts',(9.37528826459676,20.5916420820299,-11.3996398370039));
#48454=CARTESIAN_POINT('Ctrl Pts',(10.1433953963723,20.4417998065261,-11.6486751197096));
#48455=CARTESIAN_POINT('Ctrl Pts',(10.8342881133699,20.2594568751716,-11.969903308493));
#48456=CARTESIAN_POINT('Ctrl Pts',(11.6346763171622,19.9775507429201,-12.4374585345057));
#48457=CARTESIAN_POINT('Ctrl Pts',(12.087250380503,19.799601122098,-12.717071440536));
#48458=CARTESIAN_POINT('Ctrl Pts',(12.3122423823028,19.7053497381101,-12.8589426681667));
#48459=CARTESIAN_POINT('Ctrl Pts',(12.6725822269122,19.5499991694726,-13.0866433320915));
#48460=CARTESIAN_POINT('Ctrl Pts',(13.111012820426,19.339646719064,-13.3910169222338));
#48461=CARTESIAN_POINT('Ctrl Pts',(13.9921323132802,18.8489891102053,-14.0840049748908));
#48462=CARTESIAN_POINT('Ctrl Pts',(14.6125773377935,18.4239412983855,-14.6419209794113));
#48463=CARTESIAN_POINT('Ctrl Pts',(15.0291266285127,18.1158843190329,-15.0106560867984));
#48464=CARTESIAN_POINT('Ctrl Pts',(2.09999999999998,27.7680183438307,-14.371297486728));
#48465=CARTESIAN_POINT('Ctrl Pts',(2.73333333333332,27.7680183438307,-14.371297486728));
#48466=CARTESIAN_POINT('Ctrl Pts',(3.36945332065348,27.7680378208204,-14.3712683196438));
#48467=CARTESIAN_POINT('Ctrl Pts',(4.25561608029733,27.7680578943104,-14.3712329142362));
#48468=CARTESIAN_POINT('Ctrl Pts',(4.79358528048294,27.776050427636,-14.3561843266613));
#48469=CARTESIAN_POINT('Ctrl Pts',(5.78145895202477,27.798760568176,-14.3136731881339));
#48470=CARTESIAN_POINT('Ctrl Pts',(6.46486442188066,27.7976233124563,-14.3160366570693));
#48471=CARTESIAN_POINT('Ctrl Pts',(6.93654415129333,27.7679543062191,-14.370711304283));
#48472=CARTESIAN_POINT('Ctrl Pts',(7.06205598783357,27.7600999969903,-14.3856866007946));
#48473=CARTESIAN_POINT('Ctrl Pts',(7.30168699668564,27.7442029155811,-14.4167341707392));
#48474=CARTESIAN_POINT('Ctrl Pts',(7.6036656947927,27.7222916772868,-14.4606373100959));
#48475=CARTESIAN_POINT('Ctrl Pts',(7.95860291280678,27.6918305255677,-14.5218376687646));
#48476=CARTESIAN_POINT('Ctrl Pts',(8.307311571412,27.655870116953,-14.5928583523582));
#48477=CARTESIAN_POINT('Ctrl Pts',(8.87310312231183,27.5847261494896,-14.7294164513786));
#48478=CARTESIAN_POINT('Ctrl Pts',(9.29618304531655,27.5073149978084,-14.8693720517901));
#48479=CARTESIAN_POINT('Ctrl Pts',(10.0462726890403,27.3189544476347,-15.1893221911421));
#48480=CARTESIAN_POINT('Ctrl Pts',(10.740516903946,27.0847770091748,-15.6137212401067));
#48481=CARTESIAN_POINT('Ctrl Pts',(11.5482246043898,26.7159679112832,-16.241552115041));
#48482=CARTESIAN_POINT('Ctrl Pts',(12.0041796923629,26.4828720940238,-16.6169595466783));
#48483=CARTESIAN_POINT('Ctrl Pts',(12.2304128422418,26.3593556717716,-16.8073766296154));
#48484=CARTESIAN_POINT('Ctrl Pts',(12.5924521142123,26.1558011511038,-17.1128169167779));
#48485=CARTESIAN_POINT('Ctrl Pts',(13.0427789525575,25.8764554795404,-17.5278403254683));
#48486=CARTESIAN_POINT('Ctrl Pts',(13.9385896269168,25.2244859115221,-18.4699929405824));
#48487=CARTESIAN_POINT('Ctrl Pts',(14.5670688438605,24.6610742418818,-19.2247640399616));
#48488=CARTESIAN_POINT('Ctrl Pts',(14.9853697475044,24.254629587972,-19.7206424669413));
#48489=CARTESIAN_POINT('Ctrl Pts',(2.09999999999998,34.7380396419475,-17.727882836449));
#48490=CARTESIAN_POINT('Ctrl Pts',(2.73333333333332,34.7380396419475,-17.727882836449));
#48491=CARTESIAN_POINT('Ctrl Pts',(3.37020393653566,34.7380735049305,-17.7278392579628));
#48492=CARTESIAN_POINT('Ctrl Pts',(4.25711961877983,34.7381056827597,-17.7277866677452));
#48493=CARTESIAN_POINT('Ctrl Pts',(4.80402220532588,34.7481429814137,-17.7086154435085));
#48494=CARTESIAN_POINT('Ctrl Pts',(5.78813454502387,34.7761040328012,-17.6555601576571));
#48495=CARTESIAN_POINT('Ctrl Pts',(6.45445182277513,34.7742910555487,-17.6593420657212));
#48496=CARTESIAN_POINT('Ctrl Pts',(6.90690766682582,34.7394581505422,-17.7242403373792));
#48497=CARTESIAN_POINT('Ctrl Pts',(7.03214349859616,34.7298009507745,-17.7429143633733));
#48498=CARTESIAN_POINT('Ctrl Pts',(7.26849387006162,34.7105274847739,-17.781104666533));
#48499=CARTESIAN_POINT('Ctrl Pts',(7.56683268339157,34.683957518025,-17.8351670693613));
#48500=CARTESIAN_POINT('Ctrl Pts',(7.91604911717842,34.6471776150214,-17.9102341213459));
#48501=CARTESIAN_POINT('Ctrl Pts',(8.25884519308195,34.6038583650633,-17.99715521056));
#48502=CARTESIAN_POINT('Ctrl Pts',(8.814270992878,34.5181491335739,-18.1642080280054));
#48503=CARTESIAN_POINT('Ctrl Pts',(9.23053609210392,34.4249120745718,-18.3353270659959));
#48504=CARTESIAN_POINT('Ctrl Pts',(9.97649944922677,34.1947051258132,-18.7327306189381));
#48505=CARTESIAN_POINT('Ctrl Pts',(10.6790209735713,33.9025959931162,-19.2714823555945));
#48506=CARTESIAN_POINT('Ctrl Pts',(11.4920879596953,33.4429950265762,-20.065251397391));
#48507=CARTESIAN_POINT('Ctrl Pts',(11.9504408299826,33.1531140023176,-20.5385307869332));
#48508=CARTESIAN_POINT('Ctrl Pts',(12.1774708173222,32.9997497984637,-20.7780730187058));
#48509=CARTESIAN_POINT('Ctrl Pts',(12.5406713626334,32.7471412732904,-21.1620343438423));
#48510=CARTESIAN_POINT('Ctrl Pts',(12.997673300029,32.3954626109581,-21.6919929876177));
#48511=CARTESIAN_POINT('Ctrl Pts',(13.8993993294321,31.5803589389699,-22.8835829401895));
#48512=CARTESIAN_POINT('Ctrl Pts',(14.5324532885843,30.8775669453658,-23.8349298069317));
#48513=CARTESIAN_POINT('Ctrl Pts',(14.9514110803021,30.3723459825604,-24.457322833162));
#48514=CARTESIAN_POINT('',(3.2,33.4762280926097,-17.1202264205696));
#48515=CARTESIAN_POINT('Ctrl Pts',(3.2,33.4762280926097,-17.1202264205697));
#48516=CARTESIAN_POINT('Ctrl Pts',(3.5615227483539,32.470273991762,-16.6357844579161));
#48517=CARTESIAN_POINT('Ctrl Pts',(3.95224584525312,31.4490477361342,-16.1504264387208));
#48518=CARTESIAN_POINT('Ctrl Pts',(4.78767430123564,29.4297069892437,-15.1533367200056));
#48519=CARTESIAN_POINT('Ctrl Pts',(5.21513946231862,28.4699606481904,-14.6620752040124));
#48520=CARTESIAN_POINT('Ctrl Pts',(6.79548775402185,25.1212555511771,-13.012167423548));
#48521=CARTESIAN_POINT('Ctrl Pts',(7.9401629593867,23.0391778774888,-12.2240189743849));
#48522=CARTESIAN_POINT('Ctrl Pts',(9.46271935274971,20.413489232316,-11.3125228814697));
#48523=CARTESIAN_POINT('Ctrl Pts',(10.1385443659007,19.3034154994021,-11.0292622078652));
#48524=CARTESIAN_POINT('Ctrl Pts',(11.5967860400667,16.9862280609382,-10.6585988316486));
#48525=CARTESIAN_POINT('Ctrl Pts',(12.399735667707,15.7679338637663,-10.4920203380681));
#48526=CARTESIAN_POINT('Ctrl Pts',(13.6850585208124,13.8903785225595,-10.3029151929985));
#48527=CARTESIAN_POINT('Ctrl Pts',(14.3457395898618,12.9431348360658,-10.2602733177061));
#48528=CARTESIAN_POINT('Ctrl Pts',(15.,12.0570237116074,-10.2098078054769));
#48529=CARTESIAN_POINT('Ctrl Pts',(2.79814995341175,34.3237720576307,-17.5283618512166));
#48530=CARTESIAN_POINT('Ctrl Pts',(2.93286002554174,34.0413567394956,-17.3923509689602));
#48531=CARTESIAN_POINT('Ctrl Pts',(3.06772762579813,33.7587618460436,-17.2562524503664));
#48532=CARTESIAN_POINT('Ctrl Pts',(3.20257974079352,33.47625152623,-17.1201943222877));
#48533=CARTESIAN_POINT('Origin',(2.9,0.,0.));
#48534=CARTESIAN_POINT('',(3.2,24.1401481407882,-28.8273003894017));
#48535=CARTESIAN_POINT('Origin',(3.2,0.,0.));
#48536=CARTESIAN_POINT('Ctrl Pts',(3.19853209668272,24.1400733004768,-28.8273374408964));
#48537=CARTESIAN_POINT('Ctrl Pts',(3.06441460888704,24.3356896029093,-29.0726077758756));
#48538=CARTESIAN_POINT('Ctrl Pts',(2.93029925412543,24.5312702067218,-29.3178337273723));
#48539=CARTESIAN_POINT('Ctrl Pts',(2.79629300805566,24.7266240747468,-29.5627789633676));
#48540=CARTESIAN_POINT('Ctrl Pts',(2.09999999999999,4.38966495848408,-15.1878155149937));
#48541=CARTESIAN_POINT('Ctrl Pts',(2.73333333333332,4.38966495848408,-15.1878155149937));
#48542=CARTESIAN_POINT('Ctrl Pts',(3.36596254895254,4.38957946978066,-15.1878260991564));
#48543=CARTESIAN_POINT('Ctrl Pts',(4.12347126801082,4.38955322135183,-15.1878292451984));
#48544=CARTESIAN_POINT('Ctrl Pts',(4.36306410485066,4.39143213229248,-15.1873073007927));
#48545=CARTESIAN_POINT('Ctrl Pts',(4.85754827137282,4.40010260543508,-15.1849115824678));
#48546=CARTESIAN_POINT('Ctrl Pts',(5.73896685227764,4.42073647768525,-15.1792300101236));
#48547=CARTESIAN_POINT('Ctrl Pts',(6.52602599492339,4.42132553322825,-15.1790826820951));
#48548=CARTESIAN_POINT('Ctrl Pts',(7.12753345010613,4.38299182110871,-15.1894872387425));
#48549=CARTESIAN_POINT('Ctrl Pts',(7.25502865634115,4.37462153877536,-15.191853620938));
#48550=CARTESIAN_POINT('Ctrl Pts',(7.51728707570608,4.35616970860387,-15.1972532622203));
#48551=CARTESIAN_POINT('Ctrl Pts',(7.84585340416012,4.33027233957835,-15.2050840117294));
#48552=CARTESIAN_POINT('Ctrl Pts',(8.2441318948403,4.29329339033759,-15.2162818026573));
#48553=CARTESIAN_POINT('Ctrl Pts',(8.77643068220616,4.23440926929706,-15.2336446863811));
#48554=CARTESIAN_POINT('Ctrl Pts',(9.44110000562817,4.1397604107769,-15.2599899543444));
#48555=CARTESIAN_POINT('Ctrl Pts',(9.96384938741169,4.03395832280009,-15.2862881501386));
#48556=CARTESIAN_POINT('Ctrl Pts',(11.1188752712428,3.75254025914602,-15.3517209561057));
#48557=CARTESIAN_POINT('Ctrl Pts',(12.0804115271536,3.36144010237934,-15.4503087637338));
#48558=CARTESIAN_POINT('Ctrl Pts',(13.00080324578,2.91750211822961,-15.534724281135));
#48559=CARTESIAN_POINT('Ctrl Pts',(13.2107807208523,2.81340029136765,-15.5529519774906));
#48560=CARTESIAN_POINT('Ctrl Pts',(13.3144041536197,2.76145108518079,-15.5616032545832));
#48561=CARTESIAN_POINT('Ctrl Pts',(13.373284229634,2.73178424239228,-15.5664128874317));
#48562=CARTESIAN_POINT('Ctrl Pts',(13.4025633600174,2.7169858062115,-15.5687674529565));
#48563=CARTESIAN_POINT('Ctrl Pts',(13.6877617951153,2.57262378140117,-15.5914878140199));
#48564=CARTESIAN_POINT('Ctrl Pts',(14.2465713444148,2.26056171575794,-15.6382203410322));
#48565=CARTESIAN_POINT('Ctrl Pts',(14.7537307590314,1.9309622388219,-15.6810511943411));
#48566=CARTESIAN_POINT('Ctrl Pts',(14.9999999999997,1.76250180637518,-15.7004962848038));
#48567=CARTESIAN_POINT('Ctrl Pts',(2.09999999999999,6.11093362092453,-22.7291862684821));
#48568=CARTESIAN_POINT('Ctrl Pts',(2.73333333333332,6.11093362092453,-22.7291862684821));
#48569=CARTESIAN_POINT('Ctrl Pts',(3.3655737913602,6.11087106652427,-22.7291970270664));
#48570=CARTESIAN_POINT('Ctrl Pts',(4.12266523196545,6.11085340617054,-22.7291999896352));
#48571=CARTESIAN_POINT('Ctrl Pts',(4.3569775538667,6.11363264974669,-22.7284859949201));
#48572=CARTESIAN_POINT('Ctrl Pts',(4.84797905966998,6.12654915024314,-22.7251818552908));
#48573=CARTESIAN_POINT('Ctrl Pts',(5.73066233595544,6.15746420822384,-22.7172920110342));
#48574=CARTESIAN_POINT('Ctrl Pts',(6.53591128078968,6.15880152770652,-22.7169853053249));
#48575=CARTESIAN_POINT('Ctrl Pts',(7.15865947305896,6.10013179404174,-22.7317937279026));
#48576=CARTESIAN_POINT('Ctrl Pts',(7.28648425494255,6.08758374572187,-22.7350894297213));
#48577=CARTESIAN_POINT('Ctrl Pts',(7.55244779773386,6.05971829150288,-22.7426848792085));
#48578=CARTESIAN_POINT('Ctrl Pts',(7.88537213844326,6.02064645072765,-22.7537144590768));
#48579=CARTESIAN_POINT('Ctrl Pts',(8.29072621569934,5.96466756362568,-22.7695297564594));
#48580=CARTESIAN_POINT('Ctrl Pts',(8.83399521564723,5.87541197003736,-22.794060849192));
#48581=CARTESIAN_POINT('Ctrl Pts',(9.51593856281283,5.73146685019894,-22.831284068277));
#48582=CARTESIAN_POINT('Ctrl Pts',(10.0562578372541,5.56988387032315,-22.8683818954022));
#48583=CARTESIAN_POINT('Ctrl Pts',(11.2544819138336,5.13867129632783,-22.9606714121106));
#48584=CARTESIAN_POINT('Ctrl Pts',(12.2341371971438,4.54497963493266,-23.0984661085317));
#48585=CARTESIAN_POINT('Ctrl Pts',(13.1607383237085,3.8783134664302,-23.2117153171294));
#48586=CARTESIAN_POINT('Ctrl Pts',(13.3718398189947,3.72213984640676,-23.2359021626504));
#48587=CARTESIAN_POINT('Ctrl Pts',(13.4758883775225,3.64427692494074,-23.2472871755526));
#48588=CARTESIAN_POINT('Ctrl Pts',(13.5349923709208,3.59982374741586,-23.2535912907113));
#48589=CARTESIAN_POINT('Ctrl Pts',(13.5643621042971,3.57765592245332,-23.2566667766753));
#48590=CARTESIAN_POINT('Ctrl Pts',(13.8508605081462,3.36143178692841,-23.2863343991313));
#48591=CARTESIAN_POINT('Ctrl Pts',(14.4158889403965,2.89109929538129,-23.3477528779048));
#48592=CARTESIAN_POINT('Ctrl Pts',(14.9236315787721,2.39870457596863,-23.4020283054991));
#48593=CARTESIAN_POINT('Ctrl Pts',(15.169681381964,2.14715825974705,-23.4260803465695));
#48594=CARTESIAN_POINT('Ctrl Pts',(2.09999999999999,7.83220228336497,-30.2705570219704));
#48595=CARTESIAN_POINT('Ctrl Pts',(2.73333333333333,7.83220228336497,-30.2705570219704));
#48596=CARTESIAN_POINT('Ctrl Pts',(3.36510345911249,7.83209226044356,-30.270570640248));
#48597=CARTESIAN_POINT('Ctrl Pts',(4.1217534628143,7.83206130605595,-30.2705741234367));
#48598=CARTESIAN_POINT('Ctrl Pts',(4.35077319609568,7.83567895787034,-30.269681067371));
#48599=CARTESIAN_POINT('Ctrl Pts',(4.83830702967109,7.85271633513914,-30.2654944557726));
#48600=CARTESIAN_POINT('Ctrl Pts',(5.72214362909506,7.89392143672765,-30.2553902143163));
#48601=CARTESIAN_POINT('Ctrl Pts',(6.54567911469843,7.8964013330852,-30.2548130793221));
#48602=CARTESIAN_POINT('Ctrl Pts',(7.18899146074693,7.81535022009343,-30.2744804534963));
#48603=CARTESIAN_POINT('Ctrl Pts',(7.31712941776005,7.79858600371208,-30.2787128644861));
#48604=CARTESIAN_POINT('Ctrl Pts',(7.58666087185036,7.76092169042061,-30.2885887307684));
#48605=CARTESIAN_POINT('Ctrl Pts',(7.92369029396209,7.70812152044347,-30.3029317759761));
#48606=CARTESIAN_POINT('Ctrl Pts',(8.33566195251538,7.6321812153183,-30.3235714663787));
#48607=CARTESIAN_POINT('Ctrl Pts',(8.88877416188324,7.51072584522975,-30.3556463460423));
#48608=CARTESIAN_POINT('Ctrl Pts',(9.58532271430234,7.31403511981607,-30.4044467728404));
#48609=CARTESIAN_POINT('Ctrl Pts',(10.1375097070441,7.0922890814097,-30.4531604646358));
#48610=CARTESIAN_POINT('Ctrl Pts',(11.3564859597505,6.50114151522531,-30.5739966068883));
#48611=CARTESIAN_POINT('Ctrl Pts',(12.3227698011673,5.70961632447872,-30.749314104971));
#48612=CARTESIAN_POINT('Ctrl Pts',(13.2437945503543,4.82611747317232,-30.8902721426667));
#48613=CARTESIAN_POINT('Ctrl Pts',(13.4536418756815,4.61888452203683,-30.9202132651585));
#48614=CARTESIAN_POINT('Ctrl Pts',(13.5572058324948,4.51557794210463,-30.9342418296942));
#48615=CARTESIAN_POINT('Ctrl Pts',(13.616045355569,4.45658101854197,-30.9419927542262));
#48616=CARTESIAN_POINT('Ctrl Pts',(13.6453023755694,4.42715785743315,-30.9457673242247));
#48617=CARTESIAN_POINT('Ctrl Pts',(13.9303991372842,4.14015109313492,-30.9821481247373));
#48618=CARTESIAN_POINT('Ctrl Pts',(14.4834575035054,3.52369906436613,-31.0568154715655));
#48619=CARTESIAN_POINT('Ctrl Pts',(14.98335392639,2.87761683656506,-31.1220628682749));
#48620=CARTESIAN_POINT('Ctrl Pts',(15.2260186760796,2.54742814619257,-31.1506506793037));
#48621=CARTESIAN_POINT('Ctrl Pts',(2.09999999999999,9.55347094580542,-37.8119277754588));
#48622=CARTESIAN_POINT('Ctrl Pts',(2.73333333333332,9.55347094580542,-37.8119277754588));
#48623=CARTESIAN_POINT('Ctrl Pts',(3.3646253867,9.55334556061245,-37.8119373823181));
#48624=CARTESIAN_POINT('Ctrl Pts',(4.12083619687885,9.55331129117588,-37.8119392787534));
#48625=CARTESIAN_POINT('Ctrl Pts',(4.34455066434138,9.55771726793094,-37.8108785541332));
#48626=CARTESIAN_POINT('Ctrl Pts',(4.82869096816822,9.57876287103758,-37.8058356126046));
#48627=CARTESIAN_POINT('Ctrl Pts',(5.7134771442972,9.63033870088108,-37.7934981042942));
#48628=CARTESIAN_POINT('Ctrl Pts',(6.55580364168112,9.63438372222901,-37.7925563845865));
#48629=CARTESIAN_POINT('Ctrl Pts',(7.21828976823775,9.52934075289251,-37.817447696476));
#48630=CARTESIAN_POINT('Ctrl Pts',(7.3467116336193,9.50833437573421,-37.8226219766341));
#48631=CARTESIAN_POINT('Ctrl Pts',(7.61952278444273,9.46057626186425,-37.8348434394394));
#48632=CARTESIAN_POINT('Ctrl Pts',(7.960209967387,9.39369388800056,-37.8525768539309));
#48633=CARTESIAN_POINT('Ctrl Pts',(8.3778920674049,9.29718580374087,-37.8781705824178));
#48634=CARTESIAN_POINT('Ctrl Pts',(8.93892669180996,9.14269283098213,-37.9179631531491));
#48635=CARTESIAN_POINT('Ctrl Pts',(9.64584227564656,8.89230767815167,-37.9785191856093));
#48636=CARTESIAN_POINT('Ctrl Pts',(10.2035290263583,8.61151321278556,-38.0385832751922));
#48637=CARTESIAN_POINT('Ctrl Pts',(11.4269246328553,7.86934876020126,-38.1861224416156));
#48638=CARTESIAN_POINT('Ctrl Pts',(12.3794141170359,6.89524642147764,-38.3965674938924));
#48639=CARTESIAN_POINT('Ctrl Pts',(13.2972381141874,5.79878047753586,-38.5654665629587));
#48640=CARTESIAN_POINT('Ctrl Pts',(13.5062083794909,5.54140336948116,-38.6011993448011));
#48641=CARTESIAN_POINT('Ctrl Pts',(13.6094812333749,5.41297301418053,-38.61791765796));
#48642=CARTESIAN_POINT('Ctrl Pts',(13.6681544593943,5.33961012006986,-38.627141819842));
#48643=CARTESIAN_POINT('Ctrl Pts',(13.6973468401446,5.30300492151899,-38.6316312237005));
#48644=CARTESIAN_POINT('Ctrl Pts',(13.9814496921678,4.94616478641267,-38.6748449459509));
#48645=CARTESIAN_POINT('Ctrl Pts',(14.5280778199499,4.18885241132974,-38.7627420404612));
#48646=CARTESIAN_POINT('Ctrl Pts',(15.0243070371674,3.39004417986617,-38.8395722021707));
#48647=CARTESIAN_POINT('Ctrl Pts',(15.2656150130537,2.98140716137769,-38.873032388801));
#48648=CARTESIAN_POINT('',(3.2,9.24182505978396,-36.4465179346992));
#48649=CARTESIAN_POINT('Ctrl Pts',(3.19846192322169,9.24174412230254,-36.446524619893));
#48650=CARTESIAN_POINT('Ctrl Pts',(3.06435645359065,9.3115682491172,-36.7523808556989));
#48651=CARTESIAN_POINT('Ctrl Pts',(2.93025382215074,9.38137979123532,-37.0581800253732));
#48652=CARTESIAN_POINT('Ctrl Pts',(2.79625939386437,9.4511090207012,-37.3636263694961));
#48653=CARTESIAN_POINT('',(15.,1.76250180637585,-15.7004962848173));
#48654=CARTESIAN_POINT('Ctrl Pts',(15.,1.76250180637585,-15.7004962848173));
#48655=CARTESIAN_POINT('Ctrl Pts',(14.489716577951,2.14749161156547,-16.2136060493571));
#48656=CARTESIAN_POINT('Ctrl Pts',(13.9833803026603,2.52923395303641,-16.7499747962178));
#48657=CARTESIAN_POINT('Ctrl Pts',(13.4460287676664,2.91284724496658,-17.3603709065187));
#48658=CARTESIAN_POINT('Ctrl Pts',(12.8282655680968,3.3538661296022,-18.0621093952879));
#48659=CARTESIAN_POINT('Ctrl Pts',(12.1555414089315,3.86577076245241,-18.8782945384456));
#48660=CARTESIAN_POINT('Ctrl Pts',(11.590490807333,4.2779947817326,-19.615690057469));
#48661=CARTESIAN_POINT('Ctrl Pts',(11.1143368259492,4.62536563214324,-20.2370747816766));
#48662=CARTESIAN_POINT('Ctrl Pts',(10.695315894954,4.91856680462629,-20.8194972243441));
#48663=CARTESIAN_POINT('Ctrl Pts',(10.2957959918397,5.1785107966465,-21.4059609250791));
#48664=CARTESIAN_POINT('Ctrl Pts',(10.0450888109769,5.34163114412759,-21.7739792889792));
#48665=CARTESIAN_POINT('Ctrl Pts',(9.80235305588442,5.49247002263581,-22.1433667549693));
#48666=CARTESIAN_POINT('Ctrl Pts',(9.56010106243628,5.63900849396958,-22.5247929586984));
#48667=CARTESIAN_POINT('Ctrl Pts',(9.36613602954693,5.75633813492419,-22.8301912553154));
#48668=CARTESIAN_POINT('Ctrl Pts',(9.15248571318201,5.88298942934388,-23.173697229624));
#48669=CARTESIAN_POINT('Ctrl Pts',(8.89022359857544,6.03502754169084,-23.6134759700354));
#48670=CARTESIAN_POINT('Ctrl Pts',(8.39222406134029,6.32372692057166,-24.4485550646247));
#48671=CARTESIAN_POINT('Ctrl Pts',(7.76643777388907,6.67223453859443,-25.5605956387439));
#48672=CARTESIAN_POINT('Ctrl Pts',(7.10363554123529,7.0511614476926,-26.8754977862185));
#48673=CARTESIAN_POINT('Ctrl Pts',(6.2355001824917,7.5474781949211,-28.59775065634));
#48674=CARTESIAN_POINT('Ctrl Pts',(5.31040885823697,7.96875536932003,-30.6993155625113));
#48675=CARTESIAN_POINT('Ctrl Pts',(4.4641661690584,8.44366203772272,-32.909077030235));
#48676=CARTESIAN_POINT('Ctrl Pts',(4.30741751125468,8.53162850857804,-33.318388860708));
#48677=CARTESIAN_POINT('Ctrl Pts',(4.15262292089523,8.62235919623212,-33.732460653513));
#48678=CARTESIAN_POINT('Ctrl Pts',(4.,8.71775829923914,-34.1504314334527));
#48679=CARTESIAN_POINT('Ctrl Pts',(3.72434973283382,8.89005737513843,-34.9053230085993));
#48680=CARTESIAN_POINT('Ctrl Pts',(3.45587123478818,9.06598205759024,-35.6760994039458));
#48681=CARTESIAN_POINT('Ctrl Pts',(3.2,9.24182505978395,-36.4465179346992));
#48682=CARTESIAN_POINT('',(15.,2.79596292475043,-30.471996838465));
#48683=CARTESIAN_POINT('Ctrl Pts',(15.,2.79596292475043,-30.471996838465));
#48684=CARTESIAN_POINT('Ctrl Pts',(15.,2.47177016953902,-26.0694692115998));
#48685=CARTESIAN_POINT('Ctrl Pts',(15.,2.09636968496858,-20.8427222796618));
#48686=CARTESIAN_POINT('Ctrl Pts',(15.,1.76250180637585,-15.7004962848173));
#48687=CARTESIAN_POINT('Ctrl Pts',(6.,9.62277221548328,-37.7942092772018));
#48688=CARTESIAN_POINT('Ctrl Pts',(6.38595465246567,9.50256245865601,-37.2711033988583));
#48689=CARTESIAN_POINT('Ctrl Pts',(6.7702364866826,9.36752460422606,-36.7864270136994));
#48690=CARTESIAN_POINT('Ctrl Pts',(7.13915213286207,9.20934876194912,-36.3528657054113));
#48691=CARTESIAN_POINT('Ctrl Pts',(8.10667920093232,8.79451298444103,-35.2157973653154));
#48692=CARTESIAN_POINT('Ctrl Pts',(8.9801988874736,8.36872065597838,-34.3895418272531));
#48693=CARTESIAN_POINT('Ctrl Pts',(9.46656009721066,8.09341256870629,-33.9615794459728));
#48694=CARTESIAN_POINT('Ctrl Pts',(9.65648624874906,7.98590357239622,-33.7944582889962));
#48695=CARTESIAN_POINT('Ctrl Pts',(9.79228848853725,7.90448352099192,-33.6801480890427));
#48696=CARTESIAN_POINT('Ctrl Pts',(9.94593825727815,7.80836128617838,-33.5541469568644));
#48697=CARTESIAN_POINT('Ctrl Pts',(10.1065740866009,7.70786862008357,-33.4224168766375));
#48698=CARTESIAN_POINT('Ctrl Pts',(10.2660951669675,7.60273427161563,-33.2963654618293));
#48699=CARTESIAN_POINT('Ctrl Pts',(10.4261869573617,7.4903924666703,-33.1745211766193));
#48700=CARTESIAN_POINT('Ctrl Pts',(10.8065549509411,7.2234754259092,-32.8850268422731));
#48701=CARTESIAN_POINT('Ctrl Pts',(11.1894211925257,6.91488309382193,-32.619770871127));
#48702=CARTESIAN_POINT('Ctrl Pts',(11.6023503255242,6.54089716906719,-32.3560535901122));
#48703=CARTESIAN_POINT('Ctrl Pts',(11.7531893954247,6.40428368133321,-32.2597201851618));
#48704=CARTESIAN_POINT('Ctrl Pts',(11.9080270687775,6.25882196066766,-32.1636787693489));
#48705=CARTESIAN_POINT('Ctrl Pts',(12.0681766131679,6.1031541062351,-32.0669994274948));
#48706=CARTESIAN_POINT('Ctrl Pts',(12.1838435903474,5.99072400076856,-31.9971733953913));
#48707=CARTESIAN_POINT('Ctrl Pts',(12.310086541016,5.86655265076557,-31.9217320004455));
#48708=CARTESIAN_POINT('Ctrl Pts',(12.5127093730711,5.65894503108766,-31.8047262190236));
#48709=CARTESIAN_POINT('Ctrl Pts',(12.7975492664041,5.36709770250972,-31.6402436976734));
#48710=CARTESIAN_POINT('Ctrl Pts',(13.1874566943566,4.95016249777334,-31.4228609771219));
#48711=CARTESIAN_POINT('Ctrl Pts',(13.6431584568239,4.45104726343863,-31.1770289723232));
#48712=CARTESIAN_POINT('Ctrl Pts',(14.069523646534,3.98406341763974,-30.9470228191864));
#48713=CARTESIAN_POINT('Ctrl Pts',(14.53311408767,3.41883288085212,-30.7098459010755));
#48714=CARTESIAN_POINT('Ctrl Pts',(15.,2.79596292475043,-30.471996838465));
#48715=CARTESIAN_POINT('Origin',(15.,-1.89142793862867,-8.2868872535455));
#48716=CARTESIAN_POINT('',(15.,-0.464917847313567,-15.7922717682507));
#48717=CARTESIAN_POINT('Ctrl Pts',(15.,-0.464917847313565,-15.7922717682507));
#48718=CARTESIAN_POINT('Ctrl Pts',(15.,0.278045388530768,-15.8141442938323));
#48719=CARTESIAN_POINT('Ctrl Pts',(15.,1.02237787096417,-15.7835809051657));
#48720=CARTESIAN_POINT('Ctrl Pts',(15.,1.76250180637586,-15.7004962848173));
#48721=CARTESIAN_POINT('',(15.,-0.316722183622946,-30.5983608557452));
#48722=CARTESIAN_POINT('Ctrl Pts',(15.,-0.464917847313579,-15.7922717682507));
#48723=CARTESIAN_POINT('Ctrl Pts',(15.,-0.381235181719544,-21.0899243277258));
#48724=CARTESIAN_POINT('Ctrl Pts',(15.,-0.341535500947833,-26.4322224392563));
#48725=CARTESIAN_POINT('Ctrl Pts',(15.,-0.316722183622933,-30.5983608557452));
#48726=CARTESIAN_POINT('Origin',(15.,0.,0.));
#48727=CARTESIAN_POINT('Ctrl Pts',(15.,-6.80914057906323,-29.8327941127638));
#48728=CARTESIAN_POINT('Ctrl Pts',(15.,23.0236535337006,-36.641934691827));
#48729=CARTESIAN_POINT('Ctrl Pts',(15.,29.8327941127638,-6.80914057906323));
#48730=CARTESIAN_POINT('Ctrl Pts',(15.,36.641934691827,23.0236535337006));
#48731=CARTESIAN_POINT('Ctrl Pts',(15.,6.80914057906323,29.8327941127638));
#48732=CARTESIAN_POINT('Ctrl Pts',(15.,-23.0236535337006,36.641934691827));
#48733=CARTESIAN_POINT('Ctrl Pts',(15.,-29.8327941127638,6.80914057906323));
#48734=CARTESIAN_POINT('Ctrl Pts',(15.,-36.641934691827,-23.0236535337006));
#48735=CARTESIAN_POINT('Ctrl Pts',(15.,-6.80914057906323,-29.8327941127638));
#48736=CARTESIAN_POINT('Ctrl Pts',(14.7843073131059,-6.83933995053714,-29.9651062042906));
#48737=CARTESIAN_POINT('Ctrl Pts',(14.7843073131059,23.1257662537535,-36.8044461548278));
#48738=CARTESIAN_POINT('Ctrl Pts',(14.7843073131059,29.9651062042906,-6.83933995053714));
#48739=CARTESIAN_POINT('Ctrl Pts',(14.7843073131059,36.8044461548278,23.1257662537535));
#48740=CARTESIAN_POINT('Ctrl Pts',(14.7843073131059,6.83933995053714,29.9651062042906));
#48741=CARTESIAN_POINT('Ctrl Pts',(14.7843073131059,-23.1257662537535,36.8044461548278));
#48742=CARTESIAN_POINT('Ctrl Pts',(14.7843073131059,-29.9651062042906,6.83933995053714));
#48743=CARTESIAN_POINT('Ctrl Pts',(14.7843073131059,-36.8044461548278,-23.1257662537535));
#48744=CARTESIAN_POINT('Ctrl Pts',(14.7843073131059,-6.83933995053714,-29.9651062042906));
#48745=CARTESIAN_POINT('Ctrl Pts',(14.3560298066371,-6.90036423817606,-30.2324710777091));
#48746=CARTESIAN_POINT('Ctrl Pts',(14.3560298066371,23.3321068395331,-37.1328353158852));
#48747=CARTESIAN_POINT('Ctrl Pts',(14.3560298066371,30.2324710777091,-6.90036423817606));
#48748=CARTESIAN_POINT('Ctrl Pts',(14.3560298066371,37.1328353158852,23.3321068395331));
#48749=CARTESIAN_POINT('Ctrl Pts',(14.3560298066371,6.90036423817606,30.2324710777091));
#48750=CARTESIAN_POINT('Ctrl Pts',(14.3560298066371,-23.3321068395331,37.1328353158852));
#48751=CARTESIAN_POINT('Ctrl Pts',(14.3560298066371,-30.2324710777091,6.90036423817606));
#48752=CARTESIAN_POINT('Ctrl Pts',(14.3560298066371,-37.1328353158852,-23.3321068395331));
#48753=CARTESIAN_POINT('Ctrl Pts',(14.3560298066371,-6.90036423817606,-30.2324710777091));
#48754=CARTESIAN_POINT('Ctrl Pts',(13.722936818686,-6.99377723724461,-30.6417401677374));
#48755=CARTESIAN_POINT('Ctrl Pts',(13.722936818686,23.6479629304928,-37.635517404982));
#48756=CARTESIAN_POINT('Ctrl Pts',(13.722936818686,30.6417401677374,-6.99377723724461));
#48757=CARTESIAN_POINT('Ctrl Pts',(13.722936818686,37.635517404982,23.6479629304928));
#48758=CARTESIAN_POINT('Ctrl Pts',(13.722936818686,6.99377723724461,30.6417401677374));
#48759=CARTESIAN_POINT('Ctrl Pts',(13.722936818686,-23.6479629304928,37.635517404982));
#48760=CARTESIAN_POINT('Ctrl Pts',(13.722936818686,-30.6417401677374,6.99377723724461));
#48761=CARTESIAN_POINT('Ctrl Pts',(13.722936818686,-37.635517404982,-23.6479629304928));
#48762=CARTESIAN_POINT('Ctrl Pts',(13.722936818686,-6.99377723724461,-30.6417401677374));
#48763=CARTESIAN_POINT('Ctrl Pts',(12.8977690042853,-7.12214335873524,-31.204148893041));
#48764=CARTESIAN_POINT('Ctrl Pts',(12.8977690042853,24.0820055343058,-38.3262922517763));
#48765=CARTESIAN_POINT('Ctrl Pts',(12.8977690042853,31.204148893041,-7.12214335873524));
#48766=CARTESIAN_POINT('Ctrl Pts',(12.8977690042853,38.3262922517763,24.0820055343058));
#48767=CARTESIAN_POINT('Ctrl Pts',(12.8977690042853,7.12214335873524,31.204148893041));
#48768=CARTESIAN_POINT('Ctrl Pts',(12.8977690042853,-24.0820055343058,38.3262922517763));
#48769=CARTESIAN_POINT('Ctrl Pts',(12.8977690042853,-31.204148893041,7.12214335873524));
#48770=CARTESIAN_POINT('Ctrl Pts',(12.8977690042853,-38.3262922517763,-24.0820055343058));
#48771=CARTESIAN_POINT('Ctrl Pts',(12.8977690042853,-7.12214335873524,-31.204148893041));
#48772=CARTESIAN_POINT('Ctrl Pts',(11.9000549946031,-7.28939328253151,-31.9369186874159));
#48773=CARTESIAN_POINT('Ctrl Pts',(11.9000549946031,24.6475254048843,-39.2263119699474));
#48774=CARTESIAN_POINT('Ctrl Pts',(11.9000549946031,31.9369186874159,-7.28939328253151));
#48775=CARTESIAN_POINT('Ctrl Pts',(11.9000549946031,39.2263119699474,24.6475254048843));
#48776=CARTESIAN_POINT('Ctrl Pts',(11.9000549946031,7.28939328253151,31.9369186874159));
#48777=CARTESIAN_POINT('Ctrl Pts',(11.9000549946031,-24.6475254048843,39.2263119699474));
#48778=CARTESIAN_POINT('Ctrl Pts',(11.9000549946031,-31.9369186874159,7.28939328253151));
#48779=CARTESIAN_POINT('Ctrl Pts',(11.9000549946031,-39.2263119699474,-24.6475254048843));
#48780=CARTESIAN_POINT('Ctrl Pts',(11.9000549946031,-7.28939328253151,-31.9369186874159));
#48781=CARTESIAN_POINT('Ctrl Pts',(10.9391333834985,-7.4640486993045,-32.702134066474));
#48782=CARTESIAN_POINT('Ctrl Pts',(10.9391333834985,25.2380853671694,-40.1661827657784));
#48783=CARTESIAN_POINT('Ctrl Pts',(10.9391333834985,32.702134066474,-7.4640486993045));
#48784=CARTESIAN_POINT('Ctrl Pts',(10.9391333834985,40.1661827657784,25.2380853671694));
#48785=CARTESIAN_POINT('Ctrl Pts',(10.9391333834985,7.4640486993045,32.702134066474));
#48786=CARTESIAN_POINT('Ctrl Pts',(10.9391333834985,-25.2380853671694,40.1661827657784));
#48787=CARTESIAN_POINT('Ctrl Pts',(10.9391333834985,-32.702134066474,7.4640486993045));
#48788=CARTESIAN_POINT('Ctrl Pts',(10.9391333834985,-40.1661827657784,-25.2380853671694));
#48789=CARTESIAN_POINT('Ctrl Pts',(10.9391333834985,-7.4640486993045,-32.702134066474));
#48790=CARTESIAN_POINT('Ctrl Pts',(10.0180552497783,-7.64672372347923,-33.5024856413123));
#48791=CARTESIAN_POINT('Ctrl Pts',(10.0180552497783,25.855761917833,-41.1492093647915));
#48792=CARTESIAN_POINT('Ctrl Pts',(10.0180552497783,33.5024856413123,-7.64672372347923));
#48793=CARTESIAN_POINT('Ctrl Pts',(10.0180552497783,41.1492093647915,25.855761917833));
#48794=CARTESIAN_POINT('Ctrl Pts',(10.0180552497783,7.64672372347923,33.5024856413123));
#48795=CARTESIAN_POINT('Ctrl Pts',(10.0180552497783,-25.855761917833,41.1492093647915));
#48796=CARTESIAN_POINT('Ctrl Pts',(10.0180552497783,-33.5024856413123,7.64672372347923));
#48797=CARTESIAN_POINT('Ctrl Pts',(10.0180552497783,-41.1492093647915,-25.855761917833));
#48798=CARTESIAN_POINT('Ctrl Pts',(10.0180552497783,-7.64672372347923,-33.5024856413123));
#48799=CARTESIAN_POINT('Ctrl Pts',(9.13857394886632,-7.83777126657544,-34.339519618326));
#48800=CARTESIAN_POINT('Ctrl Pts',(9.13857394886632,26.5017483517505,-42.1772908849014));
#48801=CARTESIAN_POINT('Ctrl Pts',(9.13857394886632,34.339519618326,-7.83777126657544));
#48802=CARTESIAN_POINT('Ctrl Pts',(9.13857394886632,42.1772908849014,26.5017483517505));
#48803=CARTESIAN_POINT('Ctrl Pts',(9.13857394886632,7.83777126657544,34.339519618326));
#48804=CARTESIAN_POINT('Ctrl Pts',(9.13857394886632,-26.5017483517505,42.1772908849014));
#48805=CARTESIAN_POINT('Ctrl Pts',(9.13857394886632,-34.339519618326,7.83777126657544));
#48806=CARTESIAN_POINT('Ctrl Pts',(9.13857394886632,-42.1772908849014,-26.5017483517505));
#48807=CARTESIAN_POINT('Ctrl Pts',(9.13857394886632,-7.83777126657544,-34.339519618326));
#48808=CARTESIAN_POINT('Ctrl Pts',(8.29915429043693,-8.03688232886512,-35.21188218125));
#48809=CARTESIAN_POINT('Ctrl Pts',(8.29915429043693,27.1749998523849,-43.2487645101151));
#48810=CARTESIAN_POINT('Ctrl Pts',(8.29915429043693,35.21188218125,-8.03688232886512));
#48811=CARTESIAN_POINT('Ctrl Pts',(8.29915429043693,43.2487645101151,27.1749998523849));
#48812=CARTESIAN_POINT('Ctrl Pts',(8.29915429043693,8.03688232886512,35.21188218125));
#48813=CARTESIAN_POINT('Ctrl Pts',(8.29915429043693,-27.1749998523849,43.2487645101151));
#48814=CARTESIAN_POINT('Ctrl Pts',(8.29915429043693,-35.21188218125,8.03688232886512));
#48815=CARTESIAN_POINT('Ctrl Pts',(8.29915429043693,-43.2487645101151,-27.1749998523849));
#48816=CARTESIAN_POINT('Ctrl Pts',(8.29915429043693,-8.03688232886512,-35.21188218125));
#48817=CARTESIAN_POINT('Ctrl Pts',(7.4968190344241,-8.24345765802359,-36.1169478341035));
#48818=CARTESIAN_POINT('Ctrl Pts',(7.4968190344241,27.8734901760799,-44.3604054921271));
#48819=CARTESIAN_POINT('Ctrl Pts',(7.4968190344241,36.1169478341035,-8.24345765802359));
#48820=CARTESIAN_POINT('Ctrl Pts',(7.4968190344241,44.3604054921271,27.8734901760799));
#48821=CARTESIAN_POINT('Ctrl Pts',(7.4968190344241,8.24345765802359,36.1169478341035));
#48822=CARTESIAN_POINT('Ctrl Pts',(7.4968190344241,-27.8734901760799,44.3604054921271));
#48823=CARTESIAN_POINT('Ctrl Pts',(7.4968190344241,-36.1169478341035,8.24345765802359));
#48824=CARTESIAN_POINT('Ctrl Pts',(7.4968190344241,-44.3604054921271,-27.8734901760799));
#48825=CARTESIAN_POINT('Ctrl Pts',(7.4968190344241,-8.24345765802359,-36.1169478341035));
#48826=CARTESIAN_POINT('Ctrl Pts',(6.88220761950379,-8.41420410800809,-36.8650369106509));
#48827=CARTESIAN_POINT('Ctrl Pts',(6.88220761950379,28.4508328026428,-45.279241018659));
#48828=CARTESIAN_POINT('Ctrl Pts',(6.88220761950379,36.8650369106509,-8.41420410800809));
#48829=CARTESIAN_POINT('Ctrl Pts',(6.88220761950379,45.279241018659,28.4508328026428));
#48830=CARTESIAN_POINT('Ctrl Pts',(6.88220761950379,8.41420410800809,36.8650369106509));
#48831=CARTESIAN_POINT('Ctrl Pts',(6.88220761950379,-28.4508328026428,45.279241018659));
#48832=CARTESIAN_POINT('Ctrl Pts',(6.88220761950379,-36.8650369106509,8.41420410800809));
#48833=CARTESIAN_POINT('Ctrl Pts',(6.88220761950379,-45.279241018659,-28.4508328026428));
#48834=CARTESIAN_POINT('Ctrl Pts',(6.88220761950379,-8.41420410800809,-36.8650369106509));
#48835=CARTESIAN_POINT('Ctrl Pts',(6.43560997955544,-8.54515448010586,-37.4387679776515));
#48836=CARTESIAN_POINT('Ctrl Pts',(6.43560997955544,28.8936134975456,-45.9839224577573));
#48837=CARTESIAN_POINT('Ctrl Pts',(6.43560997955544,37.4387679776515,-8.54515448010586));
#48838=CARTESIAN_POINT('Ctrl Pts',(6.43560997955544,45.9839224577573,28.8936134975456));
#48839=CARTESIAN_POINT('Ctrl Pts',(6.43560997955544,8.54515448010586,37.4387679776515));
#48840=CARTESIAN_POINT('Ctrl Pts',(6.43560997955544,-28.8936134975456,45.9839224577573));
#48841=CARTESIAN_POINT('Ctrl Pts',(6.43560997955544,-37.4387679776515,8.54515448010586));
#48842=CARTESIAN_POINT('Ctrl Pts',(6.43560997955544,-45.9839224577573,-28.8936134975456));
#48843=CARTESIAN_POINT('Ctrl Pts',(6.43560997955544,-8.54515448010586,-37.4387679776515));
#48844=CARTESIAN_POINT('Ctrl Pts',(6.14415685965718,-8.63371847902027,-37.8267922098931));
#48845=CARTESIAN_POINT('Ctrl Pts',(6.14415685965718,29.1930737308728,-46.4605106889134));
#48846=CARTESIAN_POINT('Ctrl Pts',(6.14415685965718,37.8267922098931,-8.63371847902027));
#48847=CARTESIAN_POINT('Ctrl Pts',(6.14415685965718,46.4605106889134,29.1930737308728));
#48848=CARTESIAN_POINT('Ctrl Pts',(6.14415685965718,8.63371847902027,37.8267922098931));
#48849=CARTESIAN_POINT('Ctrl Pts',(6.14415685965718,-29.1930737308728,46.4605106889134));
#48850=CARTESIAN_POINT('Ctrl Pts',(6.14415685965718,-37.8267922098931,8.63371847902027));
#48851=CARTESIAN_POINT('Ctrl Pts',(6.14415685965718,-46.4605106889134,-29.1930737308728));
#48852=CARTESIAN_POINT('Ctrl Pts',(6.14415685965718,-8.63371847902027,-37.8267922098931));
#48853=CARTESIAN_POINT('Ctrl Pts',(6.,-8.67831642429627,-38.0221885750911));
#48854=CARTESIAN_POINT('Ctrl Pts',(6.,29.3438721507948,-46.7005049993874));
#48855=CARTESIAN_POINT('Ctrl Pts',(6.,38.0221885750911,-8.67831642429627));
#48856=CARTESIAN_POINT('Ctrl Pts',(6.,46.7005049993874,29.3438721507948));
#48857=CARTESIAN_POINT('Ctrl Pts',(6.,8.67831642429627,38.0221885750911));
#48858=CARTESIAN_POINT('Ctrl Pts',(6.,-29.3438721507948,46.7005049993874));
#48859=CARTESIAN_POINT('Ctrl Pts',(6.,-38.0221885750911,8.67831642429627));
#48860=CARTESIAN_POINT('Ctrl Pts',(6.,-46.7005049993874,-29.3438721507948));
#48861=CARTESIAN_POINT('Ctrl Pts',(6.,-8.67831642429627,-38.0221885750911));
#48862=CARTESIAN_POINT('Ctrl Pts',(15.,-0.316722183622945,-30.5983608557452));
#48863=CARTESIAN_POINT('Ctrl Pts',(14.0108432136945,1.17201709431794,-31.2361856660366));
#48864=CARTESIAN_POINT('Ctrl Pts',(13.3692319443824,2.16115069187936,-31.5994041040738));
#48865=CARTESIAN_POINT('Ctrl Pts',(12.3476991724842,3.32436243166655,-32.2576222115046));
#48866=CARTESIAN_POINT('Ctrl Pts',(12.0250187050191,3.69179627058093,-32.4655393067194));
#48867=CARTESIAN_POINT('Ctrl Pts',(11.666631757071,4.09680627482432,-32.7013288419197));
#48868=CARTESIAN_POINT('Ctrl Pts',(11.3593868751765,4.42827966965007,-32.911754584138));
#48869=CARTESIAN_POINT('Ctrl Pts',(10.6767716809131,5.16472407974724,-33.3792637840199));
#48870=CARTESIAN_POINT('Ctrl Pts',(10.1321636914396,5.683315063631,-33.7885713862255));
#48871=CARTESIAN_POINT('Ctrl Pts',(9.56604173138329,6.09942379383306,-34.2764646325745));
#48872=CARTESIAN_POINT('Ctrl Pts',(9.34563078589186,6.26142937765097,-34.466418422242));
#48873=CARTESIAN_POINT('Ctrl Pts',(9.12222951098693,6.4073806230979,-34.6687019818405));
#48874=CARTESIAN_POINT('Ctrl Pts',(8.88860711505275,6.54710572768653,-34.8913321958227));
#48875=CARTESIAN_POINT('Ctrl Pts',(8.7583060070074,6.62503633822089,-35.0155024982899));
#48876=CARTESIAN_POINT('Ctrl Pts',(8.62340343546547,6.70326098334285,-35.1456753402879));
#48877=CARTESIAN_POINT('Ctrl Pts',(8.40819516300417,6.81827896718242,-35.3643373125436));
#48878=CARTESIAN_POINT('Ctrl Pts',(8.02443006829128,7.02338208407037,-35.7542611362568));
#48879=CARTESIAN_POINT('Ctrl Pts',(7.46417034513341,7.28861046704501,-36.3577202537473));
#48880=CARTESIAN_POINT('Ctrl Pts',(6.85957019142019,7.5542785284151,-37.0924815402584));
#48881=CARTESIAN_POINT('Ctrl Pts',(6.58024553736739,7.67701690166778,-37.4319405048412));
#48882=CARTESIAN_POINT('Ctrl Pts',(6.28976782192773,7.7784192013204,-37.8052266187655));
#48883=CARTESIAN_POINT('Ctrl Pts',(6.,7.86863926112478,-38.1979648172293));
#48884=CARTESIAN_POINT('Ctrl Pts',(2.1,2.63423723994462,-15.5859107314896));
#48885=CARTESIAN_POINT('Ctrl Pts',(2.73333333333333,2.63423723994462,-15.5859107314896));
#48886=CARTESIAN_POINT('Ctrl Pts',(3.36803664008728,2.63428404646612,-15.585905949688));
#48887=CARTESIAN_POINT('Ctrl Pts',(4.25277473174135,2.63431300446758,-15.5859022596434));
#48888=CARTESIAN_POINT('Ctrl Pts',(4.7726738795535,2.64263459137918,-15.5845888383648));
#48889=CARTESIAN_POINT('Ctrl Pts',(5.76857447316278,2.66677604587533,-15.580829813117));
#48890=CARTESIAN_POINT('Ctrl Pts',(6.48509167696866,2.66613640606125,-15.5809838465372));
#48891=CARTESIAN_POINT('Ctrl Pts',(6.9986700738739,2.63261167807611,-15.5860120825425));
#48892=CARTESIAN_POINT('Ctrl Pts',(7.1248093702523,2.62413102225182,-15.5873970293984));
#48893=CARTESIAN_POINT('Ctrl Pts',(7.37171220185442,2.60630004336253,-15.5904834561901));
#48894=CARTESIAN_POINT('Ctrl Pts',(7.68212025671799,2.5813014534473,-15.5950682446648));
#48895=CARTESIAN_POINT('Ctrl Pts',(8.05074791674676,2.54617937678925,-15.6015350227393));
#48896=CARTESIAN_POINT('Ctrl Pts',(8.41504712921457,2.50497981155993,-15.6088256864165));
#48897=CARTESIAN_POINT('Ctrl Pts',(9.01075531436909,2.42452722421788,-15.622106164644));
#48898=CARTESIAN_POINT('Ctrl Pts',(9.46310495354993,2.33948796976415,-15.6340319240204));
#48899=CARTESIAN_POINT('Ctrl Pts',(10.2678550072569,2.13947451544829,-15.6566084350139));
#48900=CARTESIAN_POINT('Ctrl Pts',(10.980498717346,1.88789553199322,-15.6910504310237));
#48901=CARTESIAN_POINT('Ctrl Pts',(11.7910302128019,1.5198808624596,-15.7315745004185));
#48902=CARTESIAN_POINT('Ctrl Pts',(12.2471583707382,1.29675740685952,-15.7507502462899));
#48903=CARTESIAN_POINT('Ctrl Pts',(12.4732540168102,1.18219132952897,-15.7583530081557));
#48904=CARTESIAN_POINT('Ctrl Pts',(12.8351236964231,0.996750434719523,-15.7683824294791));
#48905=CARTESIAN_POINT('Ctrl Pts',(13.2802523722939,0.745571188508633,-15.7800984771434));
#48906=CARTESIAN_POINT('Ctrl Pts',(14.1612572117153,0.174593511812138,-15.8002843726132));
#48907=CARTESIAN_POINT('Ctrl Pts',(14.7820737708942,-0.295409261491528,
-15.8007188001297));
#48908=CARTESIAN_POINT('Ctrl Pts',(15.1979896574214,-0.617575400326164,
-15.7866563619325));
#48909=CARTESIAN_POINT('Ctrl Pts',(2.1,4.35569033805583,-23.1280895504496));
#48910=CARTESIAN_POINT('Ctrl Pts',(2.73333333333333,4.35569033805583,-23.1280895504496));
#48911=CARTESIAN_POINT('Ctrl Pts',(3.36872398898381,4.35569062738043,-23.1280874009591));
#48912=CARTESIAN_POINT('Ctrl Pts',(4.25416142982039,4.35570368657663,-23.1280836455188));
#48913=CARTESIAN_POINT('Ctrl Pts',(4.78310679221752,4.36813194564395,-23.125880538704));
#48914=CARTESIAN_POINT('Ctrl Pts',(5.77494665368391,4.4039188556977,-23.1196210211601));
#48915=CARTESIAN_POINT('Ctrl Pts',(6.47498050632645,4.40250321929782,-23.1199364094633));
#48916=CARTESIAN_POINT('Ctrl Pts',(6.96728299632452,4.354093744434,-23.1281247524928));
#48917=CARTESIAN_POINT('Ctrl Pts',(7.09310098340823,4.34153119782086,-23.1304190629282));
#48918=CARTESIAN_POINT('Ctrl Pts',(7.33630050458593,4.31533084892448,-23.1354690138891));
#48919=CARTESIAN_POINT('Ctrl Pts',(7.64237623855619,4.27855698732002,-23.1429403183708));
#48920=CARTESIAN_POINT('Ctrl Pts',(8.00393172538093,4.22710168295328,-23.1534475126223));
#48921=CARTESIAN_POINT('Ctrl Pts',(8.36002498314573,4.1668247936586,-23.1653185047848));
#48922=CARTESIAN_POINT('Ctrl Pts',(8.93969209567688,4.04959492469466,-23.1870206770975));
#48923=CARTESIAN_POINT('Ctrl Pts',(9.37530731609186,3.92607810867588,-23.206753996033));
#48924=CARTESIAN_POINT('Ctrl Pts',(10.1434138046995,3.63794852015698,-23.2448736971823));
#48925=CARTESIAN_POINT('Ctrl Pts',(10.8343054438102,3.27311237366711,-23.302594912175));
#48926=CARTESIAN_POINT('Ctrl Pts',(11.6346922265994,2.73179750623232,-23.3737077261503));
#48927=CARTESIAN_POINT('Ctrl Pts',(12.0872651951508,2.40223791703188,-23.4089168529062));
#48928=CARTESIAN_POINT('Ctrl Pts',(12.3122562294304,2.23255415955555,-23.4236833570785));
#48929=CARTESIAN_POINT('Ctrl Pts',(12.6725938536727,1.95767219781265,-23.4441942800126));
#48930=CARTESIAN_POINT('Ctrl Pts',(13.1110177184242,1.58855368014533,-23.4695074870954));
#48931=CARTESIAN_POINT('Ctrl Pts',(13.9921363954637,0.740833940613477,-23.5179668578115));
#48932=CARTESIAN_POINT('Ctrl Pts',(14.6125773377935,0.0396247240743743,
-23.5335057485051));
#48933=CARTESIAN_POINT('Ctrl Pts',(15.0291266285127,-0.440734376589787,
-23.5225596826963));
#48934=CARTESIAN_POINT('Ctrl Pts',(2.1,6.07714343616704,-30.6702683694095));
#48935=CARTESIAN_POINT('Ctrl Pts',(2.73333333333333,6.07714343616704,-30.6702683694095));
#48936=CARTESIAN_POINT('Ctrl Pts',(3.36945958341804,6.07717722320183,-30.6702656075858));
#48937=CARTESIAN_POINT('Ctrl Pts',(4.25562671182518,6.07721688165371,-30.670259318268));
#48938=CARTESIAN_POINT('Ctrl Pts',(4.79359973395393,6.09396500121367,-30.6671255957162));
#48939=CARTESIAN_POINT('Ctrl Pts',(5.78147401822761,6.14136098671505,-30.6583758536804));
#48940=CARTESIAN_POINT('Ctrl Pts',(6.4648840207481,6.13880226019081,-30.6589606350546));
#48941=CARTESIAN_POINT('Ctrl Pts',(6.93656501913405,6.07755693484608,-30.6698536724228));
#48942=CARTESIAN_POINT('Ctrl Pts',(7.06207690982115,6.06095167183043,-30.6730498747395));
#48943=CARTESIAN_POINT('Ctrl Pts',(7.30170804808245,6.02676597688089,-30.6799788900474));
#48944=CARTESIAN_POINT('Ctrl Pts',(7.60368704328889,5.97877943348734,-30.6902211938605));
#48945=CARTESIAN_POINT('Ctrl Pts',(7.95862439600783,5.9119387988861,-30.7045635161671));
#48946=CARTESIAN_POINT('Ctrl Pts',(8.30733299996974,5.83399140756548,-30.720729237723));
#48947=CARTESIAN_POINT('Ctrl Pts',(8.8731248965081,5.68286843237248,-30.7502492385606));
#48948=CARTESIAN_POINT('Ctrl Pts',(9.29620369485914,5.52518105379277,-30.7769877010294));
#48949=CARTESIAN_POINT('Ctrl Pts',(10.0462911639137,5.15759233537921,-30.8292071711315));
#48950=CARTESIAN_POINT('Ctrl Pts',(10.7405327020582,4.67977587197762,-30.910728379429));
#48951=CARTESIAN_POINT('Ctrl Pts',(11.5482388133752,3.9589695893727,-31.0138279185717));
#48952=CARTESIAN_POINT('Ctrl Pts',(12.0041927687279,3.52013192061582,-31.0656488947084));
#48953=CARTESIAN_POINT('Ctrl Pts',(12.2304250340033,3.29424718610841,-31.0878029021856));
#48954=CARTESIAN_POINT('Ctrl Pts',(12.592462326635,2.92853161577797,-31.1190962862895));
#48955=CARTESIAN_POINT('Ctrl Pts',(13.0427831678653,2.42988806009575,-31.1594573795255));
#48956=CARTESIAN_POINT('Ctrl Pts',(13.9385931776195,1.28678743877928,-31.2371495387447));
#48957=CARTESIAN_POINT('Ctrl Pts',(14.5670688438605,0.345402523233098,-31.2672485558412));
#48958=CARTESIAN_POINT('Ctrl Pts',(14.9853697475044,-0.295704939189027,
-31.2586524717173));
#48959=CARTESIAN_POINT('Ctrl Pts',(2.1,7.79859653427825,-38.2124471883694));
#48960=CARTESIAN_POINT('Ctrl Pts',(2.73333333333333,7.79859653427825,-38.2124471883694));
#48961=CARTESIAN_POINT('Ctrl Pts',(3.37021070699167,7.79865015066291,-38.2124467236009));
#48962=CARTESIAN_POINT('Ctrl Pts',(4.25713136478402,7.79871060554537,-38.2124392001889));
#48963=CARTESIAN_POINT('Ctrl Pts',(4.80403820074332,7.81995661662065,-38.2083337385743));
#48964=CARTESIAN_POINT('Ctrl Pts',(5.78815121291481,7.87887020159365,-38.1971151577803));
#48965=CARTESIAN_POINT('Ctrl Pts',(6.45447266161553,7.87478058883867,-38.1980560957262));
#48966=CARTESIAN_POINT('Ctrl Pts',(6.90692957647958,7.80232226231815,-38.2112861879985));
#48967=CARTESIAN_POINT('Ctrl Pts',(7.032165457778,7.78170112754514,-38.2153789543197));
#48968=CARTESIAN_POINT('Ctrl Pts',(7.26851594405159,7.73982585614224,-38.2241216301496));
#48969=CARTESIAN_POINT('Ctrl Pts',(7.56685490730932,7.6809917809098,-38.2370557901758));
#48970=CARTESIAN_POINT('Ctrl Pts',(7.91607146916962,7.59937001992814,-38.2551036608661));
#48971=CARTESIAN_POINT('Ctrl Pts',(8.25886724527956,7.50440308803594,-38.2754297306033));
#48972=CARTESIAN_POINT('Ctrl Pts',(8.81429346985747,7.32035697382287,-38.3125753180262));
#48973=CARTESIAN_POINT('Ctrl Pts',(9.23055651635836,7.1284382229659,-38.3463705594797));
#48974=CARTESIAN_POINT('Ctrl Pts',(9.97651634618026,6.67420404251485,-38.4141644165199));
#48975=CARTESIAN_POINT('Ctrl Pts',(10.6790339240321,6.07086426145419,-38.5216903207257));
#48976=CARTESIAN_POINT('Ctrl Pts',(11.4920994171454,5.16371480780835,-38.6572666452876));
#48977=CARTESIAN_POINT('Ctrl Pts',(11.9504512124452,4.6129529013925,-38.7257133127446));
#48978=CARTESIAN_POINT('Ctrl Pts',(12.1774804536882,4.33005084296087,-38.7551604165864));
#48979=CARTESIAN_POINT('Ctrl Pts',(12.5406793344479,3.87236046705292,-38.7970589070402));
#48980=CARTESIAN_POINT('Ctrl Pts',(12.997676322199,3.23875815742499,-38.852528788328));
#48981=CARTESIAN_POINT('Ctrl Pts',(13.8994019966035,1.79892708623314,-38.9581992267936));
#48982=CARTESIAN_POINT('Ctrl Pts',(14.5324532885843,0.616949591171014,-39.0018896025419));
#48983=CARTESIAN_POINT('Ctrl Pts',(14.9514110803021,-0.184656989198702,
-38.9949476528204));
#48984=CARTESIAN_POINT('',(3.2,7.48695481785668,-36.8470556158206));
#48985=CARTESIAN_POINT('Ctrl Pts',(3.2,7.48695481785666,-36.8470556158206));
#48986=CARTESIAN_POINT('Ctrl Pts',(3.56152274835393,7.23850467267132,-35.758524406553));
#48987=CARTESIAN_POINT('Ctrl Pts',(3.9522458452532,6.98124869657211,-34.6574817939615));
#48988=CARTESIAN_POINT('Ctrl Pts',(4.78767430123564,6.50176646734495,-32.4570223530551));
#48989=CARTESIAN_POINT('Ctrl Pts',(5.21513946231871,6.28745813065541,-31.4003659031685));
#48990=CARTESIAN_POINT('Ctrl Pts',(6.7954877540227,5.48952449917086,-27.7535421576937));
#48991=CARTESIAN_POINT('Ctrl Pts',(7.94016295938835,4.80756957336196,-25.6343057630554));
#48992=CARTESIAN_POINT('Ctrl Pts',(9.46271935274979,3.88311582182901,-23.0131511987367));
#48993=CARTESIAN_POINT('Ctrl Pts',(10.1385443658991,3.41245828241658,-21.9686504652261));
#48994=CARTESIAN_POINT('Ctrl Pts',(11.5967860400689,2.25751184246001,-19.9258955400566));
#48995=CARTESIAN_POINT('Ctrl Pts',(12.3997356677078,1.62815414544412,-18.8695347898452));
#48996=CARTESIAN_POINT('Ctrl Pts',(13.6850585208118,0.605365893689495,-17.2836977845855));
#48997=CARTESIAN_POINT('Ctrl Pts',(14.3457395898618,0.0481078758601368,
-16.5165260745379));
#48998=CARTESIAN_POINT('Ctrl Pts',(15.,-0.464917847313566,-15.7922717682507));
#48999=CARTESIAN_POINT('Ctrl Pts',(2.79815218354944,7.69629621196739,-37.7641605227833));
#49000=CARTESIAN_POINT('Ctrl Pts',(2.93286301340791,7.62655056963892,-37.4585579619049));
#49001=CARTESIAN_POINT('Ctrl Pts',(3.06773150272457,7.55676145962031,-37.1527603668643));
#49002=CARTESIAN_POINT('Ctrl Pts',(3.20258453830003,7.48699350665232,-36.8470540770711));
#49003=CARTESIAN_POINT('Origin',(2.9,0.,0.));
#49004=CARTESIAN_POINT('',(3.2,-7.48695481785666,-36.8470556158206));
#49005=CARTESIAN_POINT('Origin',(3.2,0.,0.));
#49006=CARTESIAN_POINT('Ctrl Pts',(3.19856230423365,-7.48704093025229,-36.8470163272698));
#49007=CARTESIAN_POINT('Ctrl Pts',(3.0644392731241,-7.55683434047029,-37.1528795715508));
#49008=CARTESIAN_POINT('Ctrl Pts',(2.93031838720717,-7.62661528615582,-37.4586872363272));
#49009=CARTESIAN_POINT('Ctrl Pts',(2.79630735614137,-7.69631837557393,-37.7641425125794));
#49010=CARTESIAN_POINT('Ctrl Pts',(2.1,-9.137400984347,-12.90142634814));
#49011=CARTESIAN_POINT('Ctrl Pts',(2.73333333333333,-9.137400984347,-12.90142634814));
#49012=CARTESIAN_POINT('Ctrl Pts',(3.365973712246,-9.13746504152622,-12.9013637498414));
#49013=CARTESIAN_POINT('Ctrl Pts',(4.12348671872558,-9.13748461543386,-12.9013444788804));
#49014=CARTESIAN_POINT('Ctrl Pts',(4.36308068280113,-9.13590525422836,-12.9024878598794));
#49015=CARTESIAN_POINT('Ctrl Pts',(4.85756687529509,-9.12862669836929,-12.9077725838742));
#49016=CARTESIAN_POINT('Ctrl Pts',(5.73898782434893,-9.11132026423094,-12.9203618153208));
#49017=CARTESIAN_POINT('Ctrl Pts',(6.52605775660734,-9.11084083138628,-12.9207276583753));
#49018=CARTESIAN_POINT('Ctrl Pts',(7.12756933428754,-9.14287723972839,-12.8972432395004));
#49019=CARTESIAN_POINT('Ctrl Pts',(7.25506469988018,-9.14994617799211,-12.8921744658959));
#49020=CARTESIAN_POINT('Ctrl Pts',(7.51732351444062,-9.16567242155789,-12.8811147657457));
#49021=CARTESIAN_POINT('Ctrl Pts',(7.84589135656503,-9.18794199222896,-12.8657492998081));
#49022=CARTESIAN_POINT('Ctrl Pts',(8.24417023302519,-9.21975289392636,-12.8438195891331));
#49023=CARTESIAN_POINT('Ctrl Pts',(8.77647055639935,-9.27004204587853,-12.8086070647954));
#49024=CARTESIAN_POINT('Ctrl Pts',(9.44114142908682,-9.34965285699896,-12.7510329694809));
#49025=CARTESIAN_POINT('Ctrl Pts',(9.96389223057755,-9.43618098671083,-12.6847093516977));
#49026=CARTESIAN_POINT('Ctrl Pts',(11.1189211579548,-9.66280193839667,-12.5054821536567));
#49027=CARTESIAN_POINT('Ctrl Pts',(12.080463293236,-9.98373232849783,-12.2611717068893));
#49028=CARTESIAN_POINT('Ctrl Pts',(13.0008495768038,-10.3265199570838,-11.9667211468366));
#49029=CARTESIAN_POINT('Ctrl Pts',(13.2108260900368,-10.4056770861943,-11.8966961179284));
#49030=CARTESIAN_POINT('Ctrl Pts',(13.3144491940718,-10.4448306117047,-11.8614746909584));
#49031=CARTESIAN_POINT('Ctrl Pts',(13.3733290414177,-10.4670878289521,-11.8412790539105));
#49032=CARTESIAN_POINT('Ctrl Pts',(13.4026082954906,-10.4781554201219,-11.8311771752724));
#49033=CARTESIAN_POINT('Ctrl Pts',(13.6877981560128,-10.5859241331148,-11.732479296786));
#49034=CARTESIAN_POINT('Ctrl Pts',(14.2465882704735,-10.8170217282857,-11.5176433731241));
#49035=CARTESIAN_POINT('Ctrl Pts',(14.7537307590314,-11.056004238249,-11.2866625718643));
#49036=CARTESIAN_POINT('Ctrl Pts',(14.9999999999997,-11.1762403837995,-11.167078717827));
#49037=CARTESIAN_POINT('Ctrl Pts',(2.1,-13.9602886030972,-18.9491361350573));
#49038=CARTESIAN_POINT('Ctrl Pts',(2.73333333333333,-13.9602886030972,-18.9491361350573));
#49039=CARTESIAN_POINT('Ctrl Pts',(3.36558929933722,-13.9603388813315,-18.949091413765));
#49040=CARTESIAN_POINT('Ctrl Pts',(4.12268680117359,-13.9603530925967,-18.9490786756313));
#49041=CARTESIAN_POINT('Ctrl Pts',(4.35700071618798,-13.9580622630443,-18.9508062100769));
#49042=CARTESIAN_POINT('Ctrl Pts',(4.84800506483027,-13.9474262305624,-18.9588441525132));
#49043=CARTESIAN_POINT('Ctrl Pts',(5.73069160467532,-13.9219831875589,-18.9780946562289));
#49044=CARTESIAN_POINT('Ctrl Pts',(6.53595554087845,-13.9209135422454,-18.9789455178027));
#49045=CARTESIAN_POINT('Ctrl Pts',(7.15870948280726,-13.969072695455,-18.9423072738915));
#49046=CARTESIAN_POINT('Ctrl Pts',(7.28653449300648,-13.9794730149236,-18.9345516012843));
#49047=CARTESIAN_POINT('Ctrl Pts',(7.55249858901944,-14.0027853431907,-18.9175010740327));
#49048=CARTESIAN_POINT('Ctrl Pts',(7.8854250805442,-14.0357701876927,-18.893829697599));
#49049=CARTESIAN_POINT('Ctrl Pts',(8.29077969779674,-14.0830375031778,-18.8599241823138));
#49050=CARTESIAN_POINT('Ctrl Pts',(8.83405094145081,-14.1578675644896,-18.805435373411));
#49051=CARTESIAN_POINT('Ctrl Pts',(9.51599654655467,-14.2767190591612,-18.7161020141187));
#49052=CARTESIAN_POINT('Ctrl Pts',(10.0563180414682,-14.4064700137606,-18.6129001575941));
#49053=CARTESIAN_POINT('Ctrl Pts',(11.2545469680855,-14.7474852276745,-18.3333024528578));
#49054=CARTESIAN_POINT('Ctrl Pts',(12.2342109401188,-15.2253867757627,-17.9550408590473));
#49055=CARTESIAN_POINT('Ctrl Pts',(13.160804185079,-15.7295857192779,-17.5044322625813));
#49056=CARTESIAN_POINT('Ctrl Pts',(13.3719043594969,-15.8458680331158,-17.3974114070575));
#49057=CARTESIAN_POINT('Ctrl Pts',(13.4759524598702,-15.903315763404,-17.3436343217885));
#49058=CARTESIAN_POINT('Ctrl Pts',(13.5350561403457,-15.9359605015101,-17.3128100925608));
#49059=CARTESIAN_POINT('Ctrl Pts',(13.5644260429486,-15.9521864940619,-17.2973960592047));
#49060=CARTESIAN_POINT('Ctrl Pts',(13.8509127097168,-16.1101904313627,-17.1468470987892));
#49061=CARTESIAN_POINT('Ctrl Pts',(14.4159152208145,-16.4514462123258,-16.8174302408524));
#49062=CARTESIAN_POINT('Ctrl Pts',(14.9236315787721,-16.8008746420588,-16.4663087459205));
#49063=CARTESIAN_POINT('Ctrl Pts',(15.169681381964,-16.9765158478446,-16.2846381189209));
#49064=CARTESIAN_POINT('Ctrl Pts',(2.1,-18.7831762218474,-24.9968459219746));
#49065=CARTESIAN_POINT('Ctrl Pts',(2.73333333333333,-18.7831762218474,-24.9968459219746));
#49066=CARTESIAN_POINT('Ctrl Pts',(3.3651198397079,-18.7832600991187,-24.9967641409249));
#49067=CARTESIAN_POINT('Ctrl Pts',(4.12177662671699,-18.7832835494852,-24.9967408050916));
#49068=CARTESIAN_POINT('Ctrl Pts',(4.35079814858358,-18.7803301229489,-24.9990120557395));
#49069=CARTESIAN_POINT('Ctrl Pts',(4.83833501195452,-18.7664351600051,-25.0097212931742));
#49070=CARTESIAN_POINT('Ctrl Pts',(5.72217492112382,-18.7328455282091,-25.0356357989273));
#49071=CARTESIAN_POINT('Ctrl Pts',(6.54572526829364,-18.7308544639692,-25.0372090892692));
#49072=CARTESIAN_POINT('Ctrl Pts',(7.189043387547,-18.7967679600979,-24.9861010385379));
#49073=CARTESIAN_POINT('Ctrl Pts',(7.31718157815736,-18.8105293955174,-24.9756330333963));
#49074=CARTESIAN_POINT('Ctrl Pts',(7.58671359051966,-18.84173419862,-24.9523431866193));
#49075=CARTESIAN_POINT('Ctrl Pts',(7.92374496455099,-18.8858694172611,-24.9200041574497));
#49076=CARTESIAN_POINT('Ctrl Pts',(8.33571713696631,-18.9493544240891,-24.8735000521768));
#49077=CARTESIAN_POINT('Ctrl Pts',(8.88883102789065,-19.0501590221844,-24.7985395646899));
#49078=CARTESIAN_POINT('Ctrl Pts',(9.58538130299016,-19.2109486375985,-24.6751859365789));
#49079=CARTESIAN_POINT('Ctrl Pts',(10.1375693358685,-19.3872925255919,-24.5321887728776));
#49080=CARTESIAN_POINT('Ctrl Pts',(11.3565468230311,-19.8503443148555,-24.1453469673367));
#49081=CARTESIAN_POINT('Ctrl Pts',(12.3228318792994,-20.4809300681266,-23.6358069932934));
#49082=CARTESIAN_POINT('Ctrl Pts',(13.2438497514686,-21.1419847785548,-23.0329488931636));
#49083=CARTESIAN_POINT('Ctrl Pts',(13.4536958211944,-21.2946007618859,-22.8895961528565));
#49084=CARTESIAN_POINT('Ctrl Pts',(13.5572593885355,-21.3699791139417,-22.8175746974478));
#49085=CARTESIAN_POINT('Ctrl Pts',(13.6160986444917,-21.4128228536293,-22.7762818189615));
#49086=CARTESIAN_POINT('Ctrl Pts',(13.645355806218,-21.4341190597128,-22.755631186663));
#49087=CARTESIAN_POINT('Ctrl Pts',(13.9304427285216,-21.6415024695375,-22.5539291559155));
#49088=CARTESIAN_POINT('Ctrl Pts',(14.4834792629394,-22.0842177076207,-22.1185350536073));
#49089=CARTESIAN_POINT('Ctrl Pts',(14.98335392639,-22.5380437985113,-21.6541002484824));
#49090=CARTESIAN_POINT('Ctrl Pts',(15.2260186760796,-22.7662639303248,-21.4137725438282));
#49091=CARTESIAN_POINT('Ctrl Pts',(2.1,-23.6060638405976,-31.0445557088918));
#49092=CARTESIAN_POINT('Ctrl Pts',(2.73333333333333,-23.6060638405976,-31.0445557088918));
#49093=CARTESIAN_POINT('Ctrl Pts',(3.36464153971337,-23.6061551620833,-31.0444583481246));
#49094=CARTESIAN_POINT('Ctrl Pts',(4.12085950545642,-23.6061797565327,-31.0444310988732));
#49095=CARTESIAN_POINT('Ctrl Pts',(4.34457587227524,-23.6026038074475,-31.0472140637149));
#49096=CARTESIAN_POINT('Ctrl Pts',(4.82871915333435,-23.5855404636303,-31.0605229321991));
#49097=CARTESIAN_POINT('Ctrl Pts',(5.71350842690898,-23.543739000069,-31.0931529169989));
#49098=CARTESIAN_POINT('Ctrl Pts',(6.55584786131197,-23.5404886370307,-31.0957210166559));
#49099=CARTESIAN_POINT('Ctrl Pts',(7.21833910031285,-23.6254456564365,-31.0291118651101));
#49100=CARTESIAN_POINT('Ctrl Pts',(7.34676118501293,-23.6425884371248,-31.0159144331966));
#49101=CARTESIAN_POINT('Ctrl Pts',(7.61957283623088,-23.6819205403188,-30.986195335862));
#49102=CARTESIAN_POINT('Ctrl Pts',(7.96026153975009,-23.7374867325871,-30.944960085127));
#49103=CARTESIAN_POINT('Ctrl Pts',(8.37794406069148,-23.8176688187955,-30.8854641795912));
#49104=CARTESIAN_POINT('Ctrl Pts',(8.93897958734005,-23.9451060235987,-30.7894856598615));
#49105=CARTESIAN_POINT('Ctrl Pts',(9.64589610894272,-24.1485645677299,-30.6314814118357));
#49106=CARTESIAN_POINT('Ctrl Pts',(10.2035826747735,-24.3705984027494,-30.4493953450365));
#49107=CARTESIAN_POINT('Ctrl Pts',(11.4269764335898,-24.9486838559586,-29.9611336557811));
#49108=CARTESIAN_POINT('Ctrl Pts',(12.3794613911947,-25.7205660291737,-29.3307527404956));
#49109=CARTESIAN_POINT('Ctrl Pts',(13.2972801181681,-26.536248516985,-28.5788115668798));
#49110=CARTESIAN_POINT('Ctrl Pts',(13.5062492987541,-26.7246568894861,-28.3998656781212));
#49111=CARTESIAN_POINT('Ctrl Pts',(13.6095218510944,-26.8178025811325,-28.30987870928));
#49112=CARTESIAN_POINT('Ctrl Pts',(13.6681948654715,-26.8707551741385,-28.2582726202542));
#49113=CARTESIAN_POINT('Ctrl Pts',(13.6973873567982,-26.8970881889659,-28.2324525330172));
#49114=CARTESIAN_POINT('Ctrl Pts',(13.9814825393856,-27.1533540380845,-27.980413093245));
#49115=CARTESIAN_POINT('Ctrl Pts',(14.5280933440888,-27.6942372345927,-27.4431392305571));
#49116=CARTESIAN_POINT('Ctrl Pts',(15.0243070371674,-28.25234233925,-26.8665204433862));
#49117=CARTESIAN_POINT('Ctrl Pts',(15.2656150130537,-28.5332835802564,-26.5678972425624));
#49118=CARTESIAN_POINT('',(3.2,-22.7328514723457,-29.9495820327475));
#49119=CARTESIAN_POINT('Ctrl Pts',(3.19847306248522,-22.7329107976785,-29.9495195044252));
#49120=CARTESIAN_POINT('Ctrl Pts',(3.06436549823724,-22.9285035669014,-30.1948090414568));
#49121=CARTESIAN_POINT('Ctrl Pts',(2.93026080897388,-23.1240595470582,-30.4400531793895));
#49122=CARTESIAN_POINT('Ctrl Pts',(2.79626461758213,-23.3193910750582,-30.6850129088235));
#49123=CARTESIAN_POINT('',(15.,-11.1762403838096,-11.1670787178359));
#49124=CARTESIAN_POINT('Ctrl Pts',(15.,-11.1762403838096,-11.1670787178359));
#49125=CARTESIAN_POINT('Ctrl Pts',(14.4897165779515,-11.3373685343331,-11.7879945733865));
#49126=CARTESIAN_POINT('Ctrl Pts',(13.983380302661,-11.5187060499957,-12.4208731978426));
#49127=CARTESIAN_POINT('Ctrl Pts',(13.4460287676664,-11.7567539704294,-13.1013698964346));
#49128=CARTESIAN_POINT('Ctrl Pts',(12.8282655681033,-12.0304244364084,-13.8836991361168));
#49129=CARTESIAN_POINT('Ctrl Pts',(12.155541408943,-12.3493763587429,-14.7928054072806));
#49130=CARTESIAN_POINT('Ctrl Pts',(11.5904908073501,-12.6688779184396,-15.5748537094225));
#49131=CARTESIAN_POINT('Ctrl Pts',(11.1143368259573,-12.9381138758599,-16.2338662149516));
#49132=CARTESIAN_POINT('Ctrl Pts',(10.6953158949572,-13.2106621367002,-16.8262345756793));
#49133=CARTESIAN_POINT('Ctrl Pts',(10.2957959918397,-13.5071054931829,-17.3951211088922));
#49134=CARTESIAN_POINT('Ctrl Pts',(10.0450888109402,-13.6931299631035,-17.7521094288247));
#49135=CARTESIAN_POINT('Ctrl Pts',(9.80235305581407,-13.8878822107991,-18.1003493308506));
#49136=CARTESIAN_POINT('Ctrl Pts',(9.56010106233158,-14.0947279826892,-18.4527330693702));
#49137=CARTESIAN_POINT('Ctrl Pts',(9.36613602939727,-14.2603441511269,-18.7348778000075));
#49138=CARTESIAN_POINT('Ctrl Pts',(9.15248571294299,-14.4499421458783,-19.0480702412718));
#49139=CARTESIAN_POINT('Ctrl Pts',(8.89022359824486,-14.6989807980091,-19.4411359839043));
#49140=CARTESIAN_POINT('Ctrl Pts',(8.39222406105985,-15.1718708059503,-20.1875135464416));
#49141=CARTESIAN_POINT('Ctrl Pts',(7.76643777374077,-15.8240081907589,-21.153333731125));
#49142=CARTESIAN_POINT('Ctrl Pts',(7.10363554123528,-16.6157830223697,-22.2694187973552));
#49143=CARTESIAN_POINT('Ctrl Pts',(6.23550018248711,-17.6528461066184,-23.7312619563649));
#49144=CARTESIAN_POINT('Ctrl Pts',(5.31040885822698,-19.033253690729,-25.3709340011067));
#49145=CARTESIAN_POINT('Ctrl Pts',(4.46416616904233,-20.4648153103685,-27.11999472538));
#49146=CARTESIAN_POINT('Ctrl Pts',(4.30741751124418,-20.7299819880861,-27.4439714337655));
#49147=CARTESIAN_POINT('Ctrl Pts',(4.15262292089009,-20.9971466932259,-27.7730770818396));
#49148=CARTESIAN_POINT('Ctrl Pts',(4.,-21.2644490398942,-28.1082636227258));
#49149=CARTESIAN_POINT('Ctrl Pts',(3.72434973283395,-21.7472203225005,-28.7136396632767));
#49150=CARTESIAN_POINT('Ctrl Pts',(3.45587123478816,-22.240150328922,-29.331754340573));
#49151=CARTESIAN_POINT('Ctrl Pts',(3.2,-22.7328514723457,-29.9495820327474));
#49152=CARTESIAN_POINT('',(15.,-22.0807120920212,-21.1849511094378));
#49153=CARTESIAN_POINT('Ctrl Pts',(15.,-22.0807120920212,-21.1849511094378));
#49154=CARTESIAN_POINT('Ctrl Pts',(15.,-18.8408082676135,-18.1865559292736));
#49155=CARTESIAN_POINT('Ctrl Pts',(15.,-14.9884313390737,-14.634232602943));
#49156=CARTESIAN_POINT('Ctrl Pts',(15.,-11.1762403838096,-11.1670787178359));
#49157=CARTESIAN_POINT('Ctrl Pts',(6.,-23.5490023259382,-31.0876903203335));
#49158=CARTESIAN_POINT('Ctrl Pts',(6.38595465246567,-23.2149712390509,-30.6675553675066));
#49159=CARTESIAN_POINT('Ctrl Pts',(6.77023648668261,-22.9202307074269,-30.25978773824));
#49160=CARTESIAN_POINT('Ctrl Pts',(7.13915213286206,-22.6798798515873,-29.8657998307839));
#49161=CARTESIAN_POINT('Ctrl Pts',(8.10667920093245,-22.049529902305,-28.8325176458075));
#49162=CARTESIAN_POINT('Ctrl Pts',(8.98019888747386,-21.6690144845904,-27.9844578967108));
#49163=CARTESIAN_POINT('Ctrl Pts',(9.46656009721089,-21.5060718063769,-27.502383186396));
#49164=CARTESIAN_POINT('Ctrl Pts',(9.65648624874925,-21.4424419872736,-27.3141309313826));
#49165=CARTESIAN_POINT('Ctrl Pts',(9.79228848853745,-21.4038352459001,-27.1792029279711));
#49166=CARTESIAN_POINT('Ctrl Pts',(9.94593825727835,-21.3652548270746,-27.0254911176928));
#49167=CARTESIAN_POINT('Ctrl Pts',(10.106574086601,-21.3249202556369,-26.8647904259633));
#49168=CARTESIAN_POINT('Ctrl Pts',(10.2660951669676,-21.291919485225,-26.7040013107996));
#49169=CARTESIAN_POINT('Ctrl Pts',(10.4261869573617,-21.2667017567949,-26.5402002816529));
#49170=CARTESIAN_POINT('Ctrl Pts',(10.8065549509411,-21.2067860250638,-26.151019370818));
#49171=CARTESIAN_POINT('Ctrl Pts',(11.1894211925257,-21.1918047278973,-25.7443677774521));
#49172=CARTESIAN_POINT('Ctrl Pts',(11.6023503255242,-21.2187986652524,-25.2875487721924));
#49173=CARTESIAN_POINT('Ctrl Pts',(11.7531893954247,-21.2286592928473,-25.1206771509872));
#49174=CARTESIAN_POINT('Ctrl Pts',(11.9080270687775,-21.2442649897398,-24.9470697549615));
#49175=CARTESIAN_POINT('Ctrl Pts',(12.068176613168,-21.2657353562899,-24.7650851418614));
#49176=CARTESIAN_POINT('Ctrl Pts',(12.1838435903475,-21.2812421902758,-24.6336479269097));
#49177=CARTESIAN_POINT('Ctrl Pts',(12.3100865410161,-21.2996793030358,-24.48952991587));
#49178=CARTESIAN_POINT('Ctrl Pts',(12.5127093730712,-21.3376417331468,-24.2542638313305));
#49179=CARTESIAN_POINT('Ctrl Pts',(12.7975492664042,-21.3910079527075,-23.9235352271283));
#49180=CARTESIAN_POINT('Ctrl Pts',(13.1874566943566,-21.4810061462248,-23.462026248552));
#49181=CARTESIAN_POINT('Ctrl Pts',(13.6431584568239,-21.600000204035,-22.9185284970073));
#49182=CARTESIAN_POINT('Ctrl Pts',(14.069523646534,-21.7113338178396,-22.4100193337122));
#49183=CARTESIAN_POINT('Ctrl Pts',(14.53311408767,-21.878316911732,-21.8202269155209));
#49184=CARTESIAN_POINT('Ctrl Pts',(15.,-22.0807120920212,-21.1849511094378));
#49185=CARTESIAN_POINT('Origin',(15.,-7.65823537717056,-3.68801178249924));
#49186=CARTESIAN_POINT('',(15.,-12.6367667846116,-9.48283298589492));
#49187=CARTESIAN_POINT('Ctrl Pts',(15.,-12.6367667846116,-9.48283298589491));
#49188=CARTESIAN_POINT('Ctrl Pts',(15.,-12.1910490642079,-10.0767937666962));
#49189=CARTESIAN_POINT('Ctrl Pts',(15.,-11.7031502151664,-10.6397366004717));
#49190=CARTESIAN_POINT('Ctrl Pts',(15.,-11.1762403838096,-11.1670787178359));
#49191=CARTESIAN_POINT('',(15.,-24.1202348804503,-18.8301425727982));
#49192=CARTESIAN_POINT('Ctrl Pts',(15.,-12.6367667846116,-9.48283298589491));
#49193=CARTESIAN_POINT('Ctrl Pts',(15.,-16.7264630501964,-12.8512910730167));
#49194=CARTESIAN_POINT('Ctrl Pts',(15.,-20.8784875564221,-16.2131979243164));
#49195=CARTESIAN_POINT('Ctrl Pts',(15.,-24.1202348804503,-18.8301425727982));
#49196=CARTESIAN_POINT('Origin',(15.,0.,0.));
#49197=CARTESIAN_POINT('Ctrl Pts',(15.,-27.569647357814,-13.2768424169973));
#49198=CARTESIAN_POINT('Ctrl Pts',(15.,-14.2928049408167,-40.8464897748113));
#49199=CARTESIAN_POINT('Ctrl Pts',(15.,13.2768424169973,-27.569647357814));
#49200=CARTESIAN_POINT('Ctrl Pts',(15.,40.8464897748113,-14.2928049408167));
#49201=CARTESIAN_POINT('Ctrl Pts',(15.,27.569647357814,13.2768424169973));
#49202=CARTESIAN_POINT('Ctrl Pts',(15.,14.2928049408167,40.8464897748113));
#49203=CARTESIAN_POINT('Ctrl Pts',(15.,-13.2768424169973,27.569647357814));
#49204=CARTESIAN_POINT('Ctrl Pts',(15.,-40.8464897748113,14.2928049408167));
#49205=CARTESIAN_POINT('Ctrl Pts',(15.,-27.569647357814,-13.2768424169973));
#49206=CARTESIAN_POINT('Ctrl Pts',(14.7843073131059,-27.6919221166174,-13.3357268373578));
#49207=CARTESIAN_POINT('Ctrl Pts',(14.7843073131059,-14.3561952792596,-41.0276489539752));
#49208=CARTESIAN_POINT('Ctrl Pts',(14.7843073131059,13.3357268373578,-27.6919221166174));
#49209=CARTESIAN_POINT('Ctrl Pts',(14.7843073131059,41.0276489539752,-14.3561952792596));
#49210=CARTESIAN_POINT('Ctrl Pts',(14.7843073131059,27.6919221166174,13.3357268373578));
#49211=CARTESIAN_POINT('Ctrl Pts',(14.7843073131059,14.3561952792596,41.0276489539752));
#49212=CARTESIAN_POINT('Ctrl Pts',(14.7843073131059,-13.3357268373578,27.6919221166174));
#49213=CARTESIAN_POINT('Ctrl Pts',(14.7843073131059,-41.0276489539752,14.3561952792596));
#49214=CARTESIAN_POINT('Ctrl Pts',(14.7843073131059,-27.6919221166174,-13.3357268373578));
#49215=CARTESIAN_POINT('Ctrl Pts',(14.3560298066371,-27.9390044129707,-13.4547154000382));
#49216=CARTESIAN_POINT('Ctrl Pts',(14.3560298066371,-14.4842890129325,-41.3937198130088));
#49217=CARTESIAN_POINT('Ctrl Pts',(14.3560298066371,13.4547154000382,-27.9390044129707));
#49218=CARTESIAN_POINT('Ctrl Pts',(14.3560298066371,41.3937198130088,-14.4842890129325));
#49219=CARTESIAN_POINT('Ctrl Pts',(14.3560298066371,27.9390044129707,13.4547154000382));
#49220=CARTESIAN_POINT('Ctrl Pts',(14.3560298066371,14.4842890129325,41.3937198130088));
#49221=CARTESIAN_POINT('Ctrl Pts',(14.3560298066371,-13.4547154000382,27.9390044129707));
#49222=CARTESIAN_POINT('Ctrl Pts',(14.3560298066371,-41.3937198130088,14.4842890129325));
#49223=CARTESIAN_POINT('Ctrl Pts',(14.3560298066371,-27.9390044129707,-13.4547154000382));
#49224=CARTESIAN_POINT('Ctrl Pts',(13.722936818686,-28.3172259246361,-13.6368572803433));
#49225=CARTESIAN_POINT('Ctrl Pts',(13.722936818686,-14.6803686442928,-41.9540832049794));
#49226=CARTESIAN_POINT('Ctrl Pts',(13.722936818686,13.6368572803433,-28.3172259246361));
#49227=CARTESIAN_POINT('Ctrl Pts',(13.722936818686,41.9540832049794,-14.6803686442928));
#49228=CARTESIAN_POINT('Ctrl Pts',(13.722936818686,28.3172259246361,13.6368572803433));
#49229=CARTESIAN_POINT('Ctrl Pts',(13.722936818686,14.6803686442928,41.9540832049794));
#49230=CARTESIAN_POINT('Ctrl Pts',(13.722936818686,-13.6368572803433,28.3172259246361));
#49231=CARTESIAN_POINT('Ctrl Pts',(13.722936818686,-41.9540832049794,14.6803686442928));
#49232=CARTESIAN_POINT('Ctrl Pts',(13.722936818686,-28.3172259246361,-13.6368572803433));
#49233=CARTESIAN_POINT('Ctrl Pts',(12.8977690042853,-28.8369697397467,-13.8871527099828));
#49234=CARTESIAN_POINT('Ctrl Pts',(12.8977690042853,-14.949817029764,-42.7241224497295));
#49235=CARTESIAN_POINT('Ctrl Pts',(12.8977690042853,13.8871527099828,-28.8369697397467));
#49236=CARTESIAN_POINT('Ctrl Pts',(12.8977690042853,42.7241224497295,-14.949817029764));
#49237=CARTESIAN_POINT('Ctrl Pts',(12.8977690042853,28.8369697397467,13.8871527099828));
#49238=CARTESIAN_POINT('Ctrl Pts',(12.8977690042853,14.949817029764,42.7241224497295));
#49239=CARTESIAN_POINT('Ctrl Pts',(12.8977690042853,-13.8871527099828,28.8369697397467));
#49240=CARTESIAN_POINT('Ctrl Pts',(12.8977690042853,-42.7241224497295,14.949817029764));
#49241=CARTESIAN_POINT('Ctrl Pts',(12.8977690042853,-28.8369697397467,-13.8871527099828));
#49242=CARTESIAN_POINT('Ctrl Pts',(11.9000549946031,-29.5141508562392,-14.2132659480213));
#49243=CARTESIAN_POINT('Ctrl Pts',(11.9000549946031,-15.3008849082179,-43.7274168042605));
#49244=CARTESIAN_POINT('Ctrl Pts',(11.9000549946031,14.2132659480213,-29.5141508562392));
#49245=CARTESIAN_POINT('Ctrl Pts',(11.9000549946031,43.7274168042605,-15.3008849082179));
#49246=CARTESIAN_POINT('Ctrl Pts',(11.9000549946031,29.5141508562392,14.2132659480213));
#49247=CARTESIAN_POINT('Ctrl Pts',(11.9000549946031,15.3008849082179,43.7274168042605));
#49248=CARTESIAN_POINT('Ctrl Pts',(11.9000549946031,-14.2132659480213,29.5141508562392));
#49249=CARTESIAN_POINT('Ctrl Pts',(11.9000549946031,-43.7274168042605,15.3008849082179));
#49250=CARTESIAN_POINT('Ctrl Pts',(11.9000549946031,-29.5141508562392,-14.2132659480213));
#49251=CARTESIAN_POINT('Ctrl Pts',(10.9391333834985,-30.2213162016529,-14.5538188296728));
#49252=CARTESIAN_POINT('Ctrl Pts',(10.9391333834985,-15.6674973719801,-44.7751350313257));
#49253=CARTESIAN_POINT('Ctrl Pts',(10.9391333834985,14.5538188296728,-30.2213162016529));
#49254=CARTESIAN_POINT('Ctrl Pts',(10.9391333834985,44.7751350313257,-15.6674973719801));
#49255=CARTESIAN_POINT('Ctrl Pts',(10.9391333834985,30.2213162016529,14.5538188296728));
#49256=CARTESIAN_POINT('Ctrl Pts',(10.9391333834985,15.6674973719801,44.7751350313257));
#49257=CARTESIAN_POINT('Ctrl Pts',(10.9391333834985,-14.5538188296728,30.2213162016529));
#49258=CARTESIAN_POINT('Ctrl Pts',(10.9391333834985,-44.7751350313257,15.6674973719801));
#49259=CARTESIAN_POINT('Ctrl Pts',(10.9391333834985,-30.2213162016529,-14.5538188296728));
#49260=CARTESIAN_POINT('Ctrl Pts',(10.0180552497783,-30.9609522745316,-14.9100087895256));
#49261=CARTESIAN_POINT('Ctrl Pts',(10.0180552497783,-16.050943485006,-45.8709610640572));
#49262=CARTESIAN_POINT('Ctrl Pts',(10.0180552497783,14.9100087895256,-30.9609522745316));
#49263=CARTESIAN_POINT('Ctrl Pts',(10.0180552497783,45.8709610640572,-16.050943485006));
#49264=CARTESIAN_POINT('Ctrl Pts',(10.0180552497783,30.9609522745316,14.9100087895256));
#49265=CARTESIAN_POINT('Ctrl Pts',(10.0180552497783,16.050943485006,45.8709610640572));
#49266=CARTESIAN_POINT('Ctrl Pts',(10.0180552497783,-14.9100087895256,30.9609522745316));
#49267=CARTESIAN_POINT('Ctrl Pts',(10.0180552497783,-45.8709610640572,16.050943485006));
#49268=CARTESIAN_POINT('Ctrl Pts',(10.0180552497783,-30.9609522745316,-14.9100087895256));
#49269=CARTESIAN_POINT('Ctrl Pts',(9.13857394886632,-31.734487984447,-15.2825239541621));
#49270=CARTESIAN_POINT('Ctrl Pts',(9.13857394886632,-16.4519640302848,-47.0170119386091));
#49271=CARTESIAN_POINT('Ctrl Pts',(9.13857394886632,15.2825239541621,-31.734487984447));
#49272=CARTESIAN_POINT('Ctrl Pts',(9.13857394886632,47.0170119386091,-16.4519640302848));
#49273=CARTESIAN_POINT('Ctrl Pts',(9.13857394886632,31.734487984447,15.2825239541621));
#49274=CARTESIAN_POINT('Ctrl Pts',(9.13857394886632,16.4519640302848,47.0170119386091));
#49275=CARTESIAN_POINT('Ctrl Pts',(9.13857394886632,-15.2825239541621,31.734487984447));
#49276=CARTESIAN_POINT('Ctrl Pts',(9.13857394886632,-47.0170119386091,16.4519640302848));
#49277=CARTESIAN_POINT('Ctrl Pts',(9.13857394886632,-31.734487984447,-15.2825239541621));
#49278=CARTESIAN_POINT('Ctrl Pts',(8.29915429043693,-32.5406722170424,-15.6707618186629));
#49279=CARTESIAN_POINT('Ctrl Pts',(8.29915429043693,-16.8699103983795,-48.2114340357053));
#49280=CARTESIAN_POINT('Ctrl Pts',(8.29915429043693,15.6707618186629,-32.5406722170424));
#49281=CARTESIAN_POINT('Ctrl Pts',(8.29915429043693,48.2114340357053,-16.8699103983795));
#49282=CARTESIAN_POINT('Ctrl Pts',(8.29915429043693,32.5406722170424,15.6707618186629));
#49283=CARTESIAN_POINT('Ctrl Pts',(8.29915429043693,16.8699103983795,48.2114340357053));
#49284=CARTESIAN_POINT('Ctrl Pts',(8.29915429043693,-15.6707618186629,32.5406722170424));
#49285=CARTESIAN_POINT('Ctrl Pts',(8.29915429043693,-48.2114340357053,16.8699103983795));
#49286=CARTESIAN_POINT('Ctrl Pts',(8.29915429043693,-32.5406722170424,-15.6707618186629));
#49287=CARTESIAN_POINT('Ctrl Pts',(7.4968190344241,-33.3770786491896,-16.0735539273924));
#49288=CARTESIAN_POINT('Ctrl Pts',(7.4968190344241,-17.3035247217972,-49.450632576582));
#49289=CARTESIAN_POINT('Ctrl Pts',(7.4968190344241,16.0735539273924,-33.3770786491896));
#49290=CARTESIAN_POINT('Ctrl Pts',(7.4968190344241,49.450632576582,-17.3035247217972));
#49291=CARTESIAN_POINT('Ctrl Pts',(7.4968190344241,33.3770786491896,16.0735539273924));
#49292=CARTESIAN_POINT('Ctrl Pts',(7.4968190344241,17.3035247217972,49.450632576582));
#49293=CARTESIAN_POINT('Ctrl Pts',(7.4968190344241,-16.0735539273924,33.3770786491896));
#49294=CARTESIAN_POINT('Ctrl Pts',(7.4968190344241,-49.450632576582,17.3035247217972));
#49295=CARTESIAN_POINT('Ctrl Pts',(7.4968190344241,-33.3770786491896,-16.0735539273924));
#49296=CARTESIAN_POINT('Ctrl Pts',(6.88220761950379,-34.0684169111937,-16.4064848873841));
#49297=CARTESIAN_POINT('Ctrl Pts',(6.88220761950379,-17.6619320238096,-50.4749017985778));
#49298=CARTESIAN_POINT('Ctrl Pts',(6.88220761950379,16.4064848873841,-34.0684169111937));
#49299=CARTESIAN_POINT('Ctrl Pts',(6.88220761950379,50.4749017985778,-17.6619320238096));
#49300=CARTESIAN_POINT('Ctrl Pts',(6.88220761950379,34.0684169111937,16.4064848873841));
#49301=CARTESIAN_POINT('Ctrl Pts',(6.88220761950379,17.6619320238096,50.4749017985778));
#49302=CARTESIAN_POINT('Ctrl Pts',(6.88220761950379,-16.4064848873841,34.0684169111937));
#49303=CARTESIAN_POINT('Ctrl Pts',(6.88220761950379,-50.4749017985778,17.6619320238096));
#49304=CARTESIAN_POINT('Ctrl Pts',(6.88220761950379,-34.0684169111937,-16.4064848873841));
#49305=CARTESIAN_POINT('Ctrl Pts',(6.43560997955544,-34.5986241433973,-16.6618192331215));
#49306=CARTESIAN_POINT('Ctrl Pts',(6.43560997955544,-17.9368049102758,-51.2604433765188));
#49307=CARTESIAN_POINT('Ctrl Pts',(6.43560997955544,16.6618192331215,-34.5986241433973));
#49308=CARTESIAN_POINT('Ctrl Pts',(6.43560997955544,51.2604433765188,-17.9368049102758));
#49309=CARTESIAN_POINT('Ctrl Pts',(6.43560997955544,34.5986241433973,16.6618192331215));
#49310=CARTESIAN_POINT('Ctrl Pts',(6.43560997955544,17.9368049102758,51.2604433765188));
#49311=CARTESIAN_POINT('Ctrl Pts',(6.43560997955544,-16.6618192331215,34.5986241433973));
#49312=CARTESIAN_POINT('Ctrl Pts',(6.43560997955544,-51.2604433765188,17.9368049102758));
#49313=CARTESIAN_POINT('Ctrl Pts',(6.43560997955544,-34.5986241433973,-16.6618192331215));
#49314=CARTESIAN_POINT('Ctrl Pts',(6.14415685965718,-34.9572124542593,-16.8345062622337));
#49315=CARTESIAN_POINT('Ctrl Pts',(6.14415685965718,-18.1227061920256,-51.791718716493));
#49316=CARTESIAN_POINT('Ctrl Pts',(6.14415685965718,16.8345062622337,-34.9572124542593));
#49317=CARTESIAN_POINT('Ctrl Pts',(6.14415685965718,51.791718716493,-18.1227061920256));
#49318=CARTESIAN_POINT('Ctrl Pts',(6.14415685965718,34.9572124542593,16.8345062622337));
#49319=CARTESIAN_POINT('Ctrl Pts',(6.14415685965718,18.1227061920256,51.791718716493));
#49320=CARTESIAN_POINT('Ctrl Pts',(6.14415685965718,-16.8345062622337,34.9572124542593));
#49321=CARTESIAN_POINT('Ctrl Pts',(6.14415685965718,-51.791718716493,18.1227061920256));
#49322=CARTESIAN_POINT('Ctrl Pts',(6.14415685965718,-34.9572124542593,-16.8345062622337));
#49323=CARTESIAN_POINT('Ctrl Pts',(6.,-35.1377858481943,-16.9214658255848));
#49324=CARTESIAN_POINT('Ctrl Pts',(6.,-18.2163200226096,-52.0592516737791));
#49325=CARTESIAN_POINT('Ctrl Pts',(6.,16.9214658255848,-35.1377858481943));
#49326=CARTESIAN_POINT('Ctrl Pts',(6.,52.0592516737791,-18.2163200226096));
#49327=CARTESIAN_POINT('Ctrl Pts',(6.,35.1377858481943,16.9214658255848));
#49328=CARTESIAN_POINT('Ctrl Pts',(6.,18.2163200226096,52.0592516737791));
#49329=CARTESIAN_POINT('Ctrl Pts',(6.,-16.9214658255848,35.1377858481943));
#49330=CARTESIAN_POINT('Ctrl Pts',(6.,-52.0592516737791,18.2163200226096));
#49331=CARTESIAN_POINT('Ctrl Pts',(6.,-35.1377858481943,-16.9214658255848));
#49332=CARTESIAN_POINT('Ctrl Pts',(15.,-24.1202348804503,-18.8301425727982));
#49333=CARTESIAN_POINT('Ctrl Pts',(14.0108432136945,-23.6906926400127,-20.3917630740682));
#49334=CARTESIAN_POINT('Ctrl Pts',(13.3692319443824,-23.3579535391276,-21.3915618529718));
#49335=CARTESIAN_POINT('Ctrl Pts',(12.3476991724842,-23.1473185206879,-22.7113896892958));
#49336=CARTESIAN_POINT('Ctrl Pts',(12.025018705019,-23.0807834000492,-23.1282952207817));
#49337=CARTESIAN_POINT('Ctrl Pts',(11.6666317570708,-23.0126114746088,-23.5919571633962));
#49338=CARTESIAN_POINT('Ctrl Pts',(11.3593868751763,-22.9704586633353,-23.9823118033932));
#49339=CARTESIAN_POINT('Ctrl Pts',(10.676771680913,-22.876806494815,-24.8495744466962));
#49340=CARTESIAN_POINT('Ctrl Pts',(10.1321636914396,-22.8734798744455,-25.510224320219));
#49341=CARTESIAN_POINT('Ctrl Pts',(9.56604173138329,-22.9954906247793,-26.139747689115));
#49342=CARTESIAN_POINT('Ctrl Pts',(9.34563078589189,-23.0429936484008,-26.3848430055616));
#49343=CARTESIAN_POINT('Ctrl Pts',(9.12222951098696,-23.1101461905759,-26.6250740206507));
#49344=CARTESIAN_POINT('Ctrl Pts',(8.88860711505281,-23.1970883230411,-26.8731231743128));
#49345=CARTESIAN_POINT('Ctrl Pts',(8.75830600700747,-23.2455796337767,-27.0114706963585));
#49346=CARTESIAN_POINT('Ctrl Pts',(8.62340343546558,-23.2985805913255,-27.1537906260844));
#49347=CARTESIAN_POINT('Ctrl Pts',(8.40819516300432,-23.3978248652992,-27.3800488166559));
#49348=CARTESIAN_POINT('Ctrl Pts',(8.02443006829141,-23.5747998847334,-27.7835184181781));
#49349=CARTESIAN_POINT('Ctrl Pts',(7.46417034513348,-23.8812360292217,-28.3671329236259));
#49350=CARTESIAN_POINT('Ctrl Pts',(6.85957019142019,-24.290054208171,-29.0329567468316));
#49351=CARTESIAN_POINT('Ctrl Pts',(6.58024553736739,-24.4789277896681,-29.3405666737144));
#49352=CARTESIAN_POINT('Ctrl Pts',(6.28976782192773,-24.7075513257838,-29.6525862691847));
#49353=CARTESIAN_POINT('Ctrl Pts',(6.,-24.9583551264995,-29.9679914138325));
#49354=CARTESIAN_POINT('Ctrl Pts',(2.09999999999999,-10.543135638033,-11.7771860002428));
#49355=CARTESIAN_POINT('Ctrl Pts',(2.73333333333333,-10.543135638033,-11.7771860002428));
#49356=CARTESIAN_POINT('Ctrl Pts',(3.36803272841208,-10.5431022073082,-11.7772201003177));
#49357=CARTESIAN_POINT('Ctrl Pts',(4.25276821260583,-10.5430810365691,-11.7772406600604));
#49358=CARTESIAN_POINT('Ctrl Pts',(4.7726650406829,-10.5368654902041,-11.7829280689769));
#49359=CARTESIAN_POINT('Ctrl Pts',(5.76856525243156,-10.5188745659,-11.7994589520322));
#49360=CARTESIAN_POINT('Ctrl Pts',(6.48507937940904,-10.5193931210859,-11.7990555387649));
#49361=CARTESIAN_POINT('Ctrl Pts',(6.99865688135792,-10.5442264472673,-11.7759801222031));
#49362=CARTESIAN_POINT('Ctrl Pts',(7.1247961420266,-10.5505968365102,-11.770213186573));
#49363=CARTESIAN_POINT('Ctrl Pts',(7.37169888445177,-10.564127314078,-11.7581967415648));
#49364=CARTESIAN_POINT('Ctrl Pts',(7.68210670520103,-10.5832981179727,-11.7415107170204));
#49365=CARTESIAN_POINT('Ctrl Pts',(8.05073427412801,-10.6102522860635,-11.7180831591284));
#49366=CARTESIAN_POINT('Ctrl Pts',(8.41503345999962,-10.641639777048,-11.6904177872868));
#49367=CARTESIAN_POINT('Ctrl Pts',(9.01074144008478,-10.7021842311636,-11.6357976675359));
#49368=CARTESIAN_POINT('Ctrl Pts',(9.4630915836405,-10.7645290505238,-11.5767471383662));
#49369=CARTESIAN_POINT('Ctrl Pts',(10.2678427399453,-10.9068861685958,-11.4344468552384));
#49370=CARTESIAN_POINT('Ctrl Pts',(10.9804879072974,-11.0906707746144,-11.2592289323592));
#49371=CARTESIAN_POINT('Ctrl Pts',(11.7910205592258,-11.3518074464669,-10.996769538782));
#49372=CARTESIAN_POINT('Ctrl Pts',(12.2471496193426,-11.5059150850389,-10.8342802498727));
#49373=CARTESIAN_POINT('Ctrl Pts',(12.4732460256849,-11.5832901851512,-10.7494488910709));
#49374=CARTESIAN_POINT('Ctrl Pts',(12.8351174828998,-11.7067525897982,-10.6107180331633));
#49375=CARTESIAN_POINT('Ctrl Pts',(13.2802512034868,-11.872521853359,-10.4216414569813));
#49376=CARTESIAN_POINT('Ctrl Pts',(14.1612564248657,-12.2443027142459,-9.98781870483396));
#49377=CARTESIAN_POINT('Ctrl Pts',(14.7820737708942,-12.5376840654805,-9.62062677307173));
#49378=CARTESIAN_POINT('Ctrl Pts',(15.1979896574214,-12.7275569106452,-9.35997935634041));
#49379=CARTESIAN_POINT('Ctrl Pts',(2.09999999999999,-15.3665400340489,-17.8255438053547));
#49380=CARTESIAN_POINT('Ctrl Pts',(2.73333333333333,-15.3665400340489,-17.8255438053547));
#49381=CARTESIAN_POINT('Ctrl Pts',(3.3687181809592,-15.3665376853649,-17.825543073398));
#49382=CARTESIAN_POINT('Ctrl Pts',(4.2541517406304,-15.3665263774122,-17.8255511225364));
#49383=CARTESIAN_POINT('Ctrl Pts',(4.78309364461817,-15.3570547633814,-17.8338945202897));
#49384=CARTESIAN_POINT('Ctrl Pts',(5.77493293929972,-15.3298480612272,-17.8579711392587));
#49385=CARTESIAN_POINT('Ctrl Pts',(6.47496215402976,-15.3309764425276,-17.8570616603784));
#49386=CARTESIAN_POINT('Ctrl Pts',(6.96726328871316,-15.3675608640459,-17.824319195921));
#49387=CARTESIAN_POINT('Ctrl Pts',(7.09308121852369,-15.377187236198,-17.8159278901612));
#49388=CARTESIAN_POINT('Ctrl Pts',(7.33628060567667,-15.3974710703976,-17.7985922469198));
#49389=CARTESIAN_POINT('Ctrl Pts',(7.64235593139221,-15.4262403669694,-17.7744996748306));
#49390=CARTESIAN_POINT('Ctrl Pts',(8.00391129102422,-15.4665370619219,-17.7408214399693));
#49391=CARTESIAN_POINT('Ctrl Pts',(8.36000437958409,-15.513400053435,-17.7010966390644));
#49392=CARTESIAN_POINT('Ctrl Pts',(8.9396712633142,-15.6034591512378,-17.6229736918479));
#49393=CARTESIAN_POINT('Ctrl Pts',(9.37528665277327,-15.6958982632444,-17.5387083063492));
#49394=CARTESIAN_POINT('Ctrl Pts',(10.1433938392068,-15.9053466146459,-17.3372073728695));
#49395=CARTESIAN_POINT('Ctrl Pts',(10.8342866476536,-16.1779457660886,-17.0879562123254));
#49396=CARTESIAN_POINT('Ctrl Pts',(11.6346749715978,-16.5710483980858,-16.7090772220389));
#49397=CARTESIAN_POINT('Ctrl Pts',(12.0872491273666,-16.8040533312314,-16.4733694239515));
#49398=CARTESIAN_POINT('Ctrl Pts',(12.3122412108241,-16.9213946705885,-16.3499117769089));
#49399=CARTESIAN_POINT('Ctrl Pts',(12.6725812427255,-17.1088177167675,-16.1477879438135));
#49400=CARTESIAN_POINT('Ctrl Pts',(13.1110124042394,-17.358752386583,-15.8749798027102));
#49401=CARTESIAN_POINT('Ctrl Pts',(13.9921319659501,-17.9251842036961,-15.2424196482269));
#49402=CARTESIAN_POINT('Ctrl Pts',(14.6125773377935,-18.3745300756618,-14.7038806929422));
#49403=CARTESIAN_POINT('Ctrl Pts',(15.0291266285127,-18.6654710972975,-14.3214960647507));
#49404=CARTESIAN_POINT('Ctrl Pts',(2.09999999999999,-20.1899444300649,-23.8739016104667));
#49405=CARTESIAN_POINT('Ctrl Pts',(2.73333333333333,-20.1899444300649,-23.8739016104667));
#49406=CARTESIAN_POINT('Ctrl Pts',(3.36945279028916,-20.1899202539663,-23.8739271559913));
#49407=CARTESIAN_POINT('Ctrl Pts',(4.2556151808724,-20.1898901685131,-23.873954635471));
#49408=CARTESIAN_POINT('Ctrl Pts',(4.79358405809382,-20.1769973476943,-23.8850954394867));
#49409=CARTESIAN_POINT('Ctrl Pts',(5.781457677744,-20.1406055273539,-23.9166958135384));
#49410=CARTESIAN_POINT('Ctrl Pts',(6.46486276385338,-20.1426565583293,-23.9150612533684));
#49411=CARTESIAN_POINT('Ctrl Pts',(6.93654238579164,-20.1893583815516,-23.8739698938311));
#49412=CARTESIAN_POINT('Ctrl Pts',(7.06205421776047,-20.2022104664193,-23.8629801928831));
#49413=CARTESIAN_POINT('Ctrl Pts',(7.30168521565929,-20.2289421717304,-23.8405729535745));
#49414=CARTESIAN_POINT('Ctrl Pts',(7.60366388861905,-20.2668688425343,-23.809441722807));
#49415=CARTESIAN_POINT('Ctrl Pts',(7.95860109522663,-20.3197565331949,-23.7661259375574));
#49416=CARTESIAN_POINT('Ctrl Pts',(8.30730975845261,-20.3809946218758,-23.7152635567132));
#49417=CARTESIAN_POINT('Ctrl Pts',(8.8731012800961,-20.4982979004896,-23.615516281743));
#49418=CARTESIAN_POINT('Ctrl Pts',(9.29618129829887,-20.6175188842592,-23.508902976663));
#49419=CARTESIAN_POINT('Ctrl Pts',(10.0462711259633,-20.8875329990534,-23.2540694624143));
#49420=CARTESIAN_POINT('Ctrl Pts',(10.7405155672895,-21.2491820582357,-22.9313257121034));
#49421=CARTESIAN_POINT('Ctrl Pts',(11.5482234021021,-21.7792041800607,-22.4320578933702));
#49422=CARTESIAN_POINT('Ctrl Pts',(12.0041785857202,-22.0933306986234,-22.121270230917));
#49423=CARTESIAN_POINT('Ctrl Pts',(12.2304118102814,-22.2514886727216,-21.9584788027488));
#49424=CARTESIAN_POINT('Ctrl Pts',(12.5924512492605,-22.5039758796212,-21.6920608765541));
#49425=CARTESIAN_POINT('Ctrl Pts',(13.0427785940057,-22.8464337698471,-21.3273673525245));
#49426=CARTESIAN_POINT('Ctrl Pts',(13.9385893244826,-23.6198877956831,-20.4820953239141));
#49427=CARTESIAN_POINT('Ctrl Pts',(14.5670688438605,-24.2303643403375,-19.7648571735367));
#49428=CARTESIAN_POINT('Ctrl Pts',(14.9853697475044,-24.6233676158593,-19.2582596049827));
#49429=CARTESIAN_POINT('Ctrl Pts',(2.09999999999999,-25.0133488260808,-29.9222594155786));
#49430=CARTESIAN_POINT('Ctrl Pts',(2.73333333333333,-25.0133488260808,-29.9222594155786));
#49431=CARTESIAN_POINT('Ctrl Pts',(3.3702033632722,-25.0133137772673,-29.9223022183699));
#49432=CARTESIAN_POINT('Ctrl Pts',(4.25711862532379,-25.0132696203947,-29.9223453341099));
#49433=CARTESIAN_POINT('Ctrl Pts',(4.80402085288096,-24.9968125168733,-29.9363970223899));
#49434=CARTESIAN_POINT('Ctrl Pts',(5.78813313564812,-24.951309348524,-29.9754629517883));
#49435=CARTESIAN_POINT('Ctrl Pts',(6.45445006013163,-24.9545928566979,-29.9728540151355));
#49436=CARTESIAN_POINT('Ctrl Pts',(6.90690581340697,-25.0101128882108,-29.9244532685749));
#49437=CARTESIAN_POINT('Ctrl Pts',(7.0321416409966,-25.0261697865242,-29.9108828348662));
#49438=CARTESIAN_POINT('Ctrl Pts',(7.26849200273963,-25.0591138242421,-29.8835944575659));
#49439=CARTESIAN_POINT('Ctrl Pts',(7.56683080333734,-25.1059083784109,-29.8456606556004));
#49440=CARTESIAN_POINT('Ctrl Pts',(7.91604722627538,-25.1709090389714,-29.7930989156434));
#49441=CARTESIAN_POINT('Ctrl Pts',(8.25884332748362,-25.2460113850425,-29.7315240189041));
#49442=CARTESIAN_POINT('Ctrl Pts',(8.8142690913405,-25.3898037321514,-29.61079095463));
#49443=CARTESIAN_POINT('Ctrl Pts',(9.23053436408081,-25.5358852579794,-29.4818139880829));
#49444=CARTESIAN_POINT('Ctrl Pts',(9.97649801930199,-25.8720992258963,-29.16894819951));
#49445=CARTESIAN_POINT('Ctrl Pts',(10.6790198772432,-26.3323429661403,-28.7642792997449));
#49446=CARTESIAN_POINT('Ctrl Pts',(11.4920869896606,-27.0039397656116,-28.1395712188247));
#49447=CARTESIAN_POINT('Ctrl Pts',(11.9504399507504,-27.4008484986125,-27.7516435052251));
#49448=CARTESIAN_POINT('Ctrl Pts',(12.1774700011005,-27.6002581978098,-27.5488212641388));
#49449=CARTESIAN_POINT('Ctrl Pts',(12.540670686897,-27.9183822175908,-27.2171066391423));
#49450=CARTESIAN_POINT('Ctrl Pts',(12.9976730423846,-28.3567980745589,-26.7563181574512));
#49451=CARTESIAN_POINT('Ctrl Pts',(13.8993991018205,-29.3371347665202,-25.6964971094244));
#49452=CARTESIAN_POINT('Ctrl Pts',(14.5324532885843,-30.1082433886537,-24.7996310338783));
#49453=CARTESIAN_POINT('Ctrl Pts',(14.9514110803021,-30.6026094817751,-24.1685815379353));
#49454=CARTESIAN_POINT('',(3.2,-24.1401481407882,-28.8273003894017));
#49455=CARTESIAN_POINT('Ctrl Pts',(3.2,-24.1401481407882,-28.8273003894017));
#49456=CARTESIAN_POINT('Ctrl Pts',(3.56152274835421,-23.4440063035266,-27.9543661360881));
#49457=CARTESIAN_POINT('Ctrl Pts',(3.95224584525397,-22.743573003028,-27.0667464745569));
#49458=CARTESIAN_POINT('Ctrl Pts',(4.787674301238,-21.3221368163265,-25.3199081516513));
#49459=CARTESIAN_POINT('Ctrl Pts',(5.2151394623216,-20.6296286000308,-24.4935406264987));
#49460=CARTESIAN_POINT('Ctrl Pts',(6.79548775402686,-18.2759304665965,-21.5959335780027));
#49461=CARTESIAN_POINT('Ctrl Pts',(7.94016295939582,-17.0442366760427,-19.7414374675915));
#49462=CARTESIAN_POINT('Ctrl Pts',(9.46271935276147,-15.5713230036123,-17.3844072806034));
#49463=CARTESIAN_POINT('Ctrl Pts',(10.1385443659149,-15.0481496226839,-16.3651968434456));
#49464=CARTESIAN_POINT('Ctrl Pts',(11.5967860400763,-14.1711568382327,-14.1885864925966));
#49465=CARTESIAN_POINT('Ctrl Pts',(12.3997356677094,-13.7376588526878,-13.0379046765038));
#49466=CARTESIAN_POINT('Ctrl Pts',(13.6850585208087,-13.1354996003446,-11.2495034212006));
#49467=CARTESIAN_POINT('Ctrl Pts',(14.3457395898605,-12.8831452960905,-10.3354978215121));
#49468=CARTESIAN_POINT('Ctrl Pts',(15.,-12.6367667846116,-9.48283298589492));
#49469=CARTESIAN_POINT('Ctrl Pts',(2.79814976461967,-24.7266470076605,-29.5627760094694));
#49470=CARTESIAN_POINT('Ctrl Pts',(2.93285977270366,-24.531202871586,-29.3177067107927));
#49471=CARTESIAN_POINT('Ctrl Pts',(3.06772729768953,-24.3356333359279,-29.0724818414568));
#49472=CARTESIAN_POINT('Ctrl Pts',(3.2025793347187,-24.1401219978448,-28.8273304373552));
#49473=CARTESIAN_POINT('Origin',(2.9,0.,0.));
#49474=CARTESIAN_POINT('',(3.2,-33.4762280926097,-17.1202264205697));
#49475=CARTESIAN_POINT('Origin',(3.2,0.,0.));
#49476=CARTESIAN_POINT('Ctrl Pts',(3.19855924658779,-33.4762497065829,-17.1201427543021));
#49477=CARTESIAN_POINT('Ctrl Pts',(3.06443679751087,-33.7588989525607,-17.2562771750589));
#49478=CARTESIAN_POINT('Ctrl Pts',(2.9303164767804,-34.0414969702962,-17.3923866976636));
#49479=CARTESIAN_POINT('Ctrl Pts',(2.79630592797694,-34.3237709021223,-17.5283375865302));
#49480=CARTESIAN_POINT('Ctrl Pts',(2.1,-15.7838176169527,-0.899999999999997));
#49481=CARTESIAN_POINT('Ctrl Pts',(2.73333333333333,-15.7838176169527,-0.899999999999997));
#49482=CARTESIAN_POINT('Ctrl Pts',(3.36596566980363,-15.7838088294802,-0.89991334692306));
#49483=CARTESIAN_POINT('Ctrl Pts',(4.12347559197154,-15.7838060309894,-0.899886769079504));
#49484=CARTESIAN_POINT('Ctrl Pts',(4.36306874504969,-15.7837152633585,-0.901834641161809));
#49485=CARTESIAN_POINT('Ctrl Pts',(4.85755348006649,-15.7833089582346,-0.910820654567172));
#49486=CARTESIAN_POINT('Ctrl Pts',(5.73897272285415,-15.7823612829529,-0.932201228099064));
#49487=CARTESIAN_POINT('Ctrl Pts',(6.52603489331944,-15.782348631485,-0.93280713780616));
#49488=CARTESIAN_POINT('Ctrl Pts',(7.1275435062192,-15.7839622361425,-0.893118870461858));
#49489=CARTESIAN_POINT('Ctrl Pts',(7.25503875736122,-15.7844067237825,-0.884431863337579));
#49490=CARTESIAN_POINT('Ctrl Pts',(7.51729728777054,-15.7855650629912,-0.865241085102853));
#49491=CARTESIAN_POINT('Ctrl Pts',(7.84586404221675,-15.7874367544175,-0.838250317529829));
#49492=CARTESIAN_POINT('Ctrl Pts',(8.24414264130042,-15.7901251990884,-0.799706719121714));
#49493=CARTESIAN_POINT('Ctrl Pts',(8.77644186211642,-15.7939497820795,-0.738435083081115));
#49494=CARTESIAN_POINT('Ctrl Pts',(9.44111162245666,-15.7985731396741,-0.640296638236062));
#49495=CARTESIAN_POINT('Ctrl Pts',(9.96386140770947,-15.8006687624932,-0.531294988793781));
#49496=CARTESIAN_POINT('Ctrl Pts',(11.1188881593647,-15.801839487482,-0.242371579936367));
#49497=CARTESIAN_POINT('Ctrl Pts',(12.080426103097,-15.8109272922644,0.160862502399577));
#49498=CARTESIAN_POINT('Ctrl Pts',(13.0008162933431,-15.7944409326678,0.612453502691948));
#49499=CARTESIAN_POINT('Ctrl Pts',(13.210793498058,-15.7890467971084,0.718001212690115));
#49500=CARTESIAN_POINT('Ctrl Pts',(13.3144168382157,-15.7859213877517,0.770572988426763));
#49501=CARTESIAN_POINT('Ctrl Pts',(13.3732968497844,-15.784008942705,0.800566234451453));
#49502=CARTESIAN_POINT('Ctrl Pts',(13.4025760150423,-15.7830115107287,0.815517600240429));
#49503=CARTESIAN_POINT('Ctrl Pts',(13.6877720326255,-15.7730387773425,0.961314730638964));
#49504=CARTESIAN_POINT('Ctrl Pts',(14.2465760997328,-15.7491595629163,1.27594900526736));
#49505=CARTESIAN_POINT('Ctrl Pts',(14.7537307590314,-15.7175740225323,1.606813173185));
#49506=CARTESIAN_POINT('Ctrl Pts',(14.9999999999997,-15.6990456112166,1.77537689056615));
#49507=CARTESIAN_POINT('Ctrl Pts',(2.1,-23.5191287709962,-0.899999999999997));
#49508=CARTESIAN_POINT('Ctrl Pts',(2.73333333333333,-23.5191287709962,-0.899999999999997));
#49509=CARTESIAN_POINT('Ctrl Pts',(3.3655781264468,-23.5191252884321,-0.899935556524944));
#49510=CARTESIAN_POINT('Ctrl Pts',(4.12267126809373,-23.5191242310313,-0.89991735126274));
#49511=CARTESIAN_POINT('Ctrl Pts',(4.35698403697962,-23.5190465734764,-0.902785708978077));
#49512=CARTESIAN_POINT('Ctrl Pts',(4.84798634051153,-23.5186994574573,-0.916113399717105));
#49513=CARTESIAN_POINT('Ctrl Pts',(5.73067052875929,-23.5178866627675,-0.948008744665266));
#49514=CARTESIAN_POINT('Ctrl Pts',(6.535923680173,-23.517885158871,-0.949379309188695));
#49515=CARTESIAN_POINT('Ctrl Pts',(7.15867348703883,-23.5192670336036,-0.888884811529982));
#49516=CARTESIAN_POINT('Ctrl Pts',(7.28649833326676,-23.5196879006994,-0.875917985293893));
#49517=CARTESIAN_POINT('Ctrl Pts',(7.55246203150236,-23.5208922670236,-0.847060977328295));
#49518=CARTESIAN_POINT('Ctrl Pts',(7.88538697752817,-23.5229509940679,-0.806514180409723));
#49519=CARTESIAN_POINT('Ctrl Pts',(8.29074120651406,-23.5259132916756,-0.748419508807197));
#49520=CARTESIAN_POINT('Ctrl Pts',(8.8340108396217,-23.5299680738502,-0.655942701497698));
#49521=CARTESIAN_POINT('Ctrl Pts',(9.51595482357549,-23.5342272010875,-0.507323297625138));
#49522=CARTESIAN_POINT('Ctrl Pts',(10.0562747286729,-23.5344392632137,-0.341535964232884));
#49523=CARTESIAN_POINT('Ctrl Pts',(11.2545001865845,-23.5284609002258,0.0994030366123566));
#49524=CARTESIAN_POINT('Ctrl Pts',(12.2341579615793,-23.5306916466498,0.708875196748114));
#49525=CARTESIAN_POINT('Ctrl Pts',(13.1607568713765,-23.4927543604707,1.38402604346733));
#49526=CARTESIAN_POINT('Ctrl Pts',(13.3718579954519,-23.4815829003965,1.54166599939733));
#49527=CARTESIAN_POINT('Ctrl Pts',(13.4759064249217,-23.4753563425579,1.62011007351799));
#49528=CARTESIAN_POINT('Ctrl Pts',(13.5350103301451,-23.4716106415352,1.66485146824944));
#49529=CARTESIAN_POINT('Ctrl Pts',(13.5643801112264,-23.4696762113674,1.68714788583071));
#49530=CARTESIAN_POINT('Ctrl Pts',(13.8508752065214,-23.4504857575959,1.9045506874055));
#49531=CARTESIAN_POINT('Ctrl Pts',(14.4158963288387,-23.4057058787818,2.37675373622547));
#49532=CARTESIAN_POINT('Ctrl Pts',(14.9236315787721,-23.34905257923,2.86887715082168));
#49533=CARTESIAN_POINT('Ctrl Pts',(15.169681381964,-23.3165272641956,3.11946875835517));
#49534=CARTESIAN_POINT('Ctrl Pts',(2.1,-31.2544399250396,-0.899999999999996));
#49535=CARTESIAN_POINT('Ctrl Pts',(2.73333333333333,-31.2544399250396,-0.899999999999996));
#49536=CARTESIAN_POINT('Ctrl Pts',(3.36510803949126,-31.2544285975785,-0.899887954579111));
#49537=CARTESIAN_POINT('Ctrl Pts',(4.1217599483887,-31.2544250687149,-0.899856461790129));
#49538=CARTESIAN_POINT('Ctrl Pts',(4.35078018391394,-31.2543593971872,-0.903581998407283));
#49539=CARTESIAN_POINT('Ctrl Pts',(4.83831486811687,-31.2540689041506,-0.921123484582133));
#49540=CARTESIAN_POINT('Ctrl Pts',(5.72215239235997,-31.2533869648983,-0.963543461248137));
#49541=CARTESIAN_POINT('Ctrl Pts',(6.54569204847154,-31.253375981803,-0.966087209027176));
#49542=CARTESIAN_POINT('Ctrl Pts',(7.18900601609011,-31.2545146303357,-0.882690915352525));
#49543=CARTESIAN_POINT('Ctrl Pts',(7.31714403897362,-31.2549105346497,-0.865405180349154));
#49544=CARTESIAN_POINT('Ctrl Pts',(7.58667564997587,-31.2561576889986,-0.826487518155644));
#49545=CARTESIAN_POINT('Ctrl Pts',(7.92370562146597,-31.2583919516221,-0.771819144977552));
#49546=CARTESIAN_POINT('Ctrl Pts',(8.33567742441321,-31.2616158481274,-0.693189967012442));
#49547=CARTESIAN_POINT('Ctrl Pts',(8.88879010852856,-31.265860135187,-0.567641912212619));
#49548=CARTESIAN_POINT('Ctrl Pts',(9.58533914692519,-31.2696691847387,-0.365023033156311));
#49549=CARTESIAN_POINT('Ctrl Pts',(10.1375264374995,-31.2678183104491,-0.137996175847509));
#49550=CARTESIAN_POINT('Ctrl Pts',(11.3565030519649,-31.2540818885826,0.465220229785789));
#49551=CARTESIAN_POINT('Ctrl Pts',(12.3227872766541,-31.2488724320959,1.27591572087597));
#49552=CARTESIAN_POINT('Ctrl Pts',(13.2438100919778,-31.1896995065743,2.16862824846055));
#49553=CARTESIAN_POINT('Ctrl Pts',(13.4536570645148,-31.1727762889572,2.37732774887136));
#49554=CARTESIAN_POINT('Ctrl Pts',(13.5572209116411,-31.1634652599129,2.4811657802529));
#49555=CARTESIAN_POINT('Ctrl Pts',(13.6160603594674,-31.1578938077571,2.54040820945414));
#49556=CARTESIAN_POINT('Ctrl Pts',(13.6453174194113,-31.1550264688678,2.56993362549346));
#49557=CARTESIAN_POINT('Ctrl Pts',(13.9304114081194,-31.1266303388415,2.85783766366555));
#49558=CARTESIAN_POINT('Ctrl Pts',(14.4834636188671,-31.0622526519641,3.47544368375122));
#49559=CARTESIAN_POINT('Ctrl Pts',(14.98335392639,-30.9820977609996,4.11984152156402));
#49560=CARTESIAN_POINT('Ctrl Pts',(15.2260186760796,-30.9364949201562,4.44811307850482));
#49561=CARTESIAN_POINT('Ctrl Pts',(2.1,-38.9897510790831,-0.899999999999995));
#49562=CARTESIAN_POINT('Ctrl Pts',(2.73333333333333,-38.9897510790831,-0.899999999999995));
#49563=CARTESIAN_POINT('Ctrl Pts',(3.36462990527675,-38.9897323635969,-0.899873465153036));
#49564=CARTESIAN_POINT('Ctrl Pts',(4.1208427270016,-38.9897265328331,-0.899838966037325));
#49565=CARTESIAN_POINT('Ctrl Pts',(4.34455772832346,-38.9896728108089,-0.904370340701259));
#49566=CARTESIAN_POINT('Ctrl Pts',(4.82869886846261,-38.9894393624541,-0.926010025459942));
#49567=CARTESIAN_POINT('Ctrl Pts',(5.71348591011319,-38.9888878390437,-0.979037562584771));
#49568=CARTESIAN_POINT('Ctrl Pts',(6.55581603709115,-38.988869624559,-0.983187703385992));
#49569=CARTESIAN_POINT('Ctrl Pts',(7.21830359959701,-38.9897625234554,-0.875238407743373));
#49570=CARTESIAN_POINT('Ctrl Pts',(7.3467255268605,-38.990132712043,-0.853607279018514));
#49571=CARTESIAN_POINT('Ctrl Pts',(7.61953681834974,-38.991420569913,-0.804326922325396));
#49572=CARTESIAN_POINT('Ctrl Pts',(7.96022442918569,-38.9938266042631,-0.735174920601364));
#49573=CARTESIAN_POINT('Ctrl Pts',(8.37790664744398,-38.9973035670093,-0.635391241461812));
#49574=CARTESIAN_POINT('Ctrl Pts',(8.93894152673479,-39.0017204784551,-0.475916526516923));
#49575=CARTESIAN_POINT('Ctrl Pts',(9.6458573751342,-39.0050422513425,-0.218333539006556));
#49576=CARTESIAN_POINT('Ctrl Pts',(10.2035440776973,-39.001117677713,0.0687868979514879));
#49577=CARTESIAN_POINT('Ctrl Pts',(11.4269391757474,-38.9798103474589,0.825175481853652));
#49578=CARTESIAN_POINT('Ctrl Pts',(12.379427420675,-38.968220494253,1.82168627873895));
#49579=CARTESIAN_POINT('Ctrl Pts',(13.2972499365664,-38.8888984651817,2.92824372486156));
#49580=CARTESIAN_POINT('Ctrl Pts',(13.5062198971924,-38.8664635788881,3.18711889465918));
#49581=CARTESIAN_POINT('Ctrl Pts',(13.6094926661745,-38.8541842965825,3.31604931695643));
#49582=CARTESIAN_POINT('Ctrl Pts',(13.6681658325864,-38.8468524163685,3.38962535504308));
#49583=CARTESIAN_POINT('Ctrl Pts',(13.6973582444968,-38.8430838348503,3.42631180642128));
#49584=CARTESIAN_POINT('Ctrl Pts',(13.981458935376,-38.8058099556096,3.78381873659936));
#49585=CARTESIAN_POINT('Ctrl Pts',(14.5280821792823,-38.7229860114931,4.5416971141935));
#49586=CARTESIAN_POINT('Ctrl Pts',(15.0243070371674,-38.6201388341544,5.33756918640965));
#49587=CARTESIAN_POINT('Ctrl Pts',(15.2656150130537,-38.5618298130439,5.74340641366416));
#49588=CARTESIAN_POINT('',(3.2,-37.5892271801377,-0.900000000000009));
#49589=CARTESIAN_POINT('Ctrl Pts',(3.19846504060563,-37.5892155742874,-0.899918216107268));
#49590=CARTESIAN_POINT('Ctrl Pts',(3.06435898455936,-37.9029407045989,-0.899932532575135));
#49591=CARTESIAN_POINT('Ctrl Pts',(2.93025577717209,-38.216607400202,-0.899947286012378));
#49592=CARTESIAN_POINT('Ctrl Pts',(2.79626085549373,-38.5299117979594,-0.89996027252497));
#49593=CARTESIAN_POINT('',(15.,-15.6990456112299,1.77537689056849));
#49594=CARTESIAN_POINT('Ctrl Pts',(15.,-15.6990456112299,1.77537689056849));
#49595=CARTESIAN_POINT('Ctrl Pts',(14.4897165779516,-16.2849589337065,1.51421724761149));
#49596=CARTESIAN_POINT('Ctrl Pts',(13.9833803026614,-16.8928254585971,1.26139925814643));
#49597=CARTESIAN_POINT('Ctrl Pts',(13.4460287676664,-17.5732796520164,1.02322986490673));
#49598=CARTESIAN_POINT('Ctrl Pts',(12.828265568108,-18.355560025857,0.749419748395156));
#49599=CARTESIAN_POINT('Ctrl Pts',(12.155541408957,-19.2651912004079,0.431967913798082));
#49600=CARTESIAN_POINT('Ctrl Pts',(11.5904908073729,-20.0758271479682,0.194165150923072));
#49601=CARTESIAN_POINT('Ctrl Pts',(11.1143368259691,-20.7589297458909,-0.00622527785325226));
#49602=CARTESIAN_POINT('Ctrl Pts',(10.6953158949622,-21.3919930406842,-0.162474098896682));
#49603=CARTESIAN_POINT('Ctrl Pts',(10.2957959918397,-22.0215958519058,-0.285400301904625));
#49604=CARTESIAN_POINT('Ctrl Pts',(10.0450888109335,-22.4166849192045,-0.362539091673938));
#49605=CARTESIAN_POINT('Ctrl Pts',(9.80235305580163,-22.8103758783969,-0.427399680658795));
#49606=CARTESIAN_POINT('Ctrl Pts',(9.56010106231365,-23.2148468084221,-0.485388811488509));
#49607=CARTESIAN_POINT('Ctrl Pts',(9.36613602937194,-23.5386964335034,-0.531819239200157));
#49608=CARTESIAN_POINT('Ctrl Pts',(9.15248571290285,-23.9017725603612,-0.578857851041087));
#49609=CARTESIAN_POINT('Ctrl Pts',(8.89022359818963,-24.3643567925319,-0.629224074447282));
#49610=CARTESIAN_POINT('Ctrl Pts',(8.39222406101306,-25.2427403660727,-0.724862577069152));
#49611=CARTESIAN_POINT('Ctrl Pts',(7.76643777371613,-26.4044500016645,-0.817180074306374));
#49612=CARTESIAN_POINT('Ctrl Pts',(7.10363554123529,-27.7707039763826,-0.894013240725695));
#49613=CARTESIAN_POINT('Ctrl Pts',(6.23550018249052,-29.5602172374331,-0.994648973713817));
#49614=CARTESIAN_POINT('Ctrl Pts',(5.31040885823351,-31.7028345140282,-0.937721664108877));
#49615=CARTESIAN_POINT('Ctrl Pts',(4.46416616905172,-33.9628693235812,-0.909003245197519));
#49616=CARTESIAN_POINT('Ctrl Pts',(4.30741751125037,-34.3814932331411,-0.903683762174411));
#49617=CARTESIAN_POINT('Ctrl Pts',(4.15262292089316,-34.8053728589431,-0.899999999999994));
#49618=CARTESIAN_POINT('Ctrl Pts',(4.,-35.2340925362767,-0.899999999999994));
#49619=CARTESIAN_POINT('Ctrl Pts',(3.72434973283394,-36.0083975548465,-0.899999999999995));
#49620=CARTESIAN_POINT('Ctrl Pts',(3.45587123478811,-36.7989959013664,-0.899999999999995));
#49621=CARTESIAN_POINT('Ctrl Pts',(3.2,-37.5892271801377,-0.899999999999995));
#49622=CARTESIAN_POINT('',(15.,-30.3301605390585,4.05479489924437));
#49623=CARTESIAN_POINT('Ctrl Pts',(15.,-30.3301605390585,4.05479489924437));
#49624=CARTESIAN_POINT('Ctrl Pts',(15.,-25.9658737968045,3.39120490592858));
#49625=CARTESIAN_POINT('Ctrl Pts',(15.,-20.7866378565132,2.59413270773475));
#49626=CARTESIAN_POINT('Ctrl Pts',(15.,-15.6990456112299,1.77537689056849));
#49627=CARTESIAN_POINT('Ctrl Pts',(6.,-38.9878978038234,-0.97150647893904));
#49628=CARTESIAN_POINT('Ctrl Pts',(6.38595465246567,-38.4511580946401,-0.970712640298574));
#49629=CARTESIAN_POINT('Ctrl Pts',(6.77023648668261,-37.9485848088862,-0.946911108705782));
#49630=CARTESIAN_POINT('Ctrl Pts',(7.13915213286207,-37.4906963516412,-0.889177532284711));
#49631=CARTESIAN_POINT('Ctrl Pts',(8.10667920093238,-36.2898270441738,-0.737764062830719));
#49632=CARTESIAN_POINT('Ctrl Pts',(8.98019888747373,-35.389539750921,-0.506506391035769));
#49633=CARTESIAN_POINT('Ctrl Pts',(9.46656009721079,-34.9110454673415,-0.333331441085477));
#49634=CARTESIAN_POINT('Ctrl Pts',(9.65648624874915,-34.7241913844214,-0.265705875706425));
#49635=CARTESIAN_POINT('Ctrl Pts',(9.79228848853734,-34.5946295139584,-0.211763607435485));
#49636=CARTESIAN_POINT('Ctrl Pts',(9.94593825727822,-34.4503982837665,-0.146089247346362));
#49637=CARTESIAN_POINT('Ctrl Pts',(10.1065740866009,-34.2996092297643,-0.0774288426831876));
#49638=CARTESIAN_POINT('Ctrl Pts',(10.2660951669675,-34.1533235936857,-0.00297951038240219));
#49639=CARTESIAN_POINT('Ctrl Pts',(10.4261869573617,-34.0095357957359,0.0794327468215139));
#49640=CARTESIAN_POINT('Ctrl Pts',(10.8065549509411,-33.6679050595643,0.275239070442707));
#49641=CARTESIAN_POINT('Ctrl Pts',(11.1894211925257,-33.3406313554732,0.517069342042946));
#49642=CARTESIAN_POINT('Ctrl Pts',(11.6023503255242,-33.0003063200243,0.822996043177648));
#49643=CARTESIAN_POINT('Ctrl Pts',(11.7531893954247,-32.8759888337811,0.934748146309273));
#49644=CARTESIAN_POINT('Ctrl Pts',(11.9080270687775,-32.7499870988422,1.05519161239494));
#49645=CARTESIAN_POINT('Ctrl Pts',(12.0681766131679,-32.621092353582,1.18544337126706));
#49646=CARTESIAN_POINT('Ctrl Pts',(12.1838435903475,-32.5279989538141,1.27951686537783));
#49647=CARTESIAN_POINT('Ctrl Pts',(12.3100865410161,-32.4268183073742,1.38378769072677));
#49648=CARTESIAN_POINT('Ctrl Pts',(12.5127093730713,-32.2665490637521,1.56015391817218));
#49649=CARTESIAN_POINT('Ctrl Pts',(12.7975492664043,-32.041248322494,1.80808322062817));
#49650=CARTESIAN_POINT('Ctrl Pts',(13.1874566943567,-31.7365390294451,2.16619278329376));
#49651=CARTESIAN_POINT('Ctrl Pts',(13.6431584568239,-31.3858069581634,2.5980913893376));
#49652=CARTESIAN_POINT('Ctrl Pts',(14.069523646534,-31.057653857987,3.00218579113323));
#49653=CARTESIAN_POINT('Ctrl Pts',(14.53311408767,-30.7006478334489,3.5004679889341));
#49654=CARTESIAN_POINT('Ctrl Pts',(15.,-30.3301605390585,4.05479489924437));
#49655=CARTESIAN_POINT('Origin',(15.,-7.65823537717056,3.68801178249925));
#49656=CARTESIAN_POINT('',(15.,-15.2928725900315,3.96737244938058));
#49657=CARTESIAN_POINT('Ctrl Pts',(15.,-15.2928725900315,3.96737244938057));
#49658=CARTESIAN_POINT('Ctrl Pts',(15.,-15.3032674728402,3.92730370856767));
#49659=CARTESIAN_POINT('Ctrl Pts',(15.,-15.3135058702623,3.88719029713218));
#49660=CARTESIAN_POINT('Ctrl Pts',(15.,-15.4950281428345,3.16414676313573));
#49661=CARTESIAN_POINT('Ctrl Pts',(15.,-15.62026181147,2.47203486354725));
#49662=CARTESIAN_POINT('Ctrl Pts',(15.,-15.6990456112299,1.77537689056849));
#49663=CARTESIAN_POINT('',(15.,-29.7607187491733,7.11755713237394));
#49664=CARTESIAN_POINT('Ctrl Pts',(15.,-15.2928725900315,3.96737244938059));
#49665=CARTESIAN_POINT('Ctrl Pts',(15.,-20.4763230842092,5.06462647823764));
#49666=CARTESIAN_POINT('Ctrl Pts',(15.,-25.6935126383795,6.2146953165994));
#49667=CARTESIAN_POINT('Ctrl Pts',(15.,-29.7607187491733,7.11755713237393));
#49668=CARTESIAN_POINT('Origin',(15.,0.,0.));
#49669=CARTESIAN_POINT('Ctrl Pts',(15.,-27.569647357814,13.2768424169973));
#49670=CARTESIAN_POINT('Ctrl Pts',(15.,-40.8464897748113,-14.2928049408167));
#49671=CARTESIAN_POINT('Ctrl Pts',(15.,-13.2768424169973,-27.569647357814));
#49672=CARTESIAN_POINT('Ctrl Pts',(15.,14.2928049408167,-40.8464897748113));
#49673=CARTESIAN_POINT('Ctrl Pts',(15.,27.569647357814,-13.2768424169973));
#49674=CARTESIAN_POINT('Ctrl Pts',(15.,40.8464897748113,14.2928049408167));
#49675=CARTESIAN_POINT('Ctrl Pts',(15.,13.2768424169973,27.569647357814));
#49676=CARTESIAN_POINT('Ctrl Pts',(15.,-14.2928049408167,40.8464897748113));
#49677=CARTESIAN_POINT('Ctrl Pts',(15.,-27.569647357814,13.2768424169973));
#49678=CARTESIAN_POINT('Ctrl Pts',(14.7843073131059,-27.6919221166174,13.3357268373578));
#49679=CARTESIAN_POINT('Ctrl Pts',(14.7843073131059,-41.0276489539752,-14.3561952792596));
#49680=CARTESIAN_POINT('Ctrl Pts',(14.7843073131059,-13.3357268373578,-27.6919221166174));
#49681=CARTESIAN_POINT('Ctrl Pts',(14.7843073131059,14.3561952792596,-41.0276489539752));
#49682=CARTESIAN_POINT('Ctrl Pts',(14.7843073131059,27.6919221166174,-13.3357268373578));
#49683=CARTESIAN_POINT('Ctrl Pts',(14.7843073131059,41.0276489539752,14.3561952792596));
#49684=CARTESIAN_POINT('Ctrl Pts',(14.7843073131059,13.3357268373578,27.6919221166174));
#49685=CARTESIAN_POINT('Ctrl Pts',(14.7843073131059,-14.3561952792596,41.0276489539752));
#49686=CARTESIAN_POINT('Ctrl Pts',(14.7843073131059,-27.6919221166174,13.3357268373578));
#49687=CARTESIAN_POINT('Ctrl Pts',(14.3560298066371,-27.9390044129707,13.4547154000382));
#49688=CARTESIAN_POINT('Ctrl Pts',(14.3560298066371,-41.3937198130089,-14.4842890129324));
#49689=CARTESIAN_POINT('Ctrl Pts',(14.3560298066371,-13.4547154000382,-27.9390044129707));
#49690=CARTESIAN_POINT('Ctrl Pts',(14.3560298066371,14.4842890129324,-41.3937198130089));
#49691=CARTESIAN_POINT('Ctrl Pts',(14.3560298066371,27.9390044129707,-13.4547154000382));
#49692=CARTESIAN_POINT('Ctrl Pts',(14.3560298066371,41.3937198130089,14.4842890129324));
#49693=CARTESIAN_POINT('Ctrl Pts',(14.3560298066371,13.4547154000382,27.9390044129707));
#49694=CARTESIAN_POINT('Ctrl Pts',(14.3560298066371,-14.4842890129324,41.3937198130089));
#49695=CARTESIAN_POINT('Ctrl Pts',(14.3560298066371,-27.9390044129707,13.4547154000382));
#49696=CARTESIAN_POINT('Ctrl Pts',(13.722936818686,-28.3172259246361,13.6368572803433));
#49697=CARTESIAN_POINT('Ctrl Pts',(13.722936818686,-41.9540832049794,-14.6803686442928));
#49698=CARTESIAN_POINT('Ctrl Pts',(13.722936818686,-13.6368572803433,-28.3172259246361));
#49699=CARTESIAN_POINT('Ctrl Pts',(13.722936818686,14.6803686442928,-41.9540832049794));
#49700=CARTESIAN_POINT('Ctrl Pts',(13.722936818686,28.3172259246361,-13.6368572803433));
#49701=CARTESIAN_POINT('Ctrl Pts',(13.722936818686,41.9540832049794,14.6803686442928));
#49702=CARTESIAN_POINT('Ctrl Pts',(13.722936818686,13.6368572803433,28.3172259246361));
#49703=CARTESIAN_POINT('Ctrl Pts',(13.722936818686,-14.6803686442928,41.9540832049794));
#49704=CARTESIAN_POINT('Ctrl Pts',(13.722936818686,-28.3172259246361,13.6368572803433));
#49705=CARTESIAN_POINT('Ctrl Pts',(12.8977690042853,-28.8369697397467,13.8871527099828));
#49706=CARTESIAN_POINT('Ctrl Pts',(12.8977690042853,-42.7241224497295,-14.9498170297639));
#49707=CARTESIAN_POINT('Ctrl Pts',(12.8977690042853,-13.8871527099828,-28.8369697397467));
#49708=CARTESIAN_POINT('Ctrl Pts',(12.8977690042853,14.9498170297639,-42.7241224497295));
#49709=CARTESIAN_POINT('Ctrl Pts',(12.8977690042853,28.8369697397467,-13.8871527099828));
#49710=CARTESIAN_POINT('Ctrl Pts',(12.8977690042853,42.7241224497295,14.9498170297639));
#49711=CARTESIAN_POINT('Ctrl Pts',(12.8977690042853,13.8871527099828,28.8369697397467));
#49712=CARTESIAN_POINT('Ctrl Pts',(12.8977690042853,-14.9498170297639,42.7241224497295));
#49713=CARTESIAN_POINT('Ctrl Pts',(12.8977690042853,-28.8369697397467,13.8871527099828));
#49714=CARTESIAN_POINT('Ctrl Pts',(11.9000549946031,-29.5141508562392,14.2132659480213));
#49715=CARTESIAN_POINT('Ctrl Pts',(11.9000549946031,-43.7274168042605,-15.3008849082179));
#49716=CARTESIAN_POINT('Ctrl Pts',(11.9000549946031,-14.2132659480213,-29.5141508562392));
#49717=CARTESIAN_POINT('Ctrl Pts',(11.9000549946031,15.3008849082179,-43.7274168042605));
#49718=CARTESIAN_POINT('Ctrl Pts',(11.9000549946031,29.5141508562392,-14.2132659480213));
#49719=CARTESIAN_POINT('Ctrl Pts',(11.9000549946031,43.7274168042605,15.3008849082179));
#49720=CARTESIAN_POINT('Ctrl Pts',(11.9000549946031,14.2132659480213,29.5141508562392));
#49721=CARTESIAN_POINT('Ctrl Pts',(11.9000549946031,-15.3008849082179,43.7274168042605));
#49722=CARTESIAN_POINT('Ctrl Pts',(11.9000549946031,-29.5141508562392,14.2132659480213));
#49723=CARTESIAN_POINT('Ctrl Pts',(10.9391333834985,-30.2213162016529,14.5538188296728));
#49724=CARTESIAN_POINT('Ctrl Pts',(10.9391333834985,-44.7751350313257,-15.6674973719801));
#49725=CARTESIAN_POINT('Ctrl Pts',(10.9391333834985,-14.5538188296728,-30.2213162016529));
#49726=CARTESIAN_POINT('Ctrl Pts',(10.9391333834985,15.6674973719801,-44.7751350313257));
#49727=CARTESIAN_POINT('Ctrl Pts',(10.9391333834985,30.2213162016529,-14.5538188296728));
#49728=CARTESIAN_POINT('Ctrl Pts',(10.9391333834985,44.7751350313257,15.6674973719801));
#49729=CARTESIAN_POINT('Ctrl Pts',(10.9391333834985,14.5538188296728,30.2213162016529));
#49730=CARTESIAN_POINT('Ctrl Pts',(10.9391333834985,-15.6674973719801,44.7751350313257));
#49731=CARTESIAN_POINT('Ctrl Pts',(10.9391333834985,-30.2213162016529,14.5538188296728));
#49732=CARTESIAN_POINT('Ctrl Pts',(10.0180552497783,-30.9609522745316,14.9100087895256));
#49733=CARTESIAN_POINT('Ctrl Pts',(10.0180552497783,-45.8709610640572,-16.0509434850059));
#49734=CARTESIAN_POINT('Ctrl Pts',(10.0180552497783,-14.9100087895256,-30.9609522745316));
#49735=CARTESIAN_POINT('Ctrl Pts',(10.0180552497783,16.0509434850059,-45.8709610640572));
#49736=CARTESIAN_POINT('Ctrl Pts',(10.0180552497783,30.9609522745316,-14.9100087895256));
#49737=CARTESIAN_POINT('Ctrl Pts',(10.0180552497783,45.8709610640572,16.0509434850059));
#49738=CARTESIAN_POINT('Ctrl Pts',(10.0180552497783,14.9100087895256,30.9609522745316));
#49739=CARTESIAN_POINT('Ctrl Pts',(10.0180552497783,-16.0509434850059,45.8709610640572));
#49740=CARTESIAN_POINT('Ctrl Pts',(10.0180552497783,-30.9609522745316,14.9100087895256));
#49741=CARTESIAN_POINT('Ctrl Pts',(9.13857394886632,-31.734487984447,15.2825239541622));
#49742=CARTESIAN_POINT('Ctrl Pts',(9.13857394886632,-47.0170119386091,-16.4519640302848));
#49743=CARTESIAN_POINT('Ctrl Pts',(9.13857394886632,-15.2825239541622,-31.734487984447));
#49744=CARTESIAN_POINT('Ctrl Pts',(9.13857394886632,16.4519640302848,-47.0170119386091));
#49745=CARTESIAN_POINT('Ctrl Pts',(9.13857394886632,31.734487984447,-15.2825239541622));
#49746=CARTESIAN_POINT('Ctrl Pts',(9.13857394886632,47.0170119386091,16.4519640302848));
#49747=CARTESIAN_POINT('Ctrl Pts',(9.13857394886632,15.2825239541622,31.734487984447));
#49748=CARTESIAN_POINT('Ctrl Pts',(9.13857394886632,-16.4519640302848,47.0170119386091));
#49749=CARTESIAN_POINT('Ctrl Pts',(9.13857394886632,-31.734487984447,15.2825239541622));
#49750=CARTESIAN_POINT('Ctrl Pts',(8.29915429043693,-32.5406722170424,15.6707618186629));
#49751=CARTESIAN_POINT('Ctrl Pts',(8.29915429043693,-48.2114340357053,-16.8699103983794));
#49752=CARTESIAN_POINT('Ctrl Pts',(8.29915429043693,-15.6707618186629,-32.5406722170424));
#49753=CARTESIAN_POINT('Ctrl Pts',(8.29915429043693,16.8699103983794,-48.2114340357053));
#49754=CARTESIAN_POINT('Ctrl Pts',(8.29915429043693,32.5406722170424,-15.6707618186629));
#49755=CARTESIAN_POINT('Ctrl Pts',(8.29915429043693,48.2114340357053,16.8699103983794));
#49756=CARTESIAN_POINT('Ctrl Pts',(8.29915429043693,15.6707618186629,32.5406722170424));
#49757=CARTESIAN_POINT('Ctrl Pts',(8.29915429043693,-16.8699103983794,48.2114340357053));
#49758=CARTESIAN_POINT('Ctrl Pts',(8.29915429043693,-32.5406722170424,15.6707618186629));
#49759=CARTESIAN_POINT('Ctrl Pts',(7.4968190344241,-33.3770786491896,16.0735539273924));
#49760=CARTESIAN_POINT('Ctrl Pts',(7.4968190344241,-49.450632576582,-17.3035247217972));
#49761=CARTESIAN_POINT('Ctrl Pts',(7.4968190344241,-16.0735539273924,-33.3770786491896));
#49762=CARTESIAN_POINT('Ctrl Pts',(7.4968190344241,17.3035247217972,-49.450632576582));
#49763=CARTESIAN_POINT('Ctrl Pts',(7.4968190344241,33.3770786491896,-16.0735539273924));
#49764=CARTESIAN_POINT('Ctrl Pts',(7.4968190344241,49.450632576582,17.3035247217972));
#49765=CARTESIAN_POINT('Ctrl Pts',(7.4968190344241,16.0735539273924,33.3770786491896));
#49766=CARTESIAN_POINT('Ctrl Pts',(7.4968190344241,-17.3035247217972,49.450632576582));
#49767=CARTESIAN_POINT('Ctrl Pts',(7.4968190344241,-33.3770786491896,16.0735539273924));
#49768=CARTESIAN_POINT('Ctrl Pts',(6.88220761950379,-34.0684169111937,16.4064848873841));
#49769=CARTESIAN_POINT('Ctrl Pts',(6.88220761950379,-50.4749017985778,-17.6619320238096));
#49770=CARTESIAN_POINT('Ctrl Pts',(6.88220761950379,-16.4064848873841,-34.0684169111937));
#49771=CARTESIAN_POINT('Ctrl Pts',(6.88220761950379,17.6619320238096,-50.4749017985778));
#49772=CARTESIAN_POINT('Ctrl Pts',(6.88220761950379,34.0684169111937,-16.4064848873841));
#49773=CARTESIAN_POINT('Ctrl Pts',(6.88220761950379,50.4749017985778,17.6619320238096));
#49774=CARTESIAN_POINT('Ctrl Pts',(6.88220761950379,16.4064848873841,34.0684169111937));
#49775=CARTESIAN_POINT('Ctrl Pts',(6.88220761950379,-17.6619320238096,50.4749017985778));
#49776=CARTESIAN_POINT('Ctrl Pts',(6.88220761950379,-34.0684169111937,16.4064848873841));
#49777=CARTESIAN_POINT('Ctrl Pts',(6.43560997955544,-34.5986241433973,16.6618192331215));
#49778=CARTESIAN_POINT('Ctrl Pts',(6.43560997955544,-51.2604433765188,-17.9368049102758));
#49779=CARTESIAN_POINT('Ctrl Pts',(6.43560997955544,-16.6618192331215,-34.5986241433973));
#49780=CARTESIAN_POINT('Ctrl Pts',(6.43560997955544,17.9368049102758,-51.2604433765188));
#49781=CARTESIAN_POINT('Ctrl Pts',(6.43560997955544,34.5986241433973,-16.6618192331215));
#49782=CARTESIAN_POINT('Ctrl Pts',(6.43560997955544,51.2604433765188,17.9368049102758));
#49783=CARTESIAN_POINT('Ctrl Pts',(6.43560997955544,16.6618192331215,34.5986241433973));
#49784=CARTESIAN_POINT('Ctrl Pts',(6.43560997955544,-17.9368049102758,51.2604433765188));
#49785=CARTESIAN_POINT('Ctrl Pts',(6.43560997955544,-34.5986241433973,16.6618192331215));
#49786=CARTESIAN_POINT('Ctrl Pts',(6.14415685965718,-34.9572124542593,16.8345062622337));
#49787=CARTESIAN_POINT('Ctrl Pts',(6.14415685965718,-51.791718716493,-18.1227061920256));
#49788=CARTESIAN_POINT('Ctrl Pts',(6.14415685965718,-16.8345062622337,-34.9572124542593));
#49789=CARTESIAN_POINT('Ctrl Pts',(6.14415685965718,18.1227061920256,-51.791718716493));
#49790=CARTESIAN_POINT('Ctrl Pts',(6.14415685965718,34.9572124542593,-16.8345062622337));
#49791=CARTESIAN_POINT('Ctrl Pts',(6.14415685965718,51.791718716493,18.1227061920256));
#49792=CARTESIAN_POINT('Ctrl Pts',(6.14415685965718,16.8345062622337,34.9572124542593));
#49793=CARTESIAN_POINT('Ctrl Pts',(6.14415685965718,-18.1227061920256,51.791718716493));
#49794=CARTESIAN_POINT('Ctrl Pts',(6.14415685965718,-34.9572124542593,16.8345062622337));
#49795=CARTESIAN_POINT('Ctrl Pts',(6.,-35.1377858481943,16.9214658255848));
#49796=CARTESIAN_POINT('Ctrl Pts',(6.,-52.0592516737791,-18.2163200226096));
#49797=CARTESIAN_POINT('Ctrl Pts',(6.,-16.9214658255848,-35.1377858481943));
#49798=CARTESIAN_POINT('Ctrl Pts',(6.,18.2163200226096,-52.0592516737791));
#49799=CARTESIAN_POINT('Ctrl Pts',(6.,35.1377858481943,-16.9214658255848));
#49800=CARTESIAN_POINT('Ctrl Pts',(6.,52.0592516737791,18.2163200226096));
#49801=CARTESIAN_POINT('Ctrl Pts',(6.,16.9214658255848,35.1377858481943));
#49802=CARTESIAN_POINT('Ctrl Pts',(6.,-18.2163200226096,52.0592516737791));
#49803=CARTESIAN_POINT('Ctrl Pts',(6.,-35.1377858481943,16.9214658255848));
#49804=CARTESIAN_POINT('Ctrl Pts',(15.,-29.7607187491733,7.11755713237394));
#49805=CARTESIAN_POINT('Ctrl Pts',(14.0108432136945,-30.7138276143533,5.80807302883452));
#49806=CARTESIAN_POINT('Ctrl Pts',(13.3692319443824,-31.2880423397517,4.92456278175723));
#49807=CARTESIAN_POINT('Ctrl Pts',(12.3476991724842,-32.1885965077159,3.9369824968736));
#49808=CARTESIAN_POINT('Ctrl Pts',(12.025018705019,-32.473062408263,3.62502689764848));
#49809=CARTESIAN_POINT('Ctrl Pts',(11.6666317570709,-32.7930634119362,3.28263944738858));
#49810=CARTESIAN_POINT('Ctrl Pts',(11.3593868751764,-33.0719731108646,3.0063009153141));
#49811=CARTESIAN_POINT('Ctrl Pts',(10.676771680913,-33.6916351769729,2.39235128793105));
#49812=CARTESIAN_POINT('Ctrl Pts',(10.1321636914396,-34.2060779331065,1.97784197265519));
#49813=CARTESIAN_POINT('Ctrl Pts',(9.56604173138329,-34.7743315804091,1.68073241792726));
#49814=CARTESIAN_POINT('Ctrl Pts',(9.34563078589188,-34.9955724657979,1.56505734701922));
#49815=CARTESIAN_POINT('Ctrl Pts',(9.12222951098695,-35.2252615616749,1.46777773062118));
#49816=CARTESIAN_POINT('Ctrl Pts',(8.88860711505279,-35.4734017321514,1.38109570926743));
#49817=CARTESIAN_POINT('Ctrl Pts',(8.75830600700743,-35.6118000181306,1.33274947351874));
#49818=CARTESIAN_POINT('Ctrl Pts',(8.62340343546551,-35.7561157762934,1.28545226594596));
#49819=CARTESIAN_POINT('Ctrl Pts',(8.40819516300419,-35.994889345564,1.22197488938494));
#49820=CARTESIAN_POINT('Ctrl Pts',(8.0244300682913,-36.4206767020539,1.10878034927987));
#49821=CARTESIAN_POINT('Ctrl Pts',(7.46417034513342,-37.0680247070473,0.984484082043485));
#49822=CARTESIAN_POINT('Ctrl Pts',(6.85957019142019,-37.843480699196,0.88897664134793));
#49823=CARTESIAN_POINT('Ctrl Pts',(6.58024553736738,-38.2017405762566,0.844852301206911));
#49824=CARTESIAN_POINT('Ctrl Pts',(6.28976782192772,-38.5882317623753,0.829056343619504));
#49825=CARTESIAN_POINT('Ctrl Pts',(6.,-38.9911990462069,0.828490759799981));
#49826=CARTESIAN_POINT('Ctrl Pts',(2.09999999999999,-15.7813123397985,0.900000000000003));
#49827=CARTESIAN_POINT('Ctrl Pts',(2.73333333333332,-15.7813123397985,0.900000000000003));
#49828=CARTESIAN_POINT('Ctrl Pts',(3.36803860157905,-15.7813180616194,0.899953654229283));
#49829=CARTESIAN_POINT('Ctrl Pts',(4.25277800527128,-15.7813208936813,0.899924760368668));
#49830=CARTESIAN_POINT('Ctrl Pts',(4.77267831987932,-15.7818921151941,0.891519719936119));
#49831=CARTESIAN_POINT('Ctrl Pts',(5.76857910493608,-15.7835993122471,0.867147114519683));
#49832=CARTESIAN_POINT('Ctrl Pts',(6.48509785298667,-15.7836071130985,0.867805461117988));
#49833=CARTESIAN_POINT('Ctrl Pts',(6.99867669895435,-15.7810493145741,0.901608701736404));
#49834=CARTESIAN_POINT('Ctrl Pts',(7.12481601332274,-15.7805124139621,0.910184915185508));
#49835=CARTESIAN_POINT('Ctrl Pts',(7.37171888970191,-15.7795536904041,0.928255643534913));
#49836=CARTESIAN_POINT('Ctrl Pts',(7.68212706220351,-15.7784608126719,0.95364774366657));
#49837=CARTESIAN_POINT('Ctrl Pts',(8.05075476794032,-15.7769500570881,0.98932824296244));
#49838=CARTESIAN_POINT('Ctrl Pts',(8.4150539939394,-15.7748901547651,1.03111723775223));
#49839=CARTESIAN_POINT('Ctrl Pts',(9.01076228194079,-15.7699352805976,1.11250789981985));
#49840=CARTESIAN_POINT('Ctrl Pts',(9.46311166877534,-15.7626389942107,1.19806894000414));
#49841=CARTESIAN_POINT('Ctrl Pts',(10.2678611694051,-15.7401422438828,1.39809158506708));
#49842=CARTESIAN_POINT('Ctrl Pts',(10.9805041482584,-15.7177390832667,1.65102715488742));
#49843=CARTESIAN_POINT('Ctrl Pts',(11.7910350621702,-15.6753561835242,2.018832180911));
#49844=CARTESIAN_POINT('Ctrl Pts',(12.2471627654155,-15.6444015292051,2.24062830476412));
#49845=CARTESIAN_POINT('Ctrl Pts',(12.4732580281126,-15.6263203413021,2.35401357536145));
#49846=CARTESIAN_POINT('Ctrl Pts',(12.8351268106022,-15.5948338653055,2.53703642714019));
#49847=CARTESIAN_POINT('Ctrl Pts',(13.2802529432254,-15.5503636458461,2.78452402958302));
#49848=CARTESIAN_POINT('Ctrl Pts',(14.1612575904519,-15.4429889615419,3.34567779498745));
#49849=CARTESIAN_POINT('Ctrl Pts',(14.7820737708942,-15.3388270460161,3.80399343913107));
#49850=CARTESIAN_POINT('Ctrl Pts',(15.1979896574214,-15.2534284724017,4.11495301335945));
#49851=CARTESIAN_POINT('Ctrl Pts',(2.09999999999999,-23.5174523402227,0.900000000000004));
#49852=CARTESIAN_POINT('Ctrl Pts',(2.73333333333332,-23.5174523402227,0.900000000000004));
#49853=CARTESIAN_POINT('Ctrl Pts',(3.3687269008229,-23.5174503117464,0.899999549356805));
#49854=CARTESIAN_POINT('Ctrl Pts',(4.25416629436656,-23.5174495574097,0.899986128047576));
#49855=CARTESIAN_POINT('Ctrl Pts',(4.78311339604061,-23.5180672355084,0.887379402076836));
#49856=CARTESIAN_POINT('Ctrl Pts',(5.77495354160743,-23.5199279942482,0.851096896517873));
#49857=CARTESIAN_POINT('Ctrl Pts',(6.47498972136719,-23.5199204649197,0.85254775775783));
#49858=CARTESIAN_POINT('Ctrl Pts',(6.96729289121827,-23.5171313867364,0.901565775281088));
#49859=CARTESIAN_POINT('Ctrl Pts',(7.09311090714753,-23.5165727443299,0.914323892311043));
#49860=CARTESIAN_POINT('Ctrl Pts',(7.3363104955997,-23.5156659563351,0.940991080822883));
#49861=CARTESIAN_POINT('Ctrl Pts',(7.64238643469451,-23.5147669843648,0.978505552682822));
#49862=CARTESIAN_POINT('Ctrl Pts',(8.00394198529363,-23.5135608591914,1.0310088470534));
#49863=CARTESIAN_POINT('Ctrl Pts',(8.36003532842669,-23.51172134836,1.09241611183573));
#49864=CARTESIAN_POINT('Ctrl Pts',(8.93970255550973,-23.5067933041018,1.21153595067129));
#49865=CARTESIAN_POINT('Ctrl Pts',(9.37531769324352,-23.4985467770246,1.33634734778052));
#49866=CARTESIAN_POINT('Ctrl Pts',(10.1434238337742,-23.4715958512647,1.62573582070569));
#49867=CARTESIAN_POINT('Ctrl Pts',(10.8343148881383,-23.4466861730614,1.9942694300716));
#49868=CARTESIAN_POINT('Ctrl Pts',(11.6347008962811,-23.3955621594738,2.53783642516313));
#49869=CARTESIAN_POINT('Ctrl Pts',(12.0872732667126,-23.3565546277241,2.86696783800558));
#49870=CARTESIAN_POINT('Ctrl Pts',(12.3122637721678,-23.3331927346526,3.03568289878328));
#49871=CARTESIAN_POINT('Ctrl Pts',(12.6726001818386,-23.2920224649212,3.30823650944636));
#49872=CARTESIAN_POINT('Ctrl Pts',(13.1110203697175,-23.2345645363005,3.67373154677588));
#49873=CARTESIAN_POINT('Ctrl Pts',(13.9921386008757,-23.093173534576,4.51098032026392));
#49874=CARTESIAN_POINT('Ctrl Pts',(14.6125773377935,-22.9522889563178,5.19806642891103));
#49875=CARTESIAN_POINT('Ctrl Pts',(15.0291266285127,-22.834727375518,5.66394619523217));
#49876=CARTESIAN_POINT('Ctrl Pts',(2.09999999999999,-31.253592340647,0.900000000000005));
#49877=CARTESIAN_POINT('Ctrl Pts',(2.73333333333333,-31.253592340647,0.900000000000005));
#49878=CARTESIAN_POINT('Ctrl Pts',(3.36946298994113,-31.253597129858,0.899967083396557));
#49879=CARTESIAN_POINT('Ctrl Pts',(4.25563250306681,-31.2535998064671,0.899927315911795));
#49880=CARTESIAN_POINT('Ctrl Pts',(4.793607610529,-31.2542714423515,0.882902120180317));
#49881=CARTESIAN_POINT('Ctrl Pts',(5.78148222806676,-31.256287669969,0.834747506040562));
#49882=CARTESIAN_POINT('Ctrl Pts',(6.46489469701572,-31.2562883708318,0.837373215514036));
#49883=CARTESIAN_POINT('Ctrl Pts',(6.93657638553836,-31.2532799135509,0.899507277096636));
#49884=CARTESIAN_POINT('Ctrl Pts',(7.0620883058075,-31.2527009610395,0.91640744616794));
#49885=CARTESIAN_POINT('Ctrl Pts',(7.30171951451256,-31.2518492172623,0.951277918119689));
#49886=CARTESIAN_POINT('Ctrl Pts',(7.60369867143904,-31.2511567052462,1.00034060541384));
#49887=CARTESIAN_POINT('Ctrl Pts',(7.95863609743802,-31.250265994518,1.06869690052304));
#49888=CARTESIAN_POINT('Ctrl Pts',(8.30734467161686,-31.2486814680989,1.14828732937022));
#49889=CARTESIAN_POINT('Ctrl Pts',(8.87313675628991,-31.2438333199221,1.30219016402905));
#49890=CARTESIAN_POINT('Ctrl Pts',(9.29621494250681,-31.2348126008038,1.46187419583854));
#49891=CARTESIAN_POINT('Ctrl Pts',(10.0463012266451,-31.203926559761,1.83186702435988));
#49892=CARTESIAN_POINT('Ctrl Pts',(10.7405413064001,-31.1770796248539,2.31584417428653));
#49893=CARTESIAN_POINT('Ctrl Pts',(11.548246551431,-31.1171997774263,3.04151994117155));
#49894=CARTESIAN_POINT('Ctrl Pts',(12.004199888209,-31.0700709489218,3.48088598485862));
#49895=CARTESIAN_POINT('Ctrl Pts',(12.2304316701899,-31.0414054563015,3.70603673720389));
#49896=CARTESIAN_POINT('Ctrl Pts',(12.5924678805365,-30.9905349539073,4.06954570137746));
#49897=CARTESIAN_POINT('Ctrl Pts',(13.0427854461794,-30.9189256840333,4.56466621801912));
#49898=CARTESIAN_POINT('Ctrl Pts',(13.9385950929121,-30.7403061321327,5.69639486896618));
#49899=CARTESIAN_POINT('Ctrl Pts',(14.5670688438605,-30.560172646277,6.62087479005202));
#49900=CARTESIAN_POINT('Ctrl Pts',(14.9853697475044,-30.4091322526247,7.24399554120779));
#49901=CARTESIAN_POINT('Ctrl Pts',(2.09999999999999,-38.9897323410713,0.900000000000005));
#49902=CARTESIAN_POINT('Ctrl Pts',(2.73333333333332,-38.9897323410713,0.900000000000005));
#49903=CARTESIAN_POINT('Ctrl Pts',(3.37021439053497,-38.9897437514265,0.899948482776489));
#49904=CARTESIAN_POINT('Ctrl Pts',(4.25713776543909,-38.9897498389542,0.899888266525458));
#49905=CARTESIAN_POINT('Ctrl Pts',(4.80404692086918,-38.990474960491,0.878261830529841));
#49906=CARTESIAN_POINT('Ctrl Pts',(5.78816029898518,-38.9926471520414,0.818329038315272));
#49907=CARTESIAN_POINT('Ctrl Pts',(6.45448401595128,-38.9926543924743,0.822526832763617));
#49908=CARTESIAN_POINT('Ctrl Pts',(6.90694151240769,-38.9894292569544,0.896112921981724));
#49909=CARTESIAN_POINT('Ctrl Pts',(7.03217742077181,-38.9888307738593,0.917127783371819));
#49910=CARTESIAN_POINT('Ctrl Pts',(7.26852796949471,-38.9880361255997,0.959898627245754));
#49911=CARTESIAN_POINT('Ctrl Pts',(7.56686701397648,-38.987554172558,1.02013588655783));
#49912=CARTESIAN_POINT('Ctrl Pts',(7.91608364547376,-38.9869869932131,1.10372729413102));
#49913=CARTESIAN_POINT('Ctrl Pts',(8.25887925774823,-38.9856712995636,1.20083627874114));
#49914=CARTESIAN_POINT('Ctrl Pts',(8.8143057136887,-38.9809314590746,1.38853371701586));
#49915=CARTESIAN_POINT('Ctrl Pts',(9.23056764068725,-38.9711733909723,1.58316088294249));
#49916=CARTESIAN_POINT('Ctrl Pts',(9.9765255462537,-38.9361908258605,2.04109193749097));
#49917=CARTESIAN_POINT('Ctrl Pts',(10.6790409718292,-38.9067650394502,2.6532312853716));
#49918=CARTESIAN_POINT('Ctrl Pts',(11.4921056515298,-38.8370824836761,3.56780480358298));
#49919=CARTESIAN_POINT('Ctrl Pts',(11.9504568599563,-38.7812570292348,4.119988399869));
#49920=CARTESIAN_POINT('Ctrl Pts',(12.1774856937747,-38.7470142391924,4.4023497722438));
#49921=CARTESIAN_POINT('Ctrl Pts',(12.5406836647159,-38.6860166444278,4.85788735474899));
#49922=CARTESIAN_POINT('Ctrl Pts',(12.9976779503012,-38.5991062464697,5.48794489488544));
#49923=CARTESIAN_POINT('Ctrl Pts',(13.899403431329,-38.3817347701346,6.91519011870003));
#49924=CARTESIAN_POINT('Ctrl Pts',(14.5324532885843,-38.1613150005834,8.07725552357689));
#49925=CARTESIAN_POINT('Ctrl Pts',(14.9514110803021,-37.9761728551056,8.85721942423245));
#49926=CARTESIAN_POINT('',(3.2,-37.5892271801377,0.89999999999999));
#49927=CARTESIAN_POINT('Ctrl Pts',(3.2,-37.5892271801377,0.900000000000005));
#49928=CARTESIAN_POINT('Ctrl Pts',(3.56152274835416,-36.4727023625927,0.900000000000005));
#49929=CARTESIAN_POINT('Ctrl Pts',(3.95224584525393,-35.3420203470068,0.905801001195174));
#49930=CARTESIAN_POINT('Ctrl Pts',(4.7876743012376,-33.0900361849772,0.883613319940321));
#49931=CARTESIAN_POINT('Ctrl Pts',(5.21513946232122,-32.0121842271598,0.857420319092421));
#49932=CARTESIAN_POINT('Ctrl Pts',(6.7954877540273,-28.2792370299721,0.82385346267847));
#49933=CARTESIAN_POINT('Ctrl Pts',(7.94016295939677,-26.0613850693145,1.01713589289149));
#49934=CARTESIAN_POINT('Ctrl Pts',(9.46271935276041,-23.3002380102246,1.33514989708753));
#49935=CARTESIAN_POINT('Ctrl Pts',(10.1385443659136,-22.1771939355819,1.56158379060409));
#49936=CARTESIAN_POINT('Ctrl Pts',(11.5967860400749,-19.9286553808136,2.23301757819717));
#49937=CARTESIAN_POINT('Ctrl Pts',(12.3997356677083,-18.7587345375746,2.6115335830299));
#49938=CARTESIAN_POINT('Ctrl Pts',(13.6850585208096,-16.9850659799596,3.25579646640259));
#49939=CARTESIAN_POINT('Ctrl Pts',(14.3457395898606,-16.1131272918145,3.62837109684756));
#49940=CARTESIAN_POINT('Ctrl Pts',(15.,-15.2928725900315,3.96737244938057));
#49941=CARTESIAN_POINT('Ctrl Pts',(2.79815339721959,-38.5299211738669,0.89998254368834));
#49942=CARTESIAN_POINT('Ctrl Pts',(2.93286463944684,-38.2164608351329,0.899976638205042));
#49943=CARTESIAN_POINT('Ctrl Pts',(3.06773361277345,-37.9028006789536,0.899969723070092));
#49944=CARTESIAN_POINT('Ctrl Pts',(3.20258714969926,-37.5892342471181,0.89996249608849));
#49945=CARTESIAN_POINT('Origin',(2.9,0.,0.));
#49946=CARTESIAN_POINT('',(3.2,-34.2572188230213,15.4984824583453));
#49947=CARTESIAN_POINT('Origin',(3.2,0.,0.));
#49948=CARTESIAN_POINT('Ctrl Pts',(3.19854856993727,-34.2571641451328,15.4985534066746));
#49949=CARTESIAN_POINT('Ctrl Pts',(3.06442805771908,-34.5398277577011,15.6346586929013));
#49950=CARTESIAN_POINT('Ctrl Pts',(2.93030968617731,-34.8224399543122,15.7707394686964));
#49951=CARTESIAN_POINT('Ctrl Pts',(2.7963008307409,-35.1047259901887,15.9066658257295));
#49952=CARTESIAN_POINT('Ctrl Pts',(2.10000000000001,-10.5446976527894,11.7791447047943));
#49953=CARTESIAN_POINT('Ctrl Pts',(2.73333333333334,-10.5446976527894,11.7791447047943));
#49954=CARTESIAN_POINT('Ctrl Pts',(3.36597186493151,-10.5446228424995,11.7791929127825));
#49955=CARTESIAN_POINT('Ctrl Pts',(4.12348416497485,-10.544599841335,11.7792076131232));
#49956=CARTESIAN_POINT('Ctrl Pts',(4.36307794326233,-10.5460660330961,11.7779222515897));
#49957=CARTESIAN_POINT('Ctrl Pts',(4.85756380192522,-10.5528379728112,11.7720020900147));
#49958=CARTESIAN_POINT('Ctrl Pts',(5.73898435898537,-10.5689627252743,11.7579308551903));
#49959=CARTESIAN_POINT('Ctrl Pts',(6.5260525135352,-10.569426646963,11.7575444691643));
#49960=CARTESIAN_POINT('Ctrl Pts',(7.12756341256172,-10.5394024697514,11.7835517417896));
#49961=CARTESIAN_POINT('Ctrl Pts',(7.25505875202547,-10.5328878017875,11.7893155337016));
#49962=CARTESIAN_POINT('Ctrl Pts',(7.51731750157009,-10.5186059928894,11.8021864593304));
#49963=CARTESIAN_POINT('Ctrl Pts',(7.84588509512945,-10.4986704206583,11.8204784852481));
#49964=CARTESIAN_POINT('Ctrl Pts',(8.24416390812632,-10.4702119644218,11.8466119866418));
#49965=CARTESIAN_POINT('Ctrl Pts',(8.77646398006391,-10.4246920294427,11.8878046798892));
#49966=CARTESIAN_POINT('Ctrl Pts',(9.4411345989597,-10.3508464915215,11.9526079594429));
#49967=CARTESIAN_POINT('Ctrl Pts',(9.96388516997986,-10.26693159457,12.0222081514324));
#49968=CARTESIAN_POINT('Ctrl Pts',(11.1189136052353,-10.0417705507235,12.2032651710146));
#49969=CARTESIAN_POINT('Ctrl Pts',(12.080454797577,-9.73217262268696,12.461784447063));
#49970=CARTESIAN_POINT('Ctrl Pts',(13.0008419744711,-9.36882675367162,12.7304564924823));
#49971=CARTESIAN_POINT('Ctrl Pts',(13.2108186458783,-9.28294322582199,12.7920469879376));
#49972=CARTESIAN_POINT('Ctrl Pts',(13.3144418038317,-9.23989237192285,12.8223813622727));
#49973=CARTESIAN_POINT('Ctrl Pts',(13.3733216886662,-9.21525036961191,12.8395866023987));
#49974=CARTESIAN_POINT('Ctrl Pts',(13.4026009224713,-9.20293900388632,12.8481288210721));
#49975=CARTESIAN_POINT('Ctrl Pts',(13.6877921880979,-9.08273430560209,12.9312335785886));
#49976=CARTESIAN_POINT('Ctrl Pts',(14.2465854854714,-8.82185938319892,13.1087324358622));
#49977=CARTESIAN_POINT('Ctrl Pts',(14.7537307590314,-8.54348998776827,13.2903258258105));
#49978=CARTESIAN_POINT('Ctrl Pts',(14.9999999999997,-8.40014929121784,13.3809374892743));
#49979=CARTESIAN_POINT('Ctrl Pts',(2.10000000000001,-15.3675852715397,17.8268544917116));
#49980=CARTESIAN_POINT('Ctrl Pts',(2.73333333333334,-15.3675852715397,17.8268544917116));
#49981=CARTESIAN_POINT('Ctrl Pts',(3.36558673280158,-15.3675309972709,17.8268931877247));
#49982=CARTESIAN_POINT('Ctrl Pts',(4.12268323605138,-15.3675155744444,17.8269040940857));
#49983=CARTESIAN_POINT('Ctrl Pts',(4.35699688852519,-15.3697095936867,17.8250550840541));
#49984=CARTESIAN_POINT('Ctrl Pts',(4.84800076874878,-15.3799128467904,17.8164742582301));
#49985=CARTESIAN_POINT('Ctrl Pts',(5.73068676826158,-15.4043424369138,17.7959526739925));
#49986=CARTESIAN_POINT('Ctrl Pts',(6.53594823423175,-15.4054106862613,17.7950986738855));
#49987=CARTESIAN_POINT('Ctrl Pts',(7.1587012295895,-15.3589748828166,17.8338974101007));
#49988=CARTESIAN_POINT('Ctrl Pts',(7.28652620235657,-15.349099382339,17.8423111652112));
#49989=CARTESIAN_POINT('Ctrl Pts',(7.55249020735376,-15.3272888912512,17.8612448875003));
#49990=CARTESIAN_POINT('Ctrl Pts',(7.88541634569422,-15.296871309982,17.8881352701714));
#49991=CARTESIAN_POINT('Ctrl Pts',(8.29077087410829,-15.2532979369236,17.9266727888899));
#49992=CARTESIAN_POINT('Ctrl Pts',(8.83404175048086,-15.1835241926749,17.9875016868031));
#49993=CARTESIAN_POINT('Ctrl Pts',(9.51598698571077,-15.0699838270507,18.0834946709078));
#49994=CARTESIAN_POINT('Ctrl Pts',(10.0563081198985,-14.9404974117035,18.1870277549497));
#49995=CARTESIAN_POINT('Ctrl Pts',(11.2545362612146,-14.5920275075708,18.4572762053696));
#49996=CARTESIAN_POINT('Ctrl Pts',(12.234198837956,-14.1169082623771,18.8390235742434));
#49997=CARTESIAN_POINT('Ctrl Pts',(13.1607933780956,-13.5654020914808,19.230311654985));
#49998=CARTESIAN_POINT('Ctrl Pts',(13.3718937697732,-13.4351891537631,19.319864196407));
#49999=CARTESIAN_POINT('Ctrl Pts',(13.4759419453006,-13.3699770181973,19.3639050860963));
#50000=CARTESIAN_POINT('Ctrl Pts',(13.5350456770886,-13.3326614567115,19.3888723313051));
#50001=CARTESIAN_POINT('Ctrl Pts',(13.5644155519561,-13.3140232750371,19.4012615507239));
#50002=CARTESIAN_POINT('Ctrl Pts',(13.8509041424671,-13.1320888318584,19.5218042916467));
#50003=CARTESIAN_POINT('Ctrl Pts',(14.4159109000634,-12.7349925891042,19.7812032596373));
#50004=CARTESIAN_POINT('Ctrl Pts',(14.9236315787721,-12.3149176903677,20.0437400385662));
#50005=CARTESIAN_POINT('Ctrl Pts',(15.169681381964,-12.0987180801296,20.1745520350237));
#50006=CARTESIAN_POINT('Ctrl Pts',(2.10000000000001,-20.1904728902899,23.8745642786288));
#50007=CARTESIAN_POINT('Ctrl Pts',(2.73333333333334,-20.1904728902899,23.8745642786288));
#50008=CARTESIAN_POINT('Ctrl Pts',(3.36511712968511,-20.1903753535268,23.8746272630908));
#50009=CARTESIAN_POINT('Ctrl Pts',(4.121772800169,-20.1903476480764,23.8746447505209));
#50010=CARTESIAN_POINT('Ctrl Pts',(4.35079402756333,-20.1932192199635,23.8722707271526));
#50011=CARTESIAN_POINT('Ctrl Pts',(4.8383303920068,-20.2067520378879,23.8611070555741));
#50012=CARTESIAN_POINT('Ctrl Pts',(5.72216975316483,-20.2394914205133,23.8341259601004));
#50013=CARTESIAN_POINT('Ctrl Pts',(6.54571765172787,-20.2414694717274,23.8325340970902));
#50014=CARTESIAN_POINT('Ctrl Pts',(7.18903482077842,-20.1769761054267,23.8854220896065));
#50015=CARTESIAN_POINT('Ctrl Pts',(7.31717297311608,-20.1637083631821,23.8965091360279));
#50016=CARTESIAN_POINT('Ctrl Pts',(7.58670489366458,-20.1340587603168,23.9217490624975));
#50017=CARTESIAN_POINT('Ctrl Pts',(7.9237359471977,-20.0927097147463,23.9575814811403));
#50018=CARTESIAN_POINT('Ctrl Pts',(8.33570803507908,-20.033244865644,24.0091266187489));
#50019=CARTESIAN_POINT('Ctrl Pts',(8.88882165089384,-19.9377329009591,24.0907234000965));
#50020=CARTESIAN_POINT('Ctrl Pts',(9.58537164389797,-19.7816931867799,24.220032764451));
#50021=CARTESIAN_POINT('Ctrl Pts',(10.1375595094415,-19.6030413696372,24.3601352854168));
#50022=CARTESIAN_POINT('Ctrl Pts',(11.3565368036444,-19.1228605744218,24.7254965438271));
#50023=CARTESIAN_POINT('Ctrl Pts',(12.3228216885107,-18.4857791115471,25.2268877754026));
#50024=CARTESIAN_POINT('Ctrl Pts',(13.2438406910188,-17.750936776662,25.7372203191382));
#50025=CARTESIAN_POINT('Ctrl Pts',(13.4536869673219,-17.5772178337914,25.8541109862439));
#50026=CARTESIAN_POINT('Ctrl Pts',(13.5572505985671,-17.4902288030533,25.9115731915362));
#50027=CARTESIAN_POINT('Ctrl Pts',(13.6160898983384,-17.4404375643633,25.9441542389479));
#50028=CARTESIAN_POINT('Ctrl Pts',(13.6453470368304,-17.4155658515524,25.9603212957986));
#50029=CARTESIAN_POINT('Ctrl Pts',(13.9304355722608,-17.172772609941,26.1176229975696));
#50030=CARTESIAN_POINT('Ctrl Pts',(14.4834756840846,-16.6497787408563,26.4523558285942));
#50031=CARTESIAN_POINT('Ctrl Pts',(14.98335392639,-16.0960001898358,26.7914585964211));
#50032=CARTESIAN_POINT('Ctrl Pts',(15.2260186760796,-15.8109142456191,26.9604788277526));
#50033=CARTESIAN_POINT('Ctrl Pts',(2.10000000000001,-25.0133605090401,29.9222740655461));
#50034=CARTESIAN_POINT('Ctrl Pts',(2.73333333333334,-25.0133605090401,29.9222740655461));
#50035=CARTESIAN_POINT('Ctrl Pts',(3.3646388685928,-25.0132463360064,29.922340718268));
#50036=CARTESIAN_POINT('Ctrl Pts',(4.12085565775573,-25.013214625916,29.9223584112847));
#50037=CARTESIAN_POINT('Ctrl Pts',(4.34457171221109,-25.0167236229088,29.9194913308185));
#50038=CARTESIAN_POINT('Ctrl Pts',(4.82871450329817,-25.033495966797,29.9058171622753));
#50039=CARTESIAN_POINT('Ctrl Pts',(5.71350326403012,-25.0746098135769,29.8723244268729));
#50040=CARTESIAN_POINT('Ctrl Pts',(6.55584056634621,-25.0778382570217,29.869726006846));
#50041=CARTESIAN_POINT('Ctrl Pts',(7.21833096387863,-24.9939949679208,29.9377306666232));
#50042=CARTESIAN_POINT('Ctrl Pts',(7.346753012671,-24.9773138147238,29.9515069240579));
#50043=CARTESIAN_POINT('Ctrl Pts',(7.61956458160806,-24.939587672514,29.9832397322665));
#50044=CARTESIAN_POINT('Ctrl Pts',(7.96025303539806,-24.8870218547869,30.0282369104503));
#50045=CARTESIAN_POINT('Ctrl Pts',(8.37793548706869,-24.8111754981506,30.0931695423523));
#50046=CARTESIAN_POINT('Ctrl Pts',(8.93897086621509,-24.689246172225,30.196054236466));
#50047=CARTESIAN_POINT('Ctrl Pts',(9.64588723426547,-24.4899298952911,30.3592522311079));
#50048=CARTESIAN_POINT('Ctrl Pts',(10.203573833095,-24.2630022112468,30.5352010907534));
#50049=CARTESIAN_POINT('Ctrl Pts',(11.4269679031769,-23.6583467725441,30.990143976638));
#50050=CARTESIAN_POINT('Ctrl Pts',(12.3794536276398,-22.8720122911001,31.6023997058208));
#50051=CARTESIAN_POINT('Ctrl Pts',(13.2972732213526,-21.957416724469,32.2303091018155));
#50052=CARTESIAN_POINT('Ctrl Pts',(13.5062425804685,-21.7410324541202,32.3741745574719));
#50053=CARTESIAN_POINT('Ctrl Pts',(13.6095151823004,-21.6325747352925,32.4449609360363));
#50054=CARTESIAN_POINT('Ctrl Pts',(13.6681882314017,-21.570479426627,32.485102482123));
#50055=CARTESIAN_POINT('Ctrl Pts',(13.6973807045977,-21.5394470731678,32.5050297522711));
#50056=CARTESIAN_POINT('Ctrl Pts',(13.9814771447632,-21.2367010730438,32.6987871955309));
#50057=CARTESIAN_POINT('Ctrl Pts',(14.5280907883129,-20.5925372303219,33.1065563793246));
#50058=CARTESIAN_POINT('Ctrl Pts',(15.0243070371674,-19.9061830796774,33.5223603522699));
#50059=CARTESIAN_POINT('Ctrl Pts',(15.2656150130537,-19.5525316786335,33.7298078962616));
#50060=CARTESIAN_POINT('',(3.2,-24.1401481407882,28.8273003894017));
#50061=CARTESIAN_POINT('Ctrl Pts',(3.198471221358,-24.1400746652962,28.8273438520674));
#50062=CARTESIAN_POINT('Ctrl Pts',(3.06436400315688,-24.3356906767046,29.0726148396917));
#50063=CARTESIAN_POINT('Ctrl Pts',(2.93025965397856,-24.531270609612,29.3178398607618));
#50064=CARTESIAN_POINT('Ctrl Pts',(2.79626375401858,-24.726623224287,29.5627827604819));
#50065=CARTESIAN_POINT('',(15.,-8.40014929122428,13.3809374892862));
#50066=CARTESIAN_POINT('Ctrl Pts',(15.,-8.40014929122428,13.3809374892862));
#50067=CARTESIAN_POINT('Ctrl Pts',(14.4897165779514,-8.96964310337579,13.6761925967553));
#50068=CARTESIAN_POINT('Ctrl Pts',(13.983380302661,-9.54630274603464,13.9938123448954));
#50069=CARTESIAN_POINT('Ctrl Pts',(13.4460287676664,-10.1567673260582,14.3773166678879));
#50070=CARTESIAN_POINT('Ctrl Pts',(12.828265568102,-10.858584530656,14.8182102769869));
#50071=CARTESIAN_POINT('Ctrl Pts',(12.1555414089414,-11.6739241299084,15.3314605852401));
#50072=CARTESIAN_POINT('Ctrl Pts',(11.5904908073485,-12.3652690628769,15.8169736923657));
#50073=CARTESIAN_POINT('Ctrl Pts',(11.1143368259563,-12.9478481122936,16.2261034204366));
#50074=CARTESIAN_POINT('Ctrl Pts',(10.6953158949566,-13.4647168679094,16.6236326882214));
#50075=CARTESIAN_POINT('Ctrl Pts',(10.2957959918397,-13.9533753754527,17.0392327535223));
#50076=CARTESIAN_POINT('Ctrl Pts',(10.0450888109516,-14.2600189140784,17.3000305759477));
#50077=CARTESIAN_POINT('Ctrl Pts',(9.80235305583622,-14.5561912626385,17.5673906464135));
#50078=CARTESIAN_POINT('Ctrl Pts',(9.56010106236485,-14.8537124907605,17.8474631215382));
#50079=CARTESIAN_POINT('Ctrl Pts',(9.36613602944513,-15.0919301994367,18.0717100558112));
#50080=CARTESIAN_POINT('Ctrl Pts',(9.15248571301987,-15.3550807294054,18.3262463074901));
#50081=CARTESIAN_POINT('Ctrl Pts',(8.89022359835155,-15.6828751797185,18.6565063967794));
#50082=CARTESIAN_POINT('Ctrl Pts',(8.39222406115036,-16.3053115722546,19.2836246972252));
#50083=CARTESIAN_POINT('Ctrl Pts',(7.76643777378863,-17.1018024085652,20.1343268458305));
#50084=CARTESIAN_POINT('Ctrl Pts',(7.10363554123529,-18.0137184170549,21.1546025207168));
#50085=CARTESIAN_POINT('Ctrl Pts',(6.23550018248797,-19.2081418699258,22.4909549732834));
#50086=CARTESIAN_POINT('Ctrl Pts',(5.31040885822886,-20.4995343283109,24.2016142119962));
#50087=CARTESIAN_POINT('Ctrl Pts',(4.46416616904574,-21.8861900198845,25.9864862188989));
#50088=CARTESIAN_POINT('Ctrl Pts',(4.30741751124639,-22.1430388190083,26.3170962141187));
#50089=CARTESIAN_POINT('Ctrl Pts',(4.15262292089116,-22.4044433616665,26.6507954384915));
#50090=CARTESIAN_POINT('Ctrl Pts',(4.,-22.6717457083367,26.9859819793801));
#50091=CARTESIAN_POINT('Ctrl Pts',(3.72434973283383,-23.1545169909432,27.5913580199313));
#50092=CARTESIAN_POINT('Ctrl Pts',(3.45587123478797,-23.6474469973648,28.2094726972278));
#50093=CARTESIAN_POINT('Ctrl Pts',(3.2,-24.1401481407882,28.8273003894017));
#50094=CARTESIAN_POINT('',(15.,-15.7403794776611,26.2411976460531));
#50095=CARTESIAN_POINT('Ctrl Pts',(15.,-15.7403794776611,26.2411976460531));
#50096=CARTESIAN_POINT('Ctrl Pts',(15.,-13.5381067497035,22.4153192789932));
#50097=CARTESIAN_POINT('Ctrl Pts',(15.,-10.9320820978596,17.8690631788246));
#50098=CARTESIAN_POINT('Ctrl Pts',(15.,-8.40014929122428,13.3809374892862));
#50099=CARTESIAN_POINT('Ctrl Pts',(6.,-25.0681110272506,29.8762415562171));
#50100=CARTESIAN_POINT('Ctrl Pts',(6.38595465246566,-24.7328386442811,29.4570965039835));
#50101=CARTESIAN_POINT('Ctrl Pts',(6.77023648668261,-24.4008805391967,29.0790088991504));
#50102=CARTESIAN_POINT('Ctrl Pts',(7.13915213286206,-24.0702538280742,28.757013583941));
#50103=CARTESIAN_POINT('Ctrl Pts',(8.10667920093243,-23.2031442442141,27.9125409071019));
#50104=CARTESIAN_POINT('Ctrl Pts',(8.98019888747383,-22.4610197697564,27.3528547579367));
#50105=CARTESIAN_POINT('Ctrl Pts',(9.46656009721086,-22.027289835851,27.0867256780847));
#50106=CARTESIAN_POINT('Ctrl Pts',(9.65648624874925,-21.8579164246816,26.9828011237888));
#50107=CARTESIAN_POINT('Ctrl Pts',(9.79228848853746,-21.7349621561682,26.9151380286895));
#50108=CARTESIAN_POINT('Ctrl Pts',(9.94593825727838,-21.5936891727254,26.8433208059295));
#50109=CARTESIAN_POINT('Ctrl Pts',(10.106574086601,-21.4459928693584,26.768238238398));
#50110=CARTESIAN_POINT('Ctrl Pts',(10.2660951669676,-21.2965784352636,26.7002859221237));
#50111=CARTESIAN_POINT('Ctrl Pts',(10.4261869573617,-21.1424957123869,26.6392512968066));
#50112=CARTESIAN_POINT('Ctrl Pts',(10.8065549509411,-20.7764048841091,26.4942368778062));
#50113=CARTESIAN_POINT('Ctrl Pts',(11.1894211925257,-20.3832825474409,26.3891427006873));
#50114=CARTESIAN_POINT('Ctrl Pts',(11.6023503255242,-19.9319102322466,26.3138080519751));
#50115=CARTESIAN_POINT('Ctrl Pts',(11.7531893954247,-19.7670282349209,26.2862890240476));
#50116=CARTESIAN_POINT('Ctrl Pts',(11.9080270687775,-19.5943009445266,26.2628721736317));
#50117=CARTESIAN_POINT('Ctrl Pts',(12.0681766131679,-19.4121014596106,26.2433088471935));
#50118=CARTESIAN_POINT('Ctrl Pts',(12.1838435903474,-19.2805090548735,26.2291793606483));
#50119=CARTESIAN_POINT('Ctrl Pts',(12.3100865410161,-19.135901739712,26.2150849420816));
#50120=CARTESIAN_POINT('Ctrl Pts',(12.5127093730712,-18.8980868317012,26.1997439459511));
#50121=CARTESIAN_POINT('Ctrl Pts',(12.7975492664042,-18.5637751830891,26.1781781250753));
#50122=CARTESIAN_POINT('Ctrl Pts',(13.1874566943566,-18.0938107160767,26.1632244670392));
#50123=CARTESIAN_POINT('Ctrl Pts',(13.6431584568239,-17.5374609190085,26.1582954681053));
#50124=CARTESIAN_POINT('Ctrl Pts',(14.069523646534,-17.0169270823873,26.1536837818257));
#50125=CARTESIAN_POINT('Ctrl Pts',(14.53311408767,-16.4047647574916,26.1852391011876));
#50126=CARTESIAN_POINT('Ctrl Pts',(15.,-15.7403794776611,26.2411976460531));
#50127=CARTESIAN_POINT('Origin',(15.,-1.89142793862867,8.2868872535455));
#50128=CARTESIAN_POINT('',(15.,-6.43313341740755,14.4300655106231));
#50129=CARTESIAN_POINT('Ctrl Pts',(15.,-6.43313341740755,14.4300655106231));
#50130=CARTESIAN_POINT('Ctrl Pts',(15.,-7.09235331145211,14.1361756785447));
#50131=CARTESIAN_POINT('Ctrl Pts',(15.,-7.73147565640373,13.7970939349841));
#50132=CARTESIAN_POINT('Ctrl Pts',(15.,-8.36396313002149,13.4036029817217));
#50133=CARTESIAN_POINT('Ctrl Pts',(15.,-8.38206859073762,13.3922880081493));
#50134=CARTESIAN_POINT('Ctrl Pts',(15.,-8.40014929122428,13.3809374892862));
#50135=CARTESIAN_POINT('',(15.,-12.9907743917407,27.7055911451623));
#50136=CARTESIAN_POINT('Ctrl Pts',(15.,-6.43313341740754,14.4300655106231));
#50137=CARTESIAN_POINT('Ctrl Pts',(15.,-8.80709419494161,19.1667769918265));
#50138=CARTESIAN_POINT('Ctrl Pts',(15.,-11.1607986514941,23.9627962274343));
#50139=CARTESIAN_POINT('Ctrl Pts',(15.,-12.9907743917407,27.7055911451623));
#50140=CARTESIAN_POINT('Origin',(15.,0.,0.));
#50141=CARTESIAN_POINT('Ctrl Pts',(15.,-6.80914057906322,29.8327941127638));
#50142=CARTESIAN_POINT('Ctrl Pts',(15.,-36.641934691827,23.0236535337006));
#50143=CARTESIAN_POINT('Ctrl Pts',(15.,-29.8327941127638,-6.80914057906322));
#50144=CARTESIAN_POINT('Ctrl Pts',(15.,-23.0236535337006,-36.641934691827));
#50145=CARTESIAN_POINT('Ctrl Pts',(15.,6.80914057906322,-29.8327941127638));
#50146=CARTESIAN_POINT('Ctrl Pts',(15.,36.641934691827,-23.0236535337006));
#50147=CARTESIAN_POINT('Ctrl Pts',(15.,29.8327941127638,6.80914057906322));
#50148=CARTESIAN_POINT('Ctrl Pts',(15.,23.0236535337006,36.641934691827));
#50149=CARTESIAN_POINT('Ctrl Pts',(15.,-6.80914057906322,29.8327941127638));
#50150=CARTESIAN_POINT('Ctrl Pts',(14.7843073131059,-6.83933995053713,29.9651062042906));
#50151=CARTESIAN_POINT('Ctrl Pts',(14.7843073131059,-36.8044461548278,23.1257662537535));
#50152=CARTESIAN_POINT('Ctrl Pts',(14.7843073131059,-29.9651062042906,-6.83933995053713));
#50153=CARTESIAN_POINT('Ctrl Pts',(14.7843073131059,-23.1257662537535,-36.8044461548278));
#50154=CARTESIAN_POINT('Ctrl Pts',(14.7843073131059,6.83933995053713,-29.9651062042906));
#50155=CARTESIAN_POINT('Ctrl Pts',(14.7843073131059,36.8044461548278,-23.1257662537535));
#50156=CARTESIAN_POINT('Ctrl Pts',(14.7843073131059,29.9651062042906,6.83933995053713));
#50157=CARTESIAN_POINT('Ctrl Pts',(14.7843073131059,23.1257662537535,36.8044461548278));
#50158=CARTESIAN_POINT('Ctrl Pts',(14.7843073131059,-6.83933995053713,29.9651062042906));
#50159=CARTESIAN_POINT('Ctrl Pts',(14.3560298066371,-6.90036423817605,30.2324710777091));
#50160=CARTESIAN_POINT('Ctrl Pts',(14.3560298066371,-37.1328353158852,23.3321068395331));
#50161=CARTESIAN_POINT('Ctrl Pts',(14.3560298066371,-30.2324710777091,-6.90036423817605));
#50162=CARTESIAN_POINT('Ctrl Pts',(14.3560298066371,-23.3321068395331,-37.1328353158852));
#50163=CARTESIAN_POINT('Ctrl Pts',(14.3560298066371,6.90036423817605,-30.2324710777091));
#50164=CARTESIAN_POINT('Ctrl Pts',(14.3560298066371,37.1328353158852,-23.3321068395331));
#50165=CARTESIAN_POINT('Ctrl Pts',(14.3560298066371,30.2324710777091,6.90036423817605));
#50166=CARTESIAN_POINT('Ctrl Pts',(14.3560298066371,23.3321068395331,37.1328353158852));
#50167=CARTESIAN_POINT('Ctrl Pts',(14.3560298066371,-6.90036423817605,30.2324710777091));
#50168=CARTESIAN_POINT('Ctrl Pts',(13.722936818686,-6.9937772372446,30.6417401677374));
#50169=CARTESIAN_POINT('Ctrl Pts',(13.722936818686,-37.635517404982,23.6479629304928));
#50170=CARTESIAN_POINT('Ctrl Pts',(13.722936818686,-30.6417401677374,-6.9937772372446));
#50171=CARTESIAN_POINT('Ctrl Pts',(13.722936818686,-23.6479629304928,-37.635517404982));
#50172=CARTESIAN_POINT('Ctrl Pts',(13.722936818686,6.9937772372446,-30.6417401677374));
#50173=CARTESIAN_POINT('Ctrl Pts',(13.722936818686,37.635517404982,-23.6479629304928));
#50174=CARTESIAN_POINT('Ctrl Pts',(13.722936818686,30.6417401677374,6.9937772372446));
#50175=CARTESIAN_POINT('Ctrl Pts',(13.722936818686,23.6479629304928,37.635517404982));
#50176=CARTESIAN_POINT('Ctrl Pts',(13.722936818686,-6.9937772372446,30.6417401677374));
#50177=CARTESIAN_POINT('Ctrl Pts',(12.8977690042853,-7.12214335873523,31.204148893041));
#50178=CARTESIAN_POINT('Ctrl Pts',(12.8977690042853,-38.3262922517763,24.0820055343058));
#50179=CARTESIAN_POINT('Ctrl Pts',(12.8977690042853,-31.204148893041,-7.12214335873523));
#50180=CARTESIAN_POINT('Ctrl Pts',(12.8977690042853,-24.0820055343058,-38.3262922517763));
#50181=CARTESIAN_POINT('Ctrl Pts',(12.8977690042853,7.12214335873523,-31.204148893041));
#50182=CARTESIAN_POINT('Ctrl Pts',(12.8977690042853,38.3262922517763,-24.0820055343058));
#50183=CARTESIAN_POINT('Ctrl Pts',(12.8977690042853,31.204148893041,7.12214335873523));
#50184=CARTESIAN_POINT('Ctrl Pts',(12.8977690042853,24.0820055343058,38.3262922517763));
#50185=CARTESIAN_POINT('Ctrl Pts',(12.8977690042853,-7.12214335873523,31.204148893041));
#50186=CARTESIAN_POINT('Ctrl Pts',(11.9000549946031,-7.2893932825315,31.9369186874159));
#50187=CARTESIAN_POINT('Ctrl Pts',(11.9000549946031,-39.2263119699474,24.6475254048844));
#50188=CARTESIAN_POINT('Ctrl Pts',(11.9000549946031,-31.9369186874159,-7.2893932825315));
#50189=CARTESIAN_POINT('Ctrl Pts',(11.9000549946031,-24.6475254048844,-39.2263119699474));
#50190=CARTESIAN_POINT('Ctrl Pts',(11.9000549946031,7.2893932825315,-31.9369186874159));
#50191=CARTESIAN_POINT('Ctrl Pts',(11.9000549946031,39.2263119699474,-24.6475254048844));
#50192=CARTESIAN_POINT('Ctrl Pts',(11.9000549946031,31.9369186874159,7.2893932825315));
#50193=CARTESIAN_POINT('Ctrl Pts',(11.9000549946031,24.6475254048844,39.2263119699474));
#50194=CARTESIAN_POINT('Ctrl Pts',(11.9000549946031,-7.2893932825315,31.9369186874159));
#50195=CARTESIAN_POINT('Ctrl Pts',(10.9391333834985,-7.4640486993045,32.702134066474));
#50196=CARTESIAN_POINT('Ctrl Pts',(10.9391333834985,-40.1661827657784,25.2380853671695));
#50197=CARTESIAN_POINT('Ctrl Pts',(10.9391333834985,-32.702134066474,-7.4640486993045));
#50198=CARTESIAN_POINT('Ctrl Pts',(10.9391333834985,-25.2380853671695,-40.1661827657784));
#50199=CARTESIAN_POINT('Ctrl Pts',(10.9391333834985,7.4640486993045,-32.702134066474));
#50200=CARTESIAN_POINT('Ctrl Pts',(10.9391333834985,40.1661827657784,-25.2380853671695));
#50201=CARTESIAN_POINT('Ctrl Pts',(10.9391333834985,32.702134066474,7.4640486993045));
#50202=CARTESIAN_POINT('Ctrl Pts',(10.9391333834985,25.2380853671695,40.1661827657784));
#50203=CARTESIAN_POINT('Ctrl Pts',(10.9391333834985,-7.4640486993045,32.702134066474));
#50204=CARTESIAN_POINT('Ctrl Pts',(10.0180552497783,-7.64672372347922,33.5024856413123));
#50205=CARTESIAN_POINT('Ctrl Pts',(10.0180552497783,-41.1492093647915,25.855761917833));
#50206=CARTESIAN_POINT('Ctrl Pts',(10.0180552497783,-33.5024856413123,-7.64672372347922));
#50207=CARTESIAN_POINT('Ctrl Pts',(10.0180552497783,-25.855761917833,-41.1492093647915));
#50208=CARTESIAN_POINT('Ctrl Pts',(10.0180552497783,7.64672372347922,-33.5024856413123));
#50209=CARTESIAN_POINT('Ctrl Pts',(10.0180552497783,41.1492093647915,-25.855761917833));
#50210=CARTESIAN_POINT('Ctrl Pts',(10.0180552497783,33.5024856413123,7.64672372347922));
#50211=CARTESIAN_POINT('Ctrl Pts',(10.0180552497783,25.855761917833,41.1492093647915));
#50212=CARTESIAN_POINT('Ctrl Pts',(10.0180552497783,-7.64672372347922,33.5024856413123));
#50213=CARTESIAN_POINT('Ctrl Pts',(9.13857394886632,-7.83777126657543,34.339519618326));
#50214=CARTESIAN_POINT('Ctrl Pts',(9.13857394886632,-42.1772908849014,26.5017483517505));
#50215=CARTESIAN_POINT('Ctrl Pts',(9.13857394886632,-34.339519618326,-7.83777126657543));
#50216=CARTESIAN_POINT('Ctrl Pts',(9.13857394886632,-26.5017483517505,-42.1772908849014));
#50217=CARTESIAN_POINT('Ctrl Pts',(9.13857394886632,7.83777126657543,-34.339519618326));
#50218=CARTESIAN_POINT('Ctrl Pts',(9.13857394886632,42.1772908849014,-26.5017483517505));
#50219=CARTESIAN_POINT('Ctrl Pts',(9.13857394886632,34.339519618326,7.83777126657543));
#50220=CARTESIAN_POINT('Ctrl Pts',(9.13857394886632,26.5017483517505,42.1772908849014));
#50221=CARTESIAN_POINT('Ctrl Pts',(9.13857394886632,-7.83777126657543,34.339519618326));
#50222=CARTESIAN_POINT('Ctrl Pts',(8.29915429043693,-8.03688232886511,35.21188218125));
#50223=CARTESIAN_POINT('Ctrl Pts',(8.29915429043693,-43.2487645101151,27.1749998523849));
#50224=CARTESIAN_POINT('Ctrl Pts',(8.29915429043693,-35.21188218125,-8.03688232886511));
#50225=CARTESIAN_POINT('Ctrl Pts',(8.29915429043693,-27.1749998523849,-43.2487645101151));
#50226=CARTESIAN_POINT('Ctrl Pts',(8.29915429043693,8.03688232886511,-35.21188218125));
#50227=CARTESIAN_POINT('Ctrl Pts',(8.29915429043693,43.2487645101151,-27.1749998523849));
#50228=CARTESIAN_POINT('Ctrl Pts',(8.29915429043693,35.21188218125,8.03688232886511));
#50229=CARTESIAN_POINT('Ctrl Pts',(8.29915429043693,27.1749998523849,43.2487645101151));
#50230=CARTESIAN_POINT('Ctrl Pts',(8.29915429043693,-8.03688232886511,35.21188218125));
#50231=CARTESIAN_POINT('Ctrl Pts',(7.4968190344241,-8.24345765802358,36.1169478341035));
#50232=CARTESIAN_POINT('Ctrl Pts',(7.4968190344241,-44.3604054921271,27.8734901760799));
#50233=CARTESIAN_POINT('Ctrl Pts',(7.4968190344241,-36.1169478341035,-8.24345765802358));
#50234=CARTESIAN_POINT('Ctrl Pts',(7.4968190344241,-27.8734901760799,-44.3604054921271));
#50235=CARTESIAN_POINT('Ctrl Pts',(7.4968190344241,8.24345765802358,-36.1169478341035));
#50236=CARTESIAN_POINT('Ctrl Pts',(7.4968190344241,44.3604054921271,-27.8734901760799));
#50237=CARTESIAN_POINT('Ctrl Pts',(7.4968190344241,36.1169478341035,8.24345765802358));
#50238=CARTESIAN_POINT('Ctrl Pts',(7.4968190344241,27.8734901760799,44.3604054921271));
#50239=CARTESIAN_POINT('Ctrl Pts',(7.4968190344241,-8.24345765802358,36.1169478341035));
#50240=CARTESIAN_POINT('Ctrl Pts',(6.88220761950379,-8.41420410800808,36.8650369106509));
#50241=CARTESIAN_POINT('Ctrl Pts',(6.88220761950379,-45.279241018659,28.4508328026428));
#50242=CARTESIAN_POINT('Ctrl Pts',(6.88220761950379,-36.8650369106509,-8.41420410800808));
#50243=CARTESIAN_POINT('Ctrl Pts',(6.88220761950379,-28.4508328026428,-45.279241018659));
#50244=CARTESIAN_POINT('Ctrl Pts',(6.88220761950379,8.41420410800808,-36.8650369106509));
#50245=CARTESIAN_POINT('Ctrl Pts',(6.88220761950379,45.279241018659,-28.4508328026428));
#50246=CARTESIAN_POINT('Ctrl Pts',(6.88220761950379,36.8650369106509,8.41420410800808));
#50247=CARTESIAN_POINT('Ctrl Pts',(6.88220761950379,28.4508328026428,45.279241018659));
#50248=CARTESIAN_POINT('Ctrl Pts',(6.88220761950379,-8.41420410800808,36.8650369106509));
#50249=CARTESIAN_POINT('Ctrl Pts',(6.43560997955544,-8.54515448010585,37.4387679776515));
#50250=CARTESIAN_POINT('Ctrl Pts',(6.43560997955544,-45.9839224577573,28.8936134975456));
#50251=CARTESIAN_POINT('Ctrl Pts',(6.43560997955544,-37.4387679776515,-8.54515448010585));
#50252=CARTESIAN_POINT('Ctrl Pts',(6.43560997955544,-28.8936134975456,-45.9839224577573));
#50253=CARTESIAN_POINT('Ctrl Pts',(6.43560997955544,8.54515448010585,-37.4387679776515));
#50254=CARTESIAN_POINT('Ctrl Pts',(6.43560997955544,45.9839224577573,-28.8936134975456));
#50255=CARTESIAN_POINT('Ctrl Pts',(6.43560997955544,37.4387679776515,8.54515448010585));
#50256=CARTESIAN_POINT('Ctrl Pts',(6.43560997955544,28.8936134975456,45.9839224577573));
#50257=CARTESIAN_POINT('Ctrl Pts',(6.43560997955544,-8.54515448010585,37.4387679776515));
#50258=CARTESIAN_POINT('Ctrl Pts',(6.14415685965718,-8.63371847902026,37.8267922098931));
#50259=CARTESIAN_POINT('Ctrl Pts',(6.14415685965718,-46.4605106889134,29.1930737308729));
#50260=CARTESIAN_POINT('Ctrl Pts',(6.14415685965718,-37.8267922098931,-8.63371847902026));
#50261=CARTESIAN_POINT('Ctrl Pts',(6.14415685965718,-29.1930737308729,-46.4605106889134));
#50262=CARTESIAN_POINT('Ctrl Pts',(6.14415685965718,8.63371847902026,-37.8267922098931));
#50263=CARTESIAN_POINT('Ctrl Pts',(6.14415685965718,46.4605106889134,-29.1930737308729));
#50264=CARTESIAN_POINT('Ctrl Pts',(6.14415685965718,37.8267922098931,8.63371847902026));
#50265=CARTESIAN_POINT('Ctrl Pts',(6.14415685965718,29.1930737308729,46.4605106889134));
#50266=CARTESIAN_POINT('Ctrl Pts',(6.14415685965718,-8.63371847902026,37.8267922098931));
#50267=CARTESIAN_POINT('Ctrl Pts',(6.,-8.67831642429626,38.0221885750911));
#50268=CARTESIAN_POINT('Ctrl Pts',(6.,-46.7005049993874,29.3438721507949));
#50269=CARTESIAN_POINT('Ctrl Pts',(6.,-38.0221885750911,-8.67831642429626));
#50270=CARTESIAN_POINT('Ctrl Pts',(6.,-29.3438721507949,-46.7005049993874));
#50271=CARTESIAN_POINT('Ctrl Pts',(6.,8.67831642429626,-38.0221885750911));
#50272=CARTESIAN_POINT('Ctrl Pts',(6.,46.7005049993874,-29.3438721507949));
#50273=CARTESIAN_POINT('Ctrl Pts',(6.,38.0221885750911,8.67831642429626));
#50274=CARTESIAN_POINT('Ctrl Pts',(6.,29.3438721507949,46.7005049993874));
#50275=CARTESIAN_POINT('Ctrl Pts',(6.,-8.67831642429626,38.0221885750911));
#50276=CARTESIAN_POINT('Ctrl Pts',(15.,-12.9907743917407,27.7055911451623));
#50277=CARTESIAN_POINT('Ctrl Pts',(14.0108432136945,-14.6088239471801,27.6343116779264));
#50278=CARTESIAN_POINT('Ctrl Pts',(13.3692319443824,-15.6575970987913,27.5323911990493));
#50279=CARTESIAN_POINT('Ctrl Pts',(12.3476991724842,-16.9912047967252,27.6207265630898));
#50280=CARTESIAN_POINT('Ctrl Pts',(12.0250187050191,-17.4124630932992,27.6486298250765));
#50281=CARTESIAN_POINT('Ctrl Pts',(11.6666317570709,-17.879669743489,27.6853416006481));
#50282=CARTESIAN_POINT('Ctrl Pts',(11.3593868751765,-18.2696172606052,27.731107727427));
#50283=CARTESIAN_POINT('Ctrl Pts',(10.6767716809131,-19.1359753867601,27.8327877076734));
#50284=CARTESIAN_POINT('Ctrl Pts',(10.1321636914396,-19.7808016313084,27.9765529194963));
#50285=CARTESIAN_POINT('Ctrl Pts',(9.56604173138328,-20.367391588899,28.2355867335771));
#50286=CARTESIAN_POINT('Ctrl Pts',(9.34563078589188,-20.5957714368658,28.3364375959427));
#50287=CARTESIAN_POINT('Ctrl Pts',(9.12222951098698,-20.8150365124456,28.4553629135261));
#50288=CARTESIAN_POINT('Ctrl Pts',(8.88860711505283,-21.0375201114275,28.595321354551));
#50289=CARTESIAN_POINT('Ctrl Pts',(8.75830600700746,-21.1616086404974,28.6733821067016));
#50290=CARTESIAN_POINT('Ctrl Pts',(8.62340343546554,-21.2885664898727,28.7567233832714));
#50291=CARTESIAN_POINT('Ctrl Pts',(8.40819516300422,-21.4870679866862,28.9038265799739));
#50292=CARTESIAN_POINT('Ctrl Pts',(8.02443006829132,-21.8410411163157,29.166144898733));
#50293=CARTESIAN_POINT('Ctrl Pts',(7.46417034513343,-22.3418347305613,29.5947644941187));
#50294=CARTESIAN_POINT('Ctrl Pts',(6.85957019142019,-22.899994357402,30.1414924867737));
#50295=CARTESIAN_POINT('Ctrl Pts',(6.58024553736738,-23.1578635354298,30.3940802614732));
#50296=CARTESIAN_POINT('Ctrl Pts',(6.28976782192773,-23.4111866254207,30.6864026200108));
#50297=CARTESIAN_POINT('Ctrl Pts',(6.,-23.6628748086085,31.0011024931715));
#50298=CARTESIAN_POINT('Ctrl Pts',(2.09999999999999,-9.1358389695905,12.8994676435885));
#50299=CARTESIAN_POINT('Ctrl Pts',(2.73333333333333,-9.1358389695905,12.8994676435885));
#50300=CARTESIAN_POINT('Ctrl Pts',(3.36803396034652,-9.13587946857483,12.8994427611867));
#50301=CARTESIAN_POINT('Ctrl Pts',(4.25277026443832,-9.13590413998491,12.8994267516404));
#50302=CARTESIAN_POINT('Ctrl Pts',(4.77266782207174,-9.14283195334969,12.8946326691098));
#50303=CARTESIAN_POINT('Ctrl Pts',(5.76856815409261,-9.16295171178049,12.8807712941876));
#50304=CARTESIAN_POINT('Ctrl Pts',(6.48508324968699,-9.16244277980798,12.8811872446167));
#50305=CARTESIAN_POINT('Ctrl Pts',(6.99866103340899,-9.13441989422394,12.9002632404603));
#50306=CARTESIAN_POINT('Ctrl Pts',(7.1248003053003,-9.12737999976702,12.9051906488153));
#50307=CARTESIAN_POINT('Ctrl Pts',(7.37170307579371,-9.11265400996954,12.9157079837048));
#50308=CARTESIAN_POINT('Ctrl Pts',(7.68211097020559,-9.09212039919145,12.9306851681623));
#50309=CARTESIAN_POINT('Ctrl Pts',(8.05073856781673,-9.06328234581171,12.9517504216116));
#50310=CARTESIAN_POINT('Ctrl Pts',(8.41503776200927,-9.02932619481544,12.9761948589261));
#50311=CARTESIAN_POINT('Ctrl Pts',(9.01074580667397,-8.96260310536268,13.0230672198542));
#50312=CARTESIAN_POINT('Ctrl Pts',(9.46309579122147,-8.89115997747123,13.0707089963125));
#50313=CARTESIAN_POINT('Ctrl Pts',(10.2678466003299,-8.72074990849221,13.1778321896751));
#50314=CARTESIAN_POINT('Ctrl Pts',(10.9804913088774,-8.50902906615356,13.3180193104141));
#50315=CARTESIAN_POINT('Ctrl Pts',(11.7910235970548,-8.19504180806732,13.5142059637011));
#50316=CARTESIAN_POINT('Ctrl Pts',(12.2471523736939,-8.00233437587927,13.6282924769383));
#50317=CARTESIAN_POINT('Ctrl Pts',(12.473248541207,-7.90241242624034,13.6848508114561));
#50318=CARTESIAN_POINT('Ctrl Pts',(12.835119440223,-7.73968708601252,13.7743470979446));
#50319=CARTESIAN_POINT('Ctrl Pts',(13.2802515759032,-7.51846451475199,13.893886306531));
#50320=CARTESIAN_POINT('Ctrl Pts',(14.1612566771783,-7.01278962913115,14.1598111690564));
#50321=CARTESIAN_POINT('Ctrl Pts',(14.7820737708942,-6.58952040585146,14.3641290043432));
#50322=CARTESIAN_POINT('Ctrl Pts',(15.1979896574214,-6.293157281203,14.4912418342554));
#50323=CARTESIAN_POINT('Ctrl Pts',(2.09999999999999,-13.9592433656065,18.9478254487004));
#50324=CARTESIAN_POINT('Ctrl Pts',(2.73333333333333,-13.9592433656065,18.9478254487004));
#50325=CARTESIAN_POINT('Ctrl Pts',(3.36872001028818,-13.9592430229431,18.9478231191763));
#50326=CARTESIAN_POINT('Ctrl Pts',(4.25415479043436,-13.9592533149426,18.9478139437242));
#50327=CARTESIAN_POINT('Ctrl Pts',(4.7830977821647,-13.9694950763228,18.9404364496675));
#50328=CARTESIAN_POINT('Ctrl Pts',(5.77493725537989,-13.9990220924234,18.9192694384421));
#50329=CARTESIAN_POINT('Ctrl Pts',(6.4749679303508,-13.9978840640735,18.9201673597862));
#50330=CARTESIAN_POINT('Ctrl Pts',(6.96726949180708,-13.9578216279669,18.9485487239907));
#50331=CARTESIAN_POINT('Ctrl Pts',(7.09308743961926,-13.9474986367052,18.9560665046118));
#50332=CARTESIAN_POINT('Ctrl Pts',(7.33628686896228,-13.9260840480499,18.9719842439271));
#50333=CARTESIAN_POINT('Ctrl Pts',(7.64236232313703,-13.8961937138069,18.9946711654445));
#50334=CARTESIAN_POINT('Ctrl Pts',(8.00391772282853,-13.8543929989952,19.0264634303694));
#50335=CARTESIAN_POINT('Ctrl Pts',(8.36001086452926,-13.8052361360177,19.0633119060548));
#50336=CARTESIAN_POINT('Ctrl Pts',(8.93967782036849,-13.7090318701985,19.1337290363374));
#50337=CARTESIAN_POINT('Ctrl Pts',(9.37529315599633,-13.6063093912297,19.2050998156635));
#50338=CARTESIAN_POINT('Ctrl Pts',(10.1434001221335,-13.3632536306442,19.3644588529799));
#50339=CARTESIAN_POINT('Ctrl Pts',(10.834292561854,-13.0595924539228,19.5747599519676));
#50340=CARTESIAN_POINT('Ctrl Pts',(11.6346804009544,-12.6027392234137,19.8736981509546));
#50341=CARTESIAN_POINT('Ctrl Pts',(12.0872541836183,-12.3210927384552,20.0484111755836));
#50342=CARTESIAN_POINT('Ctrl Pts',(12.312245937423,-12.1746196452708,20.1353385324134));
#50343=CARTESIAN_POINT('Ctrl Pts',(12.6725852131256,-11.9358582362001,20.2730855006835));
#50344=CARTESIAN_POINT('Ctrl Pts',(13.111014081714,-11.6142751048964,20.4560476897286));
#50345=CARTESIAN_POINT('Ctrl Pts',(13.9921333654529,-10.8715316570354,20.8675199651784));
#50346=CARTESIAN_POINT('Ctrl Pts',(14.6125773377935,-10.2465061114962,21.1857635085628));
#50347=CARTESIAN_POINT('Ctrl Pts',(15.0291266285127,-9.80896819642242,21.3843214467584));
#50348=CARTESIAN_POINT('Ctrl Pts',(2.09999999999999,-18.7826477616224,24.9961832538124));
#50349=CARTESIAN_POINT('Ctrl Pts',(2.73333333333333,-18.7826477616224,24.9961832538124));
#50350=CARTESIAN_POINT('Ctrl Pts',(3.36945492966225,-18.7826777179121,24.9961656007647));
#50351=CARTESIAN_POINT('Ctrl Pts',(4.2556188098197,-18.7827110508831,24.9961424923783));
#50352=CARTESIAN_POINT('Ctrl Pts',(4.79358899047167,-18.7964412840621,24.9860521050349));
#50353=CARTESIAN_POINT('Ctrl Pts',(5.78146281943922,-18.8353472835957,24.9576044685868));
#50354=CARTESIAN_POINT('Ctrl Pts',(6.46486945359605,-18.8332967951376,24.959240722034));
#50355=CARTESIAN_POINT('Ctrl Pts',(6.93654950905192,-18.7828433682711,24.9956280758371));
#50356=CARTESIAN_POINT('Ctrl Pts',(7.06206135947415,-18.769269337643,25.0057124981866));
#50357=CARTESIAN_POINT('Ctrl Pts',(7.30169240156151,-18.7414755139896,25.0267879160898));
#50358=CARTESIAN_POINT('Ctrl Pts',(7.60367117597197,-18.7026852581207,25.0568363852838));
#50359=CARTESIAN_POINT('Ctrl Pts',(7.95860842859181,-18.6486868578601,25.0987594126722));
#50360=CARTESIAN_POINT('Ctrl Pts',(8.30731707317219,-18.5854728780161,25.1471442340964));
#50361=CARTESIAN_POINT('Ctrl Pts',(8.87310871284282,-18.4621240372099,25.2393106240003));
#50362=CARTESIAN_POINT('Ctrl Pts',(9.29618834699587,-18.3316544025768,25.3318189029734));
#50363=CARTESIAN_POINT('Ctrl Pts',(10.0462774324726,-18.0231260796766,25.5383575274243));
#50364=CARTESIAN_POINT('Ctrl Pts',(10.7405209602188,-17.6279994974315,25.8191221563898));
#50365=CARTESIAN_POINT('Ctrl Pts',(11.5482282528203,-17.0233084556598,26.2247579066847));
#50366=CARTESIAN_POINT('Ctrl Pts',(12.0041830503694,-16.6504133177635,26.461851751404));
#50367=CARTESIAN_POINT('Ctrl Pts',(12.2304159734591,-16.456510112927,26.579819767925));
#50368=CARTESIAN_POINT('Ctrl Pts',(12.5924547381801,-16.1405885621055,26.76669275901));
#50369=CARTESIAN_POINT('Ctrl Pts',(13.0427800388235,-15.7088357620631,27.0194118197174));
#50370=CARTESIAN_POINT('Ctrl Pts',(13.9385905427776,-14.7126468494779,27.5853829514202));
#50371=CARTESIAN_POINT('Ctrl Pts',(14.5670688438605,-13.8775476356544,28.0209529954987));
#50372=CARTESIAN_POINT('Ctrl Pts',(14.9853697475044,-13.2962000699107,28.2913742942891));
#50373=CARTESIAN_POINT('Ctrl Pts',(2.09999999999999,-23.6060521576384,31.0445410589243));
#50374=CARTESIAN_POINT('Ctrl Pts',(2.73333333333333,-23.6060521576384,31.0445410589243));
#50375=CARTESIAN_POINT('Ctrl Pts',(3.37020567578152,-23.6061012377393,31.0445167170057));
#50376=CARTESIAN_POINT('Ctrl Pts',(4.25712263390388,-23.6061528913754,31.0444834021622));
#50377=CARTESIAN_POINT('Ctrl Pts',(4.80402631037446,-23.6235140941777,31.0315658657309));
#50378=CARTESIAN_POINT('Ctrl Pts',(5.78813882280503,-23.6717259268289,30.9958965701794));
#50379=CARTESIAN_POINT('Ctrl Pts',(6.45445717224562,-23.6684510662632,30.9985176925269));
#50380=CARTESIAN_POINT('Ctrl Pts',(6.90691329160007,-23.6089092172418,31.0418757119288));
#50381=CARTESIAN_POINT('Ctrl Pts',(7.03214913606668,-23.5921060187484,31.0545103301399));
#50382=CARTESIAN_POINT('Ctrl Pts',(7.26849953702799,-23.5581710572885,31.0805561729954));
#50383=CARTESIAN_POINT('Ctrl Pts',(7.56683838895087,-23.5107754859076,31.1177364790289));
#50384=CARTESIAN_POINT('Ctrl Pts',(7.91605485564789,-23.4450675478998,31.1694113667199));
#50385=CARTESIAN_POINT('Ctrl Pts',(8.25885085470307,-23.3683245653721,31.2289290660225));
#50386=CARTESIAN_POINT('Ctrl Pts',(8.81427676356264,-23.2186216887375,31.3422506346006));
#50387=CARTESIAN_POINT('Ctrl Pts',(9.230541336078,-23.0603721928338,31.4559695174958));
#50388=CARTESIAN_POINT('Ctrl Pts',(9.97650378825299,-22.6805359674084,31.7141346440069));
#50389=CARTESIAN_POINT('Ctrl Pts',(10.6790242999544,-22.1835991752983,32.0727916994504));
#50390=CARTESIAN_POINT('Ctrl Pts',(11.4920909027962,-21.4251096839784,32.5885394149958));
#50391=CARTESIAN_POINT('Ctrl Pts',(11.9504434973868,-20.9585878216415,32.8891746503978));
#50392=CARTESIAN_POINT('Ctrl Pts',(12.1774732934021,-20.7164781036866,33.0384524243975));
#50393=CARTESIAN_POINT('Ctrl Pts',(12.5406734120574,-20.3222914406926,33.2747866829337));
#50394=CARTESIAN_POINT('Ctrl Pts',(12.997674080036,-19.7755003700753,33.5996747028483));
#50395=CARTESIAN_POINT('Ctrl Pts',(13.8994000182975,-18.5241058978638,34.319599884084));
#50396=CARTESIAN_POINT('Ctrl Pts',(14.5324532885843,-17.4781380681113,34.8718039257929));
#50397=CARTESIAN_POINT('Ctrl Pts',(14.9514110803021,-16.7529034957905,35.2133535056034));
#50398=CARTESIAN_POINT('',(3.2,-22.7328514723457,29.9495820327474));
#50399=CARTESIAN_POINT('Ctrl Pts',(3.2,-22.7328514723457,29.9495820327475));
#50400=CARTESIAN_POINT('Ctrl Pts',(3.56152274835438,-22.0367096350838,29.0766477794334));
#50401=CARTESIAN_POINT('Ctrl Pts',(3.9522458452542,-21.3272055238567,28.1962618480736));
#50402=CARTESIAN_POINT('Ctrl Pts',(4.78767430123817,-19.9404633926114,26.4217559391896));
#50403=CARTESIAN_POINT('Ctrl Pts',(5.21513946232189,-19.2889122016819,25.5627262762193));
#50404=CARTESIAN_POINT('Ctrl Pts',(6.79548775402795,-16.9877013184703,22.6232620424128));
#50405=CARTESIAN_POINT('Ctrl Pts',(7.94016295939784,-15.4537789500188,21.0097851802331));
#50406=CARTESIAN_POINT('Ctrl Pts',(9.46271935276271,-13.4835985568963,19.0493119701759));
#50407=CARTESIAN_POINT('Ctrl Pts',(10.1385443659171,-12.606358882668,18.3124599798231));
#50408=CARTESIAN_POINT('Ctrl Pts',(11.5967860400763,-10.6794699511535,16.973113867352));
#50409=CARTESIAN_POINT('Ctrl Pts',(12.3997356677094,-9.65410050721625,16.2944337889661));
#50410=CARTESIAN_POINT('Ctrl Pts',(13.6850585208088,-8.0445312444617,15.3094152086593));
#50411=CARTESIAN_POINT('Ctrl Pts',(14.3457395898605,-7.20959578890565,14.8600025739989));
#50412=CARTESIAN_POINT('Ctrl Pts',(15.,-6.43313341740755,14.4300655106231));
#50413=CARTESIAN_POINT('Ctrl Pts',(2.7981505262301,-23.3193787656373,30.685034966607));
#50414=CARTESIAN_POINT('Ctrl Pts',(2.93286079301997,-23.1239442315795,30.439958005238));
#50415=CARTESIAN_POINT('Ctrl Pts',(3.06772862158681,-22.9283859253528,30.1947241748125));
#50416=CARTESIAN_POINT('Ctrl Pts',(3.20258097292904,-22.7328862936894,29.94956342958));
#50417=CARTESIAN_POINT('Origin',(2.9,0.,0.));
#50418=CARTESIAN_POINT('',(3.2,-9.24182505978395,36.4465179346992));
#50419=CARTESIAN_POINT('Origin',(3.2,0.,0.));
#50420=CARTESIAN_POINT('Ctrl Pts',(3.19857330932923,-9.24172635305947,36.4465202813748));
#50421=CARTESIAN_POINT('Ctrl Pts',(3.06444826166183,-9.31155448788265,36.7523757023571));
#50422=CARTESIAN_POINT('Ctrl Pts',(2.93032536154112,-9.38136974531151,37.0581756374017));
#50423=CARTESIAN_POINT('Ctrl Pts',(2.79631258706843,-9.45110215575605,37.3636243084515));
#50424=CARTESIAN_POINT('Ctrl Pts',(2.1,2.6347947165568,15.5883531961151));
#50425=CARTESIAN_POINT('Ctrl Pts',(2.73333333333333,2.6347947165568,15.5883531961151));
#50426=CARTESIAN_POINT('Ctrl Pts',(3.36597092855911,2.63487877694595,15.5883248523788));
#50427=CARTESIAN_POINT('Ctrl Pts',(4.12348287006708,2.63490452868168,15.5883160613212));
#50428=CARTESIAN_POINT('Ctrl Pts',(4.36307655407023,2.63298541566169,15.5886609732488));
#50429=CARTESIAN_POINT('Ctrl Pts',(4.85756224330648,2.62413456290923,15.5902643440359));
#50430=CARTESIAN_POINT('Ctrl Pts',(5.73898260168751,2.60307954294172,15.5940979332686));
#50431=CARTESIAN_POINT('Ctrl Pts',(6.52604985398505,2.60248787292251,15.5942198385231));
#50432=CARTESIAN_POINT('Ctrl Pts',(7.12756040848415,2.64154082328796,15.5869612993371));
#50433=CARTESIAN_POINT('Ctrl Pts',(7.25505573466752,2.65010896186311,15.5854615937326));
#50434=CARTESIAN_POINT('Ctrl Pts',(7.51731445119969,2.66907640732711,15.5823205204395));
#50435=CARTESIAN_POINT('Ctrl Pts',(7.84588191847868,2.69580726019365,15.5781391720899));
#50436=CARTESIAN_POINT('Ctrl Pts',(8.24416069925083,2.7339827985819,15.5721834308337));
#50437=CARTESIAN_POINT('Ctrl Pts',(8.77646064332894,2.7945696858706,15.5622777615526));
#50438=CARTESIAN_POINT('Ctrl Pts',(9.44113113319551,2.89127679751306,15.5449472038089));
#50439=CARTESIAN_POINT('Ctrl Pts',(9.96388158672623,2.99801240629933,15.5227349400434));
#50440=CARTESIAN_POINT('Ctrl Pts',(11.1189097708078,3.27995384619542,15.4595842505362));
#50441=CARTESIAN_POINT('Ctrl Pts',(12.0804504807078,3.67510301631977,15.378715156088));
#50442=CARTESIAN_POINT('Ctrl Pts',(13.0008381113228,4.11170193500177,15.2621541211597));
#50443=CARTESIAN_POINT('Ctrl Pts',(13.2108148630541,4.21340285849752,15.2334087107959));
#50444=CARTESIAN_POINT('Ctrl Pts',(13.3144380484095,4.26396100854989,15.218663366468));
#50445=CARTESIAN_POINT('Ctrl Pts',(13.3733179522989,4.2927766528207,15.2101247620612));
#50446=CARTESIAN_POINT('Ctrl Pts',(13.4025971758006,4.3071312344584,15.2058253366162));
#50447=CARTESIAN_POINT('Ctrl Pts',(13.6877891557158,4.44705188898038,15.1636603735762));
#50448=CARTESIAN_POINT('Ctrl Pts',(14.2465840714085,4.74847969800923,15.0703686144057));
#50449=CARTESIAN_POINT('Ctrl Pts',(14.7537307590314,5.06401626322089,14.9659520583603));
#50450=CARTESIAN_POINT('Ctrl Pts',(14.9999999999997,5.22423077688621,14.9103792371774));
#50451=CARTESIAN_POINT('Ctrl Pts',(2.1,4.35606337899725,23.1297239496034));
#50452=CARTESIAN_POINT('Ctrl Pts',(2.73333333333333,4.35606337899725,23.1297239496034));
#50453=CARTESIAN_POINT('Ctrl Pts',(3.36558543190671,4.35612716337005,23.1297057293561));
#50454=CARTESIAN_POINT('Ctrl Pts',(4.12268142832915,4.35614521108889,23.1297004979493));
#50455=CARTESIAN_POINT('Ctrl Pts',(4.3569949475632,4.35333162406734,23.1302630191334));
#50456=CARTESIAN_POINT('Ctrl Pts',(4.84799859005213,4.34026118051108,23.1328902028501));
#50457=CARTESIAN_POINT('Ctrl Pts',(5.73068431571993,4.30898508319672,23.1391950484359));
#50458=CARTESIAN_POINT('Ctrl Pts',(6.53594452799194,4.30765093285249,23.1394978970553));
#50459=CARTESIAN_POINT('Ctrl Pts',(7.15869704281812,4.36693709747872,23.1273835845108));
#50460=CARTESIAN_POINT('Ctrl Pts',(7.28652199655925,4.37967250394112,23.1249084995651));
#50461=CARTESIAN_POINT('Ctrl Pts',(7.55248595534259,4.40807408785084,23.1196613579342));
#50462=CARTESIAN_POINT('Ctrl Pts',(7.88541191425088,4.44806281423684,23.1126458361116));
#50463=CARTESIAN_POINT('Ctrl Pts',(8.29076639755633,4.50536019693898,23.1026065558361));
#50464=CARTESIAN_POINT('Ctrl Pts',(8.83403708716025,4.59642126151075,23.0859814745868));
#50465=CARTESIAN_POINT('Ctrl Pts',(9.51598213434279,4.74226276135199,23.0570627188072));
#50466=CARTESIAN_POINT('Ctrl Pts',(10.0563030846795,4.9039414957736,23.0203780338792));
#50467=CARTESIAN_POINT('Ctrl Pts',(11.2545308253523,5.33249726135678,22.9164305886563));
#50468=CARTESIAN_POINT('Ctrl Pts',(12.2341926884871,5.92719043165041,22.7829833102729));
#50469=CARTESIAN_POINT('Ctrl Pts',(13.1607878864896,6.5769705088875,22.5957624671674));
#50470=CARTESIAN_POINT('Ctrl Pts',(13.3718883884894,6.72817198515924,22.5497929772012));
#50471=CARTESIAN_POINT('Ctrl Pts',(13.4759366022101,6.80326365911736,22.5262671163551));
#50472=CARTESIAN_POINT('Ctrl Pts',(13.5350403600778,6.84604972260816,22.5126594542453));
#50473=CARTESIAN_POINT('Ctrl Pts',(13.5644102208465,6.86735671317708,22.5058120913436));
#50474=CARTESIAN_POINT('Ctrl Pts',(13.850899789237,7.0750356041283,22.4387270236514));
#50475=CARTESIAN_POINT('Ctrl Pts',(14.4159087057268,7.52542850338841,22.2899969175317));
#50476=CARTESIAN_POINT('Ctrl Pts',(14.9236315787721,7.99260139788206,22.1252578594855));
#50477=CARTESIAN_POINT('Ctrl Pts',(15.169681381964,8.22967258714631,22.0377861434561));
#50478=CARTESIAN_POINT('Ctrl Pts',(2.1,6.0773320414377,30.6710947030918));
#50479=CARTESIAN_POINT('Ctrl Pts',(2.73333333333333,6.0773320414377,30.6710947030918));
#50480=CARTESIAN_POINT('Ctrl Pts',(3.36511575592128,6.07744159234164,30.6710578689652));
#50481=CARTESIAN_POINT('Ctrl Pts',(4.12177085956525,6.07747238314756,30.6710471580155));
#50482=CARTESIAN_POINT('Ctrl Pts',(4.35079193747223,6.0738258616781,30.6718120759031));
#50483=CARTESIAN_POINT('Ctrl Pts',(4.83832804865265,6.05666008100118,30.6754320523652));
#50484=CARTESIAN_POINT('Ctrl Pts',(5.72216713207848,6.01515261534281,30.6842063322053));
#50485=CARTESIAN_POINT('Ctrl Pts',(6.5457137878836,6.01267406596902,30.6847605261392));
#50486=CARTESIAN_POINT('Ctrl Pts',(7.18903047452237,6.09423426265411,30.6673127811817));
#50487=CARTESIAN_POINT('Ctrl Pts',(7.31716860740305,6.11117475734039,30.6638523057514));
#50488=CARTESIAN_POINT('Ctrl Pts',(7.58670048132759,6.14939432722339,30.6564081566631));
#50489=CARTESIAN_POINT('Ctrl Pts',(7.92373137203068,6.20318983887758,30.6464213526081));
#50490=CARTESIAN_POINT('Ctrl Pts',(8.33570341698837,6.2805651510717,30.6320677369574));
#50491=CARTESIAN_POINT('Ctrl Pts',(8.88881689288255,6.40391068085729,30.608268282651));
#50492=CARTESIAN_POINT('Ctrl Pts',(9.58536674245199,6.60229784679161,30.5668946362938));
#50493=CARTESIAN_POINT('Ctrl Pts',(10.1375545224602,6.82322181666221,30.5145715779978));
#50494=CARTESIAN_POINT('Ctrl Pts',(11.3565317171601,7.40826014599771,30.3669503054083));
#50495=CARTESIAN_POINT('Ctrl Pts',(12.3228165107166,8.19747637375704,30.1814726492943));
#50496=CARTESIAN_POINT('Ctrl Pts',(13.243836087323,9.05463748545945,29.9251367893499));
#50497=CARTESIAN_POINT('Ctrl Pts',(13.4536824685161,9.25433833928729,29.862197970734));
#50498=CARTESIAN_POINT('Ctrl Pts',(13.5572461322348,9.35350089827159,29.8300142987523));
#50499=CARTESIAN_POINT('Ctrl Pts',(13.6160854542733,9.41001813369078,29.8113998859174));
#50500=CARTESIAN_POINT('Ctrl Pts',(13.6453425809554,9.43816529738583,29.8020343960706));
#50501=CARTESIAN_POINT('Ctrl Pts',(13.9304319363095,9.71252849392874,29.710286783206));
#50502=CARTESIAN_POINT('Ctrl Pts',(14.4834738667375,10.3003159989071,29.5100957209417));
#50503=CARTESIAN_POINT('Ctrl Pts',(14.98335392639,10.9107138228419,29.288560902014));
#50504=CARTESIAN_POINT('Ctrl Pts',(15.2260186760796,11.2206073397433,29.1710541261593));
#50505=CARTESIAN_POINT('Ctrl Pts',(2.1,7.79860070387815,38.2124654565801));
#50506=CARTESIAN_POINT('Ctrl Pts',(2.73333333333333,7.79860070387815,38.2124654565801));
#50507=CARTESIAN_POINT('Ctrl Pts',(3.36463751436128,7.79872338061474,38.2124179470539));
#50508=CARTESIAN_POINT('Ctrl Pts',(4.12085370601274,7.79875679292426,38.2124042468681));
#50509=CARTESIAN_POINT('Ctrl Pts',(4.34456960184645,7.79432734686382,38.2133601111439));
#50510=CARTESIAN_POINT('Ctrl Pts',(4.82871214417148,7.77317894546784,38.2179475900756));
#50511=CARTESIAN_POINT('Ctrl Pts',(5.71350064499196,7.72135905324094,38.2292093593782));
#50512=CARTESIAN_POINT('Ctrl Pts',(6.55583686528122,7.71731376425226,38.2301136297106));
#50513=CARTESIAN_POINT('Ctrl Pts',(7.21832683560861,7.82275706013742,38.2069626157521));
#50514=CARTESIAN_POINT('Ctrl Pts',(7.3467488661425,7.84392828956102,38.2025101244878));
#50515=CARTESIAN_POINT('Ctrl Pts',(7.61956039329437,7.89225983243226,38.1927997302842));
#50516=CARTESIAN_POINT('Ctrl Pts',(7.96024872021727,7.96021416603579,38.1797574416493));
#50517=CARTESIAN_POINT('Ctrl Pts',(8.37793113671827,8.05826993943243,38.1609432159692));
#50518=CARTESIAN_POINT('Ctrl Pts',(8.93896644082855,8.21472997667767,38.1297626383333));
#50519=CARTESIAN_POINT('Ctrl Pts',(9.6458827308017,8.46659482431919,38.0756832340632));
#50520=CARTESIAN_POINT('Ctrl Pts',(10.2035693459978,8.745644125101,38.0079664066119));
#50521=CARTESIAN_POINT('Ctrl Pts',(11.4269635730292,9.47832897311608,37.8188801486782));
#50522=CARTESIAN_POINT('Ctrl Pts',(12.3794496835402,10.4472805414767,37.5858346075197));
#50523=CARTESIAN_POINT('Ctrl Pts',(13.297269717393,11.5084412735018,37.2622699611218));
#50524=CARTESIAN_POINT('Ctrl Pts',(13.5062391671476,11.7558332723801,37.1827925479603));
#50525=CARTESIAN_POINT('Ctrl Pts',(13.609511794127,11.8787985987299,37.1421314651239));
#50526=CARTESIAN_POINT('Ctrl Pts',(13.668184860874,11.9488983329783,37.1186112363832));
#50527=CARTESIAN_POINT('Ctrl Pts',(13.6973773248548,11.9838264461449,37.106773618565));
#50528=CARTESIAN_POINT('Ctrl Pts',(13.9814744041932,12.3240718432943,36.9908828203732));
#50529=CARTESIAN_POINT('Ctrl Pts',(14.5280894908559,13.0445097705752,36.7414946448057));
#50530=CARTESIAN_POINT('Ctrl Pts',(15.0243070371674,13.797534545931,36.464130441338));
#50531=CARTESIAN_POINT('Ctrl Pts',(15.2656150130537,14.1802216087483,36.3169760702825));
#50532=CARTESIAN_POINT('',(3.2,7.48695481785667,36.8470556158206));
#50533=CARTESIAN_POINT('Ctrl Pts',(3.19847028779066,7.48703421002627,36.8470253949768));
#50534=CARTESIAN_POINT('Ctrl Pts',(3.06436324509112,7.55683027125151,37.1528880888971));
#50535=CARTESIAN_POINT('Ctrl Pts',(2.93025906836479,7.6266128911633,37.4586939150269));
#50536=CARTESIAN_POINT('Ctrl Pts',(2.79626331616334,7.69631666193415,37.7641461193963));
#50537=CARTESIAN_POINT('',(15.,5.22423077689144,14.9103792371898));
#50538=CARTESIAN_POINT('Ctrl Pts',(15.,5.22423077689144,14.9103792371898));
#50539=CARTESIAN_POINT('Ctrl Pts',(14.4897165779514,5.09999693117215,15.5397159770542));
#50540=CARTESIAN_POINT('Ctrl Pts',(13.9833803026614,4.98878064338043,16.1885993141875));
#50541=CARTESIAN_POINT('Ctrl Pts',(13.4460287676664,4.9079979567178,16.9049907761367));
#50542=CARTESIAN_POINT('Ctrl Pts',(12.8282655681041,4.81512659089501,17.728586230604));
#50543=CARTESIAN_POINT('Ctrl Pts',(12.155541408949,4.70804591508919,18.6860507311911));
#50544=CARTESIAN_POINT('Ctrl Pts',(11.5904908073611,4.65658883211823,19.5292784359842));
#50545=CARTESIAN_POINT('Ctrl Pts',(11.1143368259633,4.61322723784883,20.2398452909418));
#50546=CARTESIAN_POINT('Ctrl Pts',(10.6953158949599,4.60176573657917,20.8918050007962));
#50547=CARTESIAN_POINT('Ctrl Pts',(10.2957959918397,4.62202135570262,21.5329760085416));
#50548=CARTESIAN_POINT('Ctrl Pts',(10.0450888109446,4.63473218469528,21.935324363575));
#50549=CARTESIAN_POINT('Ctrl Pts',(9.8023530558227,4.6591022660215,22.3335775072864));
#50550=CARTESIAN_POINT('Ctrl Pts',(9.56010106234469,4.69257029287764,22.740811302168));
#50551=CARTESIAN_POINT('Ctrl Pts',(9.36613602941621,4.71936729395905,23.0668730831249));
#50552=CARTESIAN_POINT('Ctrl Pts',(9.15248571297353,4.75430007716532,23.4313132092381));
#50553=CARTESIAN_POINT('Ctrl Pts',(8.8902235982873,4.80813131550359,23.8935070279378));
#50554=CARTESIAN_POINT('Ctrl Pts',(8.39222406109597,4.91034940297294,24.7711492603301));
#50555=CARTESIAN_POINT('Ctrl Pts',(7.76643777375998,5.07885121123793,25.924274985688));
#50556=CARTESIAN_POINT('Ctrl Pts',(7.10363554123529,5.30796452320538,27.2733711088097));
#50557=CARTESIAN_POINT('Ctrl Pts',(6.23550018248759,5.60805610032957,29.0404110935273));
#50558=CARTESIAN_POINT('Ctrl Pts',(5.31040885822732,6.14033332093044,31.1166409635101));
#50559=CARTESIAN_POINT('Ctrl Pts',(4.46416616904365,6.67123676571769,33.3136215324547));
#50560=CARTESIAN_POINT('Ctrl Pts',(4.30741751124502,6.76957546152532,33.7205659702542));
#50561=CARTESIAN_POINT('Ctrl Pts',(4.15262292089048,6.86748895430781,34.1329983346473));
#50562=CARTESIAN_POINT('Ctrl Pts',(4.,6.96288805731186,34.5509691145741));
#50563=CARTESIAN_POINT('Ctrl Pts',(3.72434973283387,7.13518713321112,35.3058606897205));
#50564=CARTESIAN_POINT('Ctrl Pts',(3.45587123478811,7.31111181566301,36.0766370850674));
#50565=CARTESIAN_POINT('Ctrl Pts',(3.2,7.48695481785667,36.8470556158205));
#50566=CARTESIAN_POINT('',(15.,10.7022283756421,28.6674433425027));
#50567=CARTESIAN_POINT('Ctrl Pts',(15.,10.7022283756421,28.6674433425027));
#50568=CARTESIAN_POINT('Ctrl Pts',(15.,9.08413080697444,24.5602410457909));
#50569=CARTESIAN_POINT('Ctrl Pts',(15.,7.15455445431742,19.6882246137983));
#50570=CARTESIAN_POINT('Ctrl Pts',(15.,5.22423077689144,14.9103792371898));
#50571=CARTESIAN_POINT('Ctrl Pts',(6.,7.72847464911697,38.226570335278));
#50572=CARTESIAN_POINT('Ctrl Pts',(6.38595465246565,7.60981276318642,37.7031111655031));
#50573=CARTESIAN_POINT('Ctrl Pts',(6.77023648668261,7.52118446376145,37.2078421022651));
#50574=CARTESIAN_POINT('Ctrl Pts',(7.13915213286207,7.47558077173047,36.7485869352853));
#50575=CARTESIAN_POINT('Ctrl Pts',(8.10667920093242,7.35597942952432,35.5441332619163));
#50576=CARTESIAN_POINT('Ctrl Pts',(8.98019888747381,7.3811062193398,34.6149583776291));
#50577=CARTESIAN_POINT('Ctrl Pts',(9.46656009721084,7.44346431686218,34.1099258931473));
#50578=CARTESIAN_POINT('Ctrl Pts',(9.65648624874921,7.46781542308235,33.9127085282358));
#50579=CARTESIAN_POINT('Ctrl Pts',(9.79228848853741,7.49157501764555,33.7743917604516));
#50580=CARTESIAN_POINT('Ctrl Pts',(9.94593825727831,7.52350831636315,33.6191627883852));
#50581=CARTESIAN_POINT('Ctrl Pts',(10.106574086601,7.55689354020401,33.4568759534155));
#50582=CARTESIAN_POINT('Ctrl Pts',(10.2660951669676,7.59692465594275,33.2976914686953));
#50583=CARTESIAN_POINT('Ctrl Pts',(10.4261869573617,7.64527487070543,33.1391702786004));
#50584=CARTESIAN_POINT('Ctrl Pts',(10.8065549509411,7.76015193050434,32.7625339322407));
#50585=CARTESIAN_POINT('Ctrl Pts',(11.1894211925257,7.92309376200424,32.3896533653038));
#50586=CARTESIAN_POINT('Ctrl Pts',(11.6023503255242,8.14562079728536,31.9897858937717));
#50587=CARTESIAN_POINT('Ctrl Pts',(11.7531893954247,8.22690779872745,31.8437181241004));
#50588=CARTESIAN_POINT('Ctrl Pts',(11.9080270687775,8.31629347191557,31.6940743231629));
#50589=CARTESIAN_POINT('Ctrl Pts',(12.0681766131679,8.41459776815341,31.5394274952415));
#50590=CARTESIAN_POINT('Ctrl Pts',(12.1838435903474,8.48559741309695,31.4277348195979));
#50591=CARTESIAN_POINT('Ctrl Pts',(12.310086541016,8.56473913921171,31.3058885417699));
#50592=CARTESIAN_POINT('Ctrl Pts',(12.5127093730712,8.70102023533918,31.1103924050491));
#50593=CARTESIAN_POINT('Ctrl Pts',(12.7975492664042,8.89259930118548,30.8355709638236));
#50594=CARTESIAN_POINT('Ctrl Pts',(13.1874566943566,9.17392611297301,30.458814494586));
#50595=CARTESIAN_POINT('Ctrl Pts',(13.6431584568239,9.51695089116758,30.0207695274047));
#50596=CARTESIAN_POINT('Ctrl Pts',(14.069523646534,9.83789286830266,29.6109244468797));
#50597=CARTESIAN_POINT('Ctrl Pts',(14.53311408767,10.2442407770738,29.151991088712));
#50598=CARTESIAN_POINT('Ctrl Pts',(15.,10.7022283756421,28.6674433425027));
#50599=CARTESIAN_POINT('Origin',(15.,5.29966331579924,6.64556760097825));
#50600=CARTESIAN_POINT('',(15.,7.27088643053102,14.0266249226733));
#50601=CARTESIAN_POINT('Ctrl Pts',(15.,7.27088643053101,14.0266249226733));
#50602=CARTESIAN_POINT('Ctrl Pts',(15.,6.61162657474121,14.3683609829217));
#50603=CARTESIAN_POINT('Ctrl Pts',(15.,5.92779573167863,14.6638673522892));
#50604=CARTESIAN_POINT('Ctrl Pts',(15.,5.22423077689144,14.9103792371898));
#50605=CARTESIAN_POINT('',(15.,13.5614880461774,27.4307499345787));
#50606=CARTESIAN_POINT('Ctrl Pts',(15.,7.27088643053102,14.0266249226733));
#50607=CARTESIAN_POINT('Ctrl Pts',(15.,9.49405625509847,18.8359534995712));
#50608=CARTESIAN_POINT('Ctrl Pts',(15.,11.776224358769,23.666422827049));
#50609=CARTESIAN_POINT('Ctrl Pts',(15.,13.5614880461774,27.4307499345787));
#50610=CARTESIAN_POINT('Origin',(15.,0.,0.));
#50611=CARTESIAN_POINT('Ctrl Pts',(15.,19.0787879368772,23.9240433635217));
#50612=CARTESIAN_POINT('Ctrl Pts',(15.,-4.84525542664446,43.0028313003989));
#50613=CARTESIAN_POINT('Ctrl Pts',(15.,-23.9240433635217,19.0787879368772));
#50614=CARTESIAN_POINT('Ctrl Pts',(15.,-43.0028313003989,-4.84525542664446));
#50615=CARTESIAN_POINT('Ctrl Pts',(15.,-19.0787879368772,-23.9240433635217));
#50616=CARTESIAN_POINT('Ctrl Pts',(15.,4.84525542664446,-43.0028313003989));
#50617=CARTESIAN_POINT('Ctrl Pts',(15.,23.9240433635217,-19.0787879368772));
#50618=CARTESIAN_POINT('Ctrl Pts',(15.,43.0028313003989,4.84525542664446));
#50619=CARTESIAN_POINT('Ctrl Pts',(15.,19.0787879368772,23.9240433635217));
#50620=CARTESIAN_POINT('Ctrl Pts',(14.7843073131059,19.1634046954076,24.0301494226203));
#50621=CARTESIAN_POINT('Ctrl Pts',(14.7843073131059,-4.86674472721275,43.1935541180279));
#50622=CARTESIAN_POINT('Ctrl Pts',(14.7843073131059,-24.0301494226203,19.1634046954076));
#50623=CARTESIAN_POINT('Ctrl Pts',(14.7843073131059,-43.1935541180279,-4.86674472721275));
#50624=CARTESIAN_POINT('Ctrl Pts',(14.7843073131059,-19.1634046954076,-24.0301494226203));
#50625=CARTESIAN_POINT('Ctrl Pts',(14.7843073131059,4.86674472721275,-43.1935541180279));
#50626=CARTESIAN_POINT('Ctrl Pts',(14.7843073131059,24.0301494226203,-19.1634046954076));
#50627=CARTESIAN_POINT('Ctrl Pts',(14.7843073131059,43.1935541180279,4.86674472721275));
#50628=CARTESIAN_POINT('Ctrl Pts',(14.7843073131059,19.1634046954076,24.0301494226203));
#50629=CARTESIAN_POINT('Ctrl Pts',(14.3560298066371,19.3343909497437,24.2445594038433));
#50630=CARTESIAN_POINT('Ctrl Pts',(14.3560298066371,-4.91016845409963,43.578950353587));
#50631=CARTESIAN_POINT('Ctrl Pts',(14.3560298066371,-24.2445594038433,19.3343909497437));
#50632=CARTESIAN_POINT('Ctrl Pts',(14.3560298066371,-43.578950353587,-4.91016845409963));
#50633=CARTESIAN_POINT('Ctrl Pts',(14.3560298066371,-19.3343909497437,-24.2445594038433));
#50634=CARTESIAN_POINT('Ctrl Pts',(14.3560298066371,4.91016845409963,-43.578950353587));
#50635=CARTESIAN_POINT('Ctrl Pts',(14.3560298066371,24.2445594038433,-19.3343909497437));
#50636=CARTESIAN_POINT('Ctrl Pts',(14.3560298066371,43.578950353587,4.91016845409963));
#50637=CARTESIAN_POINT('Ctrl Pts',(14.3560298066371,19.3343909497437,24.2445594038433));
#50638=CARTESIAN_POINT('Ctrl Pts',(13.722936818686,19.5961283568486,24.5727677312355));
#50639=CARTESIAN_POINT('Ctrl Pts',(13.722936818686,-4.97663937438694,44.1688960880841));
#50640=CARTESIAN_POINT('Ctrl Pts',(13.722936818686,-24.5727677312355,19.5961283568486));
#50641=CARTESIAN_POINT('Ctrl Pts',(13.722936818686,-44.1688960880841,-4.97663937438694));
#50642=CARTESIAN_POINT('Ctrl Pts',(13.722936818686,-19.5961283568486,-24.5727677312355));
#50643=CARTESIAN_POINT('Ctrl Pts',(13.722936818686,4.97663937438694,-44.1688960880841));
#50644=CARTESIAN_POINT('Ctrl Pts',(13.722936818686,24.5727677312355,-19.5961283568486));
#50645=CARTESIAN_POINT('Ctrl Pts',(13.722936818686,44.1688960880841,4.97663937438694));
#50646=CARTESIAN_POINT('Ctrl Pts',(13.722936818686,19.5961283568486,24.5727677312355));
#50647=CARTESIAN_POINT('Ctrl Pts',(12.8977690042853,19.9558022366521,25.0237845110024));
#50648=CARTESIAN_POINT('Ctrl Pts',(12.8977690042853,-5.0679822743503,44.9795867476544));
#50649=CARTESIAN_POINT('Ctrl Pts',(12.8977690042853,-25.0237845110024,19.9558022366521));
#50650=CARTESIAN_POINT('Ctrl Pts',(12.8977690042853,-44.9795867476544,-5.0679822743503));
#50651=CARTESIAN_POINT('Ctrl Pts',(12.8977690042853,-19.9558022366521,-25.0237845110024));
#50652=CARTESIAN_POINT('Ctrl Pts',(12.8977690042853,5.0679822743503,-44.9795867476544));
#50653=CARTESIAN_POINT('Ctrl Pts',(12.8977690042853,25.0237845110024,-19.9558022366521));
#50654=CARTESIAN_POINT('Ctrl Pts',(12.8977690042853,44.9795867476544,5.0679822743503));
#50655=CARTESIAN_POINT('Ctrl Pts',(12.8977690042853,19.9558022366521,25.0237845110024));
#50656=CARTESIAN_POINT('Ctrl Pts',(11.9000549946031,20.4244261094473,25.6114202607695));
#50657=CARTESIAN_POINT('Ctrl Pts',(11.9000549946031,-5.18699415132218,46.0358463702168));
#50658=CARTESIAN_POINT('Ctrl Pts',(11.9000549946031,-25.6114202607695,20.4244261094473));
#50659=CARTESIAN_POINT('Ctrl Pts',(11.9000549946031,-46.0358463702168,-5.18699415132218));
#50660=CARTESIAN_POINT('Ctrl Pts',(11.9000549946031,-20.4244261094473,-25.6114202607695));
#50661=CARTESIAN_POINT('Ctrl Pts',(11.9000549946031,5.18699415132218,-46.0358463702168));
#50662=CARTESIAN_POINT('Ctrl Pts',(11.9000549946031,25.6114202607695,-20.4244261094473));
#50663=CARTESIAN_POINT('Ctrl Pts',(11.9000549946031,46.0358463702168,5.18699415132218));
#50664=CARTESIAN_POINT('Ctrl Pts',(11.9000549946031,20.4244261094473,25.6114202607695));
#50665=CARTESIAN_POINT('Ctrl Pts',(10.9391333834985,20.9137997124663,26.2250753492544));
#50666=CARTESIAN_POINT('Ctrl Pts',(10.9391333834985,-5.3112756367881,47.1388750617207));
#50667=CARTESIAN_POINT('Ctrl Pts',(10.9391333834985,-26.2250753492544,20.9137997124663));
#50668=CARTESIAN_POINT('Ctrl Pts',(10.9391333834985,-47.1388750617207,-5.3112756367881));
#50669=CARTESIAN_POINT('Ctrl Pts',(10.9391333834985,-20.9137997124663,-26.2250753492544));
#50670=CARTESIAN_POINT('Ctrl Pts',(10.9391333834985,5.3112756367881,-47.1388750617207));
#50671=CARTESIAN_POINT('Ctrl Pts',(10.9391333834985,26.2250753492544,-20.9137997124663));
#50672=CARTESIAN_POINT('Ctrl Pts',(10.9391333834985,47.1388750617207,5.3112756367881));
#50673=CARTESIAN_POINT('Ctrl Pts',(10.9391333834985,20.9137997124663,26.2250753492544));
#50674=CARTESIAN_POINT('Ctrl Pts',(10.0180552497783,21.4256437560905,26.8669074790281));
#50675=CARTESIAN_POINT('Ctrl Pts',(10.0180552497783,-5.44126372293754,48.2925512351186));
#50676=CARTESIAN_POINT('Ctrl Pts',(10.0180552497783,-26.8669074790281,21.4256437560905));
#50677=CARTESIAN_POINT('Ctrl Pts',(10.0180552497783,-48.2925512351186,-5.44126372293754));
#50678=CARTESIAN_POINT('Ctrl Pts',(10.0180552497783,-21.4256437560905,-26.8669074790281));
#50679=CARTESIAN_POINT('Ctrl Pts',(10.0180552497783,5.44126372293754,-48.2925512351186));
#50680=CARTESIAN_POINT('Ctrl Pts',(10.0180552497783,26.8669074790281,-21.4256437560905));
#50681=CARTESIAN_POINT('Ctrl Pts',(10.0180552497783,48.2925512351186,5.44126372293754));
#50682=CARTESIAN_POINT('Ctrl Pts',(10.0180552497783,21.4256437560905,26.8669074790281));
#50683=CARTESIAN_POINT('Ctrl Pts',(9.13857394886632,21.9609470764246,27.5381566113461));
#50684=CARTESIAN_POINT('Ctrl Pts',(9.13857394886632,-5.57720953492155,49.4991036877707));
#50685=CARTESIAN_POINT('Ctrl Pts',(9.13857394886632,-27.5381566113461,21.9609470764246));
#50686=CARTESIAN_POINT('Ctrl Pts',(9.13857394886632,-49.4991036877707,-5.57720953492155));
#50687=CARTESIAN_POINT('Ctrl Pts',(9.13857394886632,-21.9609470764246,-27.5381566113461));
#50688=CARTESIAN_POINT('Ctrl Pts',(9.13857394886632,5.57720953492155,-49.4991036877707));
#50689=CARTESIAN_POINT('Ctrl Pts',(9.13857394886632,27.5381566113461,-21.9609470764246));
#50690=CARTESIAN_POINT('Ctrl Pts',(9.13857394886632,49.4991036877707,5.57720953492155));
#50691=CARTESIAN_POINT('Ctrl Pts',(9.13857394886632,21.9609470764246,27.5381566113461));
#50692=CARTESIAN_POINT('Ctrl Pts',(8.29915429043693,22.5188438754702,28.2377370698584));
#50693=CARTESIAN_POINT('Ctrl Pts',(8.29915429043693,-5.71889319438813,50.7565809453286));
#50694=CARTESIAN_POINT('Ctrl Pts',(8.29915429043693,-28.2377370698584,22.5188438754702));
#50695=CARTESIAN_POINT('Ctrl Pts',(8.29915429043693,-50.7565809453286,-5.71889319438813));
#50696=CARTESIAN_POINT('Ctrl Pts',(8.29915429043693,-22.5188438754702,-28.2377370698584));
#50697=CARTESIAN_POINT('Ctrl Pts',(8.29915429043693,5.71889319438813,-50.7565809453286));
#50698=CARTESIAN_POINT('Ctrl Pts',(8.29915429043693,28.2377370698584,-22.5188438754702));
#50699=CARTESIAN_POINT('Ctrl Pts',(8.29915429043693,50.7565809453286,5.71889319438813));
#50700=CARTESIAN_POINT('Ctrl Pts',(8.29915429043693,22.5188438754702,28.2377370698584));
#50701=CARTESIAN_POINT('Ctrl Pts',(7.4968190344241,23.0976550855257,28.9635433702624));
#50702=CARTESIAN_POINT('Ctrl Pts',(7.4968190344241,-5.86588828473676,52.0611984557881));
#50703=CARTESIAN_POINT('Ctrl Pts',(7.4968190344241,-28.9635433702624,23.0976550855257));
#50704=CARTESIAN_POINT('Ctrl Pts',(7.4968190344241,-52.0611984557881,-5.86588828473676));
#50705=CARTESIAN_POINT('Ctrl Pts',(7.4968190344241,-23.0976550855257,-28.9635433702624));
#50706=CARTESIAN_POINT('Ctrl Pts',(7.4968190344241,5.86588828473676,-52.0611984557881));
#50707=CARTESIAN_POINT('Ctrl Pts',(7.4968190344241,28.9635433702624,-23.0976550855257));
#50708=CARTESIAN_POINT('Ctrl Pts',(7.4968190344241,52.0611984557881,5.86588828473676));
#50709=CARTESIAN_POINT('Ctrl Pts',(7.4968190344241,23.0976550855257,28.9635433702624));
#50710=CARTESIAN_POINT('Ctrl Pts',(6.88220761950379,23.5760760069919,29.5634642304892));
#50711=CARTESIAN_POINT('Ctrl Pts',(6.88220761950379,-5.98738822349723,53.1395402374811));
#50712=CARTESIAN_POINT('Ctrl Pts',(6.88220761950379,-29.5634642304892,23.5760760069919));
#50713=CARTESIAN_POINT('Ctrl Pts',(6.88220761950379,-53.1395402374811,-5.98738822349723));
#50714=CARTESIAN_POINT('Ctrl Pts',(6.88220761950379,-23.5760760069919,-29.5634642304892));
#50715=CARTESIAN_POINT('Ctrl Pts',(6.88220761950379,5.98738822349723,-53.1395402374811));
#50716=CARTESIAN_POINT('Ctrl Pts',(6.88220761950379,29.5634642304892,-23.5760760069919));
#50717=CARTESIAN_POINT('Ctrl Pts',(6.88220761950379,53.1395402374811,5.98738822349723));
#50718=CARTESIAN_POINT('Ctrl Pts',(6.88220761950379,23.5760760069919,29.5634642304892));
#50719=CARTESIAN_POINT('Ctrl Pts',(6.43560997955544,23.9429907960904,30.0235608233205));
#50720=CARTESIAN_POINT('Ctrl Pts',(6.43560997955544,-6.08057002723012,53.9665516194108));
#50721=CARTESIAN_POINT('Ctrl Pts',(6.43560997955544,-30.0235608233205,23.9429907960904));
#50722=CARTESIAN_POINT('Ctrl Pts',(6.43560997955544,-53.9665516194108,-6.08057002723012));
#50723=CARTESIAN_POINT('Ctrl Pts',(6.43560997955544,-23.9429907960904,-30.0235608233205));
#50724=CARTESIAN_POINT('Ctrl Pts',(6.43560997955544,6.08057002723012,-53.9665516194108));
#50725=CARTESIAN_POINT('Ctrl Pts',(6.43560997955544,30.0235608233205,-23.9429907960904));
#50726=CARTESIAN_POINT('Ctrl Pts',(6.43560997955544,53.9665516194108,6.08057002723012));
#50727=CARTESIAN_POINT('Ctrl Pts',(6.43560997955544,23.9429907960904,30.0235608233205));
#50728=CARTESIAN_POINT('Ctrl Pts',(6.14415685965718,24.1911416066824,30.3347320975618));
#50729=CARTESIAN_POINT('Ctrl Pts',(6.14415685965718,-6.14359049087935,54.5258737042442));
#50730=CARTESIAN_POINT('Ctrl Pts',(6.14415685965718,-30.3347320975618,24.1911416066824));
#50731=CARTESIAN_POINT('Ctrl Pts',(6.14415685965718,-54.5258737042442,-6.14359049087935));
#50732=CARTESIAN_POINT('Ctrl Pts',(6.14415685965718,-24.1911416066824,-30.3347320975618));
#50733=CARTESIAN_POINT('Ctrl Pts',(6.14415685965718,6.14359049087935,-54.5258737042442));
#50734=CARTESIAN_POINT('Ctrl Pts',(6.14415685965718,30.3347320975618,-24.1911416066824));
#50735=CARTESIAN_POINT('Ctrl Pts',(6.14415685965718,54.5258737042442,6.14359049087935));
#50736=CARTESIAN_POINT('Ctrl Pts',(6.14415685965718,24.1911416066824,30.3347320975618));
#50737=CARTESIAN_POINT('Ctrl Pts',(6.,24.3161022724906,30.4914278162532));
#50738=CARTESIAN_POINT('Ctrl Pts',(6.,-6.17532554376255,54.8075300887438));
#50739=CARTESIAN_POINT('Ctrl Pts',(6.,-30.4914278162532,24.3161022724906));
#50740=CARTESIAN_POINT('Ctrl Pts',(6.,-54.8075300887438,-6.17532554376255));
#50741=CARTESIAN_POINT('Ctrl Pts',(6.,-24.3161022724906,-30.4914278162532));
#50742=CARTESIAN_POINT('Ctrl Pts',(6.,6.17532554376255,-54.8075300887438));
#50743=CARTESIAN_POINT('Ctrl Pts',(6.,30.4914278162532,-24.3161022724906));
#50744=CARTESIAN_POINT('Ctrl Pts',(6.,54.8075300887438,6.17532554376255));
#50745=CARTESIAN_POINT('Ctrl Pts',(6.,24.3161022724906,30.4914278162532));
#50746=CARTESIAN_POINT('Ctrl Pts',(15.,13.5614880461774,27.4307499345787));
#50747=CARTESIAN_POINT('Ctrl Pts',(14.0108432136945,12.4969221179203,28.6513499963111));
#50748=CARTESIAN_POINT('Ctrl Pts',(13.3692319443824,11.7633381143331,29.4077674850275));
#50749=CARTESIAN_POINT('Ctrl Pts',(12.3476991724842,11.0009106836133,30.5055001671566));
#50750=CARTESIAN_POINT('Ctrl Pts',(12.0250187050191,10.7600760804358,30.8522505649563));
#50751=CARTESIAN_POINT('Ctrl Pts',(11.666631757071,10.497479920601,31.2404168505702));
#50752=CARTESIAN_POINT('Ctrl Pts',(11.3593868751766,10.2901330191653,31.573824809279));
#50753=CARTESIAN_POINT('Ctrl Pts',(10.6767716809131,9.82946417244362,32.3145672981358));
#50754=CARTESIAN_POINT('Ctrl Pts',(10.1321636914397,9.53982175368366,32.908348900279));
#50755=CARTESIAN_POINT('Ctrl Pts',(9.56604173138328,9.37660968812532,33.5284683378389));
#50756=CARTESIAN_POINT('Ctrl Pts',(9.3456307858919,9.3130655611995,33.7699023771341));
#50757=CARTESIAN_POINT('Ctrl Pts',(9.12222951098702,9.26933558002086,34.0154794389242));
#50758=CARTESIAN_POINT('Ctrl Pts',(8.88860711505289,9.24004324040524,34.2766867816041));
#50759=CARTESIAN_POINT('Ctrl Pts',(8.7583060070075,9.22370566157897,34.4223731831355));
#50760=CARTESIAN_POINT('Ctrl Pts',(8.62340343546557,9.209707571039,34.5735952627387));
#50761=CARTESIAN_POINT('Ctrl Pts',(8.40819516300421,9.20095382247576,34.8205073252293));
#50762=CARTESIAN_POINT('Ctrl Pts',(8.02443006829131,9.18534390605366,35.2608074585084));
#50763=CARTESIAN_POINT('Ctrl Pts',(7.46417034513342,9.20821248841079,35.9195836189444));
#50764=CARTESIAN_POINT('Ctrl Pts',(6.85957019142019,9.2876548102706,36.6968497152622));
#50765=CARTESIAN_POINT('Ctrl Pts',(6.58024553736738,9.32435708190311,37.0559458586018));
#50766=CARTESIAN_POINT('Ctrl Pts',(6.28976782192772,9.39495954165252,37.4362618349962));
#50767=CARTESIAN_POINT('Ctrl Pts',(6.,9.48407679455224,37.8292517419395));
#50768=CARTESIAN_POINT('Ctrl Pts',(2.09999999999999,4.3891074818719,15.1853730503683));
#50769=CARTESIAN_POINT('Ctrl Pts',(2.73333333333333,4.3891074818719,15.1853730503683));
#50770=CARTESIAN_POINT('Ctrl Pts',(3.36803488963027,4.38906293639893,15.1853891480969));
#50771=CARTESIAN_POINT('Ctrl Pts',(4.25277181297707,4.38903510934131,15.1853984318492));
#50772=CARTESIAN_POINT('Ctrl Pts',(4.77266992155204,4.38096760094831,15.1878257280945));
#50773=CARTESIAN_POINT('Ctrl Pts',(5.76857034429174,4.35758589293773,15.1949135576046));
#50774=CARTESIAN_POINT('Ctrl Pts',(6.4850861707799,4.35822862174715,15.1947749329422));
#50775=CARTESIAN_POINT('Ctrl Pts',(6.9986641671015,4.39061489150108,15.1847594251365));
#50776=CARTESIAN_POINT('Ctrl Pts',(7.12480344747274,4.39885659944923,15.1823276020454));
#50777=CARTESIAN_POINT('Ctrl Pts',(7.37170623914911,4.4162608941154,15.177371808595));
#50778=CARTESIAN_POINT('Ctrl Pts',(7.68211418916856,4.440773054857,15.1706560971746));
#50779=CARTESIAN_POINT('Ctrl Pts',(8.0507418084214,4.47522277126092,15.1612435681501));
#50780=CARTESIAN_POINT('Ctrl Pts',(8.41504100892412,4.51550554400247,15.1499364273002));
#50781=CARTESIAN_POINT('Ctrl Pts',(9.01074910230582,4.59375299963977,15.1269946547022));
#50782=CARTESIAN_POINT('Ctrl Pts',(9.46309896700665,4.67554497516132,15.1008422997988));
#50783=CARTESIAN_POINT('Ctrl Pts',(10.2678495141822,4.86554628727075,15.0344005222421));
#50784=CARTESIAN_POINT('Ctrl Pts',(10.9804938765534,5.10715483420763,14.9562757133094));
#50785=CARTESIAN_POINT('Ctrl Pts',(11.7910258900602,5.45630749934349,14.833110998574));
#50786=CARTESIAN_POINT('Ctrl Pts',(12.2471544524677,5.66565497142133,14.7535780631897));
#50787=CARTESIAN_POINT('Ctrl Pts',(12.4732504394558,5.77217429860475,14.7107195079034));
#50788=CARTESIAN_POINT('Ctrl Pts',(12.8351209164145,5.94360272017494,14.6392957979959));
#50789=CARTESIAN_POINT('Ctrl Pts',(13.2802518542094,6.17499175205375,14.5408686766578));
#50790=CARTESIAN_POINT('Ctrl Pts',(14.161256864772,6.69818327390388,14.3113175847781));
#50791=CARTESIAN_POINT('Ctrl Pts',(14.7820737708942,7.12182950163928,14.1077824544514));
#50792=CARTESIAN_POINT('Ctrl Pts',(15.1979896574214,7.40598969975549,13.9553299864943));
#50793=CARTESIAN_POINT('Ctrl Pts',(2.09999999999999,6.11056057998312,22.7275518693282));
#50794=CARTESIAN_POINT('Ctrl Pts',(2.73333333333333,6.11056057998312,22.7275518693282));
#50795=CARTESIAN_POINT('Ctrl Pts',(3.36872139010523,6.11055911614926,22.7275501174862));
#50796=CARTESIAN_POINT('Ctrl Pts',(4.25415709201328,6.11054559328987,22.7275524283132));
#50797=CARTESIAN_POINT('Ctrl Pts',(4.7831009051333,6.09839208015139,22.7309599500369));
#50798=CARTESIAN_POINT('Ctrl Pts',(5.77494051300236,6.06343326294559,22.740847682661));
#50799=CARTESIAN_POINT('Ctrl Pts',(6.4749722897255,6.06484508260633,22.7405177238962));
#50800=CARTESIAN_POINT('Ctrl Pts',(6.96727417314943,6.11201313509931,22.726891120736));
#50801=CARTESIAN_POINT('Ctrl Pts',(7.09309213456251,6.12432705592286,22.7235075398897));
#50802=CARTESIAN_POINT('Ctrl Pts',(7.33629159574246,6.15012383123003,22.7166894865964));
#50803=CARTESIAN_POINT('Ctrl Pts',(7.64236714688785,6.18649753874622,22.7074653368708));
#50804=CARTESIAN_POINT('Ctrl Pts',(8.00392257679634,6.237416056974,22.6946063739332));
#50805=CARTESIAN_POINT('Ctrl Pts',(8.36001575867264,6.29687420312726,22.6791486280887));
#50806=CARTESIAN_POINT('Ctrl Pts',(8.93968276887491,6.4119109021405,22.6478374700045));
#50807=CARTESIAN_POINT('Ctrl Pts',(9.37529806425592,6.53175739185493,22.6120247145612));
#50808=CARTESIAN_POINT('Ctrl Pts',(10.1434048645354,6.80789230240586,22.5213547453348));
#50809=CARTESIAN_POINT('Ctrl Pts',(10.8342970263929,7.16164219057595,22.4150634069346));
#50810=CARTESIAN_POINT('Ctrl Pts',(11.6346844994435,7.68020478527314,22.2442660982912));
#50811=CARTESIAN_POINT('Ctrl Pts',(12.0872580001815,7.99240455061643,22.1329978262207));
#50812=CARTESIAN_POINT('Ctrl Pts',(12.3122495048507,8.15169147256195,22.0726789031247));
#50813=CARTESIAN_POINT('Ctrl Pts',(12.6725882088788,8.40825142471423,21.9718916318112));
#50814=CARTESIAN_POINT('Ctrl Pts',(13.1110153447534,8.75180009316219,21.8345430981404));
#50815=CARTESIAN_POINT('Ctrl Pts',(13.992134418419,9.5365949967812,21.5103916607701));
#50816=CARTESIAN_POINT('Ctrl Pts',(14.6125773377935,10.1751048259157,21.2201485554486));
#50817=CARTESIAN_POINT('Ctrl Pts',(15.0291266285127,10.603144101066,21.0018664882136));
#50818=CARTESIAN_POINT('Ctrl Pts',(2.09999999999999,7.83201367809433,30.2697306882881));
#50819=CARTESIAN_POINT('Ctrl Pts',(2.73333333333333,7.83201367809433,30.2697306882881));
#50820=CARTESIAN_POINT('Ctrl Pts',(3.36945654347763,7.83198149032742,30.2697430182653));
#50821=CARTESIAN_POINT('Ctrl Pts',(4.25562154880783,7.83194277590752,30.2697546322492));
#50822=CARTESIAN_POINT('Ctrl Pts',(4.79359271386228,7.81549328468654,30.2741980639674));
#50823=CARTESIAN_POINT('Ctrl Pts',(5.7814667007226,7.76899455850239,30.2868791804613));
#50824=CARTESIAN_POINT('Ctrl Pts',(6.46487450280797,7.77155275140848,30.2862961028278));
#50825=CARTESIAN_POINT('Ctrl Pts',(6.93655488526515,7.83145888919768,30.269537124378));
#50826=CARTESIAN_POINT('Ctrl Pts',(7.06206674963109,7.84780648351963,30.2652120527099));
#50827=CARTESIAN_POINT('Ctrl Pts',(7.30169782506139,7.88161308928391,30.2566222703851));
#50828=CARTESIAN_POINT('Ctrl Pts',(7.60367667602142,7.92929132068129,30.2450297222388));
#50829=CARTESIAN_POINT('Ctrl Pts',(7.9586139633519,7.99573552796043,30.2289506497327));
#50830=CARTESIAN_POINT('Ctrl Pts',(8.30732259385584,8.07297763461527,30.2096953931838));
#50831=CARTESIAN_POINT('Ctrl Pts',(8.87311432258292,8.22194296928411,30.1707221913514));
#50832=CARTESIAN_POINT('Ctrl Pts',(9.29619366695843,8.37561549009779,30.1263948339446));
#50833=CARTESIAN_POINT('Ctrl Pts',(10.0462821922003,8.72945832787965,30.0139523275426));
#50834=CARTESIAN_POINT('Ctrl Pts',(10.7405250303565,9.19532650893385,29.880083738196));
#50835=CARTESIAN_POINT('Ctrl Pts',(11.5482319135987,9.88948391526171,29.6602270293575));
#50836=CARTESIAN_POINT('Ctrl Pts',(12.0041864194649,10.3073475275797,29.5165115073217));
#50837=CARTESIAN_POINT('Ctrl Pts',(12.2304191147553,10.5204751681415,29.4384637783906));
#50838=CARTESIAN_POINT('Ctrl Pts',(12.5924573698282,10.8635518683441,29.3079798844092));
#50839=CARTESIAN_POINT('Ctrl Pts',(13.0427811260593,11.3303280696709,29.1279900325959));
#50840=CARTESIAN_POINT('Ctrl Pts',(13.9385914588617,12.3939356634149,28.7020154314488));
#50841=CARTESIAN_POINT('Ctrl Pts',(14.5670688438605,13.2551537949985,28.3206820720608));
#50842=CARTESIAN_POINT('Ctrl Pts',(14.9853697475044,13.8290419584993,28.0347711649074));
#50843=CARTESIAN_POINT('Ctrl Pts',(2.09999999999999,9.55346677620554,37.8119095072481));
#50844=CARTESIAN_POINT('Ctrl Pts',(2.73333333333333,9.55346677620554,37.8119095072481));
#50845=CARTESIAN_POINT('Ctrl Pts',(3.37020742035998,9.55341753387,37.8119325809509));
#50846=CARTESIAN_POINT('Ctrl Pts',(4.25712565984989,9.55335946206722,37.8119521381032));
#50847=CARTESIAN_POINT('Ctrl Pts',(4.80403043076164,9.53243579429088,37.8174716594016));
#50848=CARTESIAN_POINT('Ctrl Pts',(5.7881431164665,9.47448886427121,37.8329257348436));
#50849=CARTESIAN_POINT('Ctrl Pts',(6.45446254072639,9.47858058983615,37.8319994104911));
#50850=CARTESIAN_POINT('Ctrl Pts',(6.9069189360726,9.5496032041587,37.8124809392428));
#50851=CARTESIAN_POINT('Ctrl Pts',(7.03215479329302,9.56995797627607,37.8072212231688));
#50852=CARTESIAN_POINT('Ctrl Pts',(7.26850522383847,9.61147955883885,37.7969291135373));
#50853=CARTESIAN_POINT('Ctrl Pts',(7.56684411441826,9.67009901821235,37.7830552828907));
#50854=CARTESIAN_POINT('Ctrl Pts',(7.91606061411963,9.75146832226317,37.7639015082074));
#50855=CARTESIAN_POINT('Ctrl Pts',(8.25885653597654,9.84584964259562,37.7410100895783));
#50856=CARTESIAN_POINT('Ctrl Pts',(8.81428255427399,10.0277862636405,37.6946225034532));
#50857=CARTESIAN_POINT('Ctrl Pts',(9.23054659804177,10.2153622393428,37.6418005979312));
#50858=CARTESIAN_POINT('Ctrl Pts',(9.97650814168219,10.6540278309757,37.5057959766103));
#50859=CARTESIAN_POINT('Ctrl Pts',(10.6790276368305,11.2442721267542,37.3408941588814));
#50860=CARTESIAN_POINT('Ctrl Pts',(11.4920938550392,12.1204102224677,37.0694466964272));
#50861=CARTESIAN_POINT('Ctrl Pts',(11.9504461727733,12.6463277688412,36.8921482749081));
#50862=CARTESIAN_POINT('Ctrl Pts',(12.1774757766432,12.9139906211525,36.7959324971495));
#50863=CARTESIAN_POINT('Ctrl Pts',(12.5406754666789,13.3445351774205,36.6350970810471));
#50864=CARTESIAN_POINT('Ctrl Pts',(12.997674859905,13.9394605109857,36.410163322069));
#50865=CARTESIAN_POINT('Ctrl Pts',(13.8994007067086,15.2825523021509,35.8806497606637));
#50866=CARTESIAN_POINT('Ctrl Pts',(14.5324532885843,16.3664333186909,35.4071727167216));
#50867=CARTESIAN_POINT('Ctrl Pts',(14.9514110803021,17.0856438928078,35.0531141757479));
#50868=CARTESIAN_POINT('',(3.2,9.24182505978396,36.4465179346992));
#50869=CARTESIAN_POINT('Ctrl Pts',(3.2,9.24182505978395,36.4465179346992));
#50870=CARTESIAN_POINT('Ctrl Pts',(3.56152274835423,8.9933749145984,35.3579867254307));
#50871=CARTESIAN_POINT('Ctrl Pts',(3.95224584525383,8.7474300544665,34.2543624244307));
#50872=CARTESIAN_POINT('Ctrl Pts',(4.78767430123771,8.22468504571474,32.0637774306311));
#50873=CARTESIAN_POINT('Ctrl Pts',(5.21513946232109,7.95930413376433,31.0187779627676));
#50874=CARTESIAN_POINT('Ctrl Pts',(6.79548775402598,7.09591997179492,27.3868928737702));
#50875=CARTESIAN_POINT('Ctrl Pts',(7.94016295939418,6.79083791828153,25.1816377053514));
#50876=CARTESIAN_POINT('Ctrl Pts',(9.46271935275874,6.48646562505714,22.4189535945791));
#50877=CARTESIAN_POINT('Ctrl Pts',(10.1385443659107,6.45732153174645,21.2736802981369));
#50878=CARTESIAN_POINT('Ctrl Pts',(11.5967860400751,6.61157417320919,18.9321092259658));
#50879=CARTESIAN_POINT('Ctrl Pts',(12.3997356677092,6.72026811283589,17.7072930059352));
#50880=CARTESIAN_POINT('Ctrl Pts',(13.6850585208092,6.95369959664903,15.8347320436374));
#50881=CARTESIAN_POINT('Ctrl Pts',(14.3457395898607,7.12290839200202,14.9017490241179));
#50882=CARTESIAN_POINT('Ctrl Pts',(15.,7.27088643053102,14.0266249226733));
#50883=CARTESIAN_POINT('Ctrl Pts',(2.79815110085753,9.45113165484999,37.3636308035525));
#50884=CARTESIAN_POINT('Ctrl Pts',(2.93286156280202,9.38137424991818,37.0580309336991));
#50885=CARTESIAN_POINT('Ctrl Pts',(3.06772962045781,9.31157137579472,36.7522364869069));
#50886=CARTESIAN_POINT('Ctrl Pts',(3.20258220903908,9.2417890578256,36.4465334820215));
#50887=CARTESIAN_POINT('Origin',(2.9,0.,0.));
#50888=CARTESIAN_POINT('',(3.2,22.7328514723457,29.9495820327474));
#50889=CARTESIAN_POINT('Origin',(3.2,0.,0.));
#50890=CARTESIAN_POINT('Ctrl Pts',(3.19853733010153,22.732905589146,29.9495159265607));
#50891=CARTESIAN_POINT('Ctrl Pts',(3.06441888114801,22.9284975216313,30.1948057550582));
#50892=CARTESIAN_POINT('Ctrl Pts',(2.93030256786884,23.1240541237703,30.4400509061236));
#50893=CARTESIAN_POINT('Ctrl Pts',(2.79629549285327,23.3193875333591,30.685012507583));
#50894=CARTESIAN_POINT('Ctrl Pts',(2.09999999999999,13.8302329243183,7.6592137863052));
#50895=CARTESIAN_POINT('Ctrl Pts',(2.73333333333332,13.8302329243183,7.6592137863052));
#50896=CARTESIAN_POINT('Ctrl Pts',(3.3659678189539,13.8302628375624,7.65913128553974));
#50897=CARTESIAN_POINT('Ctrl Pts',(4.12347856757956,13.8302719183902,7.65910593972428));
#50898=CARTESIAN_POINT('Ctrl Pts',(4.36307193792893,13.829345007715,7.66082148123924));
#50899=CARTESIAN_POINT('Ctrl Pts',(4.85755706347495,13.8250800963554,7.66874120057285));
#50900=CARTESIAN_POINT('Ctrl Pts',(5.73897676214029,13.81494964431,7.68759310001621));
#50901=CARTESIAN_POINT('Ctrl Pts',(6.5260410124842,13.8146756387459,7.68813277015824));
#50902=CARTESIAN_POINT('Ctrl Pts',(7.12755042026095,13.8333496467612,7.65307471747093));
#50903=CARTESIAN_POINT('Ctrl Pts',(7.25504570216537,13.8375192712337,7.64544084036889));
#50904=CARTESIAN_POINT('Ctrl Pts',(7.51730430878851,13.8468894755058,7.62865310498325));
#50905=CARTESIAN_POINT('Ctrl Pts',(7.84587135530479,13.8602867128817,7.60514723495773));
#50906=CARTESIAN_POINT('Ctrl Pts',(8.24415002878778,13.8794323696111,7.5715870957123));
#50907=CARTESIAN_POINT('Ctrl Pts',(8.77644954625804,13.9094630260358,7.51804251641122));
#50908=CARTESIAN_POINT('Ctrl Pts',(9.4411196057495,13.9562092623828,7.43162866581977));
#50909=CARTESIAN_POINT('Ctrl Pts',(9.96386966585737,14.0053914713958,7.33433060678515));
#50910=CARTESIAN_POINT('Ctrl Pts',(11.1188970074167,14.1318056158801,7.07452696639597));
#50911=CARTESIAN_POINT('Ctrl Pts',(12.0804360933392,14.3149505401524,6.71516750612135));
#50912=CARTESIAN_POINT('Ctrl Pts',(13.0008252351436,14.4960346678446,6.30114540183651));
#50913=CARTESIAN_POINT('Ctrl Pts',(13.2108022543453,14.5369701280712,6.20370984482182));
#50914=CARTESIAN_POINT('Ctrl Pts',(13.3144255310506,14.5569642596936,6.15498827691463));
#50915=CARTESIAN_POINT('Ctrl Pts',(13.3733054984755,14.5682547807254,6.1271355373132));
#50916=CARTESIAN_POINT('Ctrl Pts',(13.4025846876148,14.5738432840613,6.11323204156111));
#50917=CARTESIAN_POINT('Ctrl Pts',(13.6877790496802,14.6281168885643,5.97754713224256));
#50918=CARTESIAN_POINT('Ctrl Pts',(14.2465793638156,14.7431165252461,5.68371239772979));
#50919=CARTESIAN_POINT('Ctrl Pts',(14.7537307590314,14.8582149808983,5.37191114117815));
#50920=CARTESIAN_POINT('Ctrl Pts',(14.9999999999997,14.914658515108,5.21200130317825));
#50921=CARTESIAN_POINT('Ctrl Pts',(2.09999999999999,20.7995074576498,11.0154395130593));
#50922=CARTESIAN_POINT('Ctrl Pts',(2.73333333333333,20.7995074576498,11.0154395130593));
#50923=CARTESIAN_POINT('Ctrl Pts',(3.36558111194426,20.7995325669748,11.0153792642041));
#50924=CARTESIAN_POINT('Ctrl Pts',(4.12267542201538,20.7995396015868,11.0153621943559));
#50925=CARTESIAN_POINT('Ctrl Pts',(4.35698849797995,20.7982251231441,11.0179127481155));
#50926=CARTESIAN_POINT('Ctrl Pts',(4.84799134950577,20.7921297696213,11.0297698437277));
#50927=CARTESIAN_POINT('Ctrl Pts',(5.73067616595878,20.7775586661749,11.0581537306883));
#50928=CARTESIAN_POINT('Ctrl Pts',(6.53593220712833,20.776963041793,11.0593869811326));
#50929=CARTESIAN_POINT('Ctrl Pts',(7.15868312259406,20.8044557954121,11.0054825453739));
#50930=CARTESIAN_POINT('Ctrl Pts',(7.28650801289721,20.810461084153,10.9939824326641));
#50931=CARTESIAN_POINT('Ctrl Pts',(7.55247181782137,20.8240667812859,10.9685056887052));
#50932=CARTESIAN_POINT('Ctrl Pts',(7.8853971788604,20.8435142926672,10.9328673721134));
#50933=CARTESIAN_POINT('Ctrl Pts',(8.29075151198502,20.871389579138,10.8818111380178));
#50934=CARTESIAN_POINT('Ctrl Pts',(8.83402157842737,20.915167083861,10.8002514899699));
#50935=CARTESIAN_POINT('Ctrl Pts',(9.51596599837448,20.9834880538297,10.6681977805184));
#50936=CARTESIAN_POINT('Ctrl Pts',(10.0562863332648,21.0556116709674,10.5189202217359));
#50937=CARTESIAN_POINT('Ctrl Pts',(11.2545127308448,21.2415419513394,10.1190530365671));
#50938=CARTESIAN_POINT('Ctrl Pts',(12.2341721931925,21.5079926455151,9.57090330100297));
#50939=CARTESIAN_POINT('Ctrl Pts',(13.1607695825083,21.7667490771537,8.9461536326231));
#50940=CARTESIAN_POINT('Ctrl Pts',(13.3718704518382,21.825081315333,8.79927791727695));
#50941=CARTESIAN_POINT('Ctrl Pts',(13.4759187928771,21.8535069727006,8.72590068814449));
#50942=CARTESIAN_POINT('Ctrl Pts',(13.5350226376953,21.8695447648399,8.68396491535917));
#50943=CARTESIAN_POINT('Ctrl Pts',(13.5643924514481,21.8774759629775,8.66303720261835));
#50944=CARTESIAN_POINT('Ctrl Pts',(13.8508852807691,21.9545130564942,8.45883878182458));
#50945=CARTESIAN_POINT('Ctrl Pts',(14.4159013980166,22.1190480003223,8.01397192202503));
#50946=CARTESIAN_POINT('Ctrl Pts',(14.9236315787721,22.2815286141703,7.54600523920185));
#50947=CARTESIAN_POINT('Ctrl Pts',(15.169681381964,22.3609519415738,7.30611779695347));
#50948=CARTESIAN_POINT('Ctrl Pts',(2.09999999999999,27.7687819909813,14.3716652398135));
#50949=CARTESIAN_POINT('Ctrl Pts',(2.73333333333332,27.7687819909813,14.3716652398135));
#50950=CARTESIAN_POINT('Ctrl Pts',(3.36511119330026,27.7688208479248,14.3715582517052));
#50951=CARTESIAN_POINT('Ctrl Pts',(4.12176441016776,27.7688314711666,14.3715280007939));
#50952=CARTESIAN_POINT('Ctrl Pts',(4.3507849905463,27.7671558884117,14.3748560117099));
#50953=CARTESIAN_POINT('Ctrl Pts',(4.83832025888307,27.7592832848126,14.3905340890695));
#50954=CARTESIAN_POINT('Ctrl Pts',(5.72215842021101,27.7402636513287,14.4284570078183));
#50955=CARTESIAN_POINT('Ctrl Pts',(6.54570094113893,27.7391506882908,14.4307425531356));
#50956=CARTESIAN_POINT('Ctrl Pts',(7.1890160219809,27.7763611050952,14.3560985578327));
#50957=CARTESIAN_POINT('Ctrl Pts',(7.31715408996789,27.7842178101884,14.3406964044614));
#50958=CARTESIAN_POINT('Ctrl Pts',(7.58668580864389,27.8022272202947,14.3061738683707));
#50959=CARTESIAN_POINT('Ctrl Pts',(7.92371615677765,27.8279600361707,14.2578885292085));
#50960=CARTESIAN_POINT('Ctrl Pts',(8.33568805882525,27.8649806117798,14.1884448255293));
#50961=CARTESIAN_POINT('Ctrl Pts',(8.88880106775738,27.9232779595706,14.0771711465573));
#50962=CARTESIAN_POINT('Ctrl Pts',(9.58535043882608,28.01462294777,13.896270217051));
#50963=CARTESIAN_POINT('Ctrl Pts',(10.137537931292,28.1114587716087,13.6909226061858));
#50964=CARTESIAN_POINT('Ctrl Pts',(11.3565147873056,28.3608087900239,13.141482355084));
#50965=CARTESIAN_POINT('Ctrl Pts',(12.3227992560538,28.7078636311036,12.408808264513));
#50966=CARTESIAN_POINT('Ctrl Pts',(13.2438207447798,29.0418838222233,11.5788287297239));
#50967=CARTESIAN_POINT('Ctrl Pts',(13.4536674751769,29.1171877957502,11.3834544055582));
#50968=CARTESIAN_POINT('Ctrl Pts',(13.5572312471348,29.1538524613806,11.2858597235973));
#50969=CARTESIAN_POINT('Ctrl Pts',(13.6160706434025,29.1745370684473,11.2300668162362));
#50970=CARTESIAN_POINT('Ctrl Pts',(13.6453277307064,29.1847642914313,11.202221221814));
#50971=CARTESIAN_POINT('Ctrl Pts',(13.9304198199502,29.2840965816901,10.9305095482656));
#50972=CARTESIAN_POINT('Ctrl Pts',(14.4834678155218,29.4940622370905,10.3461367513705));
#50973=CARTESIAN_POINT('Ctrl Pts',(14.98335392639,29.7014377889178,9.73077947062731));
#50974=CARTESIAN_POINT('Ctrl Pts',(15.2260186760796,29.8027827396015,9.41523068650629));
#50975=CARTESIAN_POINT('Ctrl Pts',(2.09999999999999,34.7380565243128,17.7278909665676));
#50976=CARTESIAN_POINT('Ctrl Pts',(2.73333333333332,34.7380565243128,17.7278909665676));
#50977=CARTESIAN_POINT('Ctrl Pts',(3.36463301569964,34.7380950962072,17.7277674494899));
#50978=CARTESIAN_POINT('Ctrl Pts',(4.12084721759174,34.7381049772718,17.7277334070115));
#50979=CARTESIAN_POINT('Ctrl Pts',(4.34456258524319,34.7360905272795,17.731792616583));
#50980=CARTESIAN_POINT('Ctrl Pts',(4.82870429948491,34.7264911965689,17.7511877392265));
#50981=CARTESIAN_POINT('Ctrl Pts',(5.71349193736137,34.702986637018,17.7987242584056));
#50982=CARTESIAN_POINT('Ctrl Pts',(6.55582455797101,34.7011703174735,17.8024535759284));
#50983=CARTESIAN_POINT('Ctrl Pts',(7.21831310628172,34.7488125263721,17.7055813111283));
#50984=CARTESIAN_POINT('Ctrl Pts',(7.34673507590046,34.7585314597734,17.6862529310369));
#50985=CARTESIAN_POINT('Ctrl Pts',(7.61954646390551,34.7810737524572,17.6424115760599));
#50986=CARTESIAN_POINT('Ctrl Pts',(7.96023436813318,34.8132455546453,17.5811514236554));
#50987=CARTESIAN_POINT('Ctrl Pts',(8.37791666755937,34.8596727342253,17.4927579600399));
#50988=CARTESIAN_POINT('Ctrl Pts',(8.93895172116899,34.9328458405683,17.3509922932392));
#50989=CARTESIAN_POINT('Ctrl Pts',(9.64586775066713,35.0475998470716,17.1203589614845));
#50990=CARTESIAN_POINT('Ctrl Pts',(10.2035544184636,35.1686409304077,16.8599692096752));
#50991=CARTESIAN_POINT('Ctrl Pts',(11.4269491626946,35.4776285918087,16.1692409322816));
#50992=CARTESIAN_POINT('Ctrl Pts',(12.379436542279,35.8995568801641,15.2663852248503));
#50993=CARTESIAN_POINT('Ctrl Pts',(13.2972580417114,36.308207182279,14.2349957870837));
#50994=CARTESIAN_POINT('Ctrl Pts',(13.5062277931751,36.4003157142188,13.9920233463097));
#50995=CARTESIAN_POINT('Ctrl Pts',(13.6095005039641,36.4451932562173,13.8705333276639));
#50996=CARTESIAN_POINT('Ctrl Pts',(13.6681736295282,36.4705108919158,13.8010624659116));
#50997=CARTESIAN_POINT('Ctrl Pts',(13.6973660627842,36.4830331801897,13.7663739662738));
#50998=CARTESIAN_POINT('Ctrl Pts',(13.9814652731774,36.6045664539301,13.4281004008165));
#50999=CARTESIAN_POINT('Ctrl Pts',(14.5280851725163,36.8587744770471,12.7093432028732));
#51000=CARTESIAN_POINT('Ctrl Pts',(15.0243070371674,37.1114272400404,11.9476665753718));
#51001=CARTESIAN_POINT('Ctrl Pts',(15.2656150130537,37.2349788009363,11.5567205320759));
#51002=CARTESIAN_POINT('Ctrl Pts',(3.19846718588995,33.4762534656926,17.1201468043523));
#51003=CARTESIAN_POINT('Ctrl Pts',(3.06436072639559,33.7589037690507,17.2562800913157));
#51004=CARTESIAN_POINT('Ctrl Pts',(2.93025712268473,34.0415012332836,17.3923884232182));
#51005=CARTESIAN_POINT('Ctrl Pts',(2.79626186145775,34.3237730524972,17.5283379493497));
#51006=CARTESIAN_POINT('',(15.,29.0858399764131,9.50651949277382));
#51007=CARTESIAN_POINT('Ctrl Pts',(15.,29.0858399764131,9.50651949277382));
#51008=CARTESIAN_POINT('Ctrl Pts',(15.,24.8658325835021,8.21080036749256));
#51009=CARTESIAN_POINT('Ctrl Pts',(15.,19.8536655760794,6.68175134799012));
#51010=CARTESIAN_POINT('Ctrl Pts',(15.,14.914658515121,5.2120013031819));
#51011=CARTESIAN_POINT('Ctrl Pts',(6.,34.705361282547,17.7915119719457));
#51012=CARTESIAN_POINT('Ctrl Pts',(6.38595465246567,34.2221199480834,17.5579141160912));
#51013=CARTESIAN_POINT('Ctrl Pts',(6.77023648668261,33.7796441613039,17.3184113007142));
#51014=CARTESIAN_POINT('Ctrl Pts',(7.13915213286207,33.3921505763645,17.0677247897979));
#51015=CARTESIAN_POINT('Ctrl Pts',(8.10667920093239,32.3759005581963,16.4102683023233));
#51016=CARTESIAN_POINT('Ctrl Pts',(8.98019888747373,31.6651086781454,15.8112923224959));
#51017=CARTESIAN_POINT('Ctrl Pts',(9.46656009721078,31.309138019977,15.4476561949843));
#51018=CARTESIAN_POINT('Ctrl Pts',(9.65648624874914,31.1701299415921,15.3056547177367));
#51019=CARTESIAN_POINT('Ctrl Pts',(9.79228848853732,31.0768034028916,15.200839624557));
#51020=CARTESIAN_POINT('Ctrl Pts',(9.9459382572782,30.9753505916291,15.0790894852441));
#51021=CARTESIAN_POINT('Ctrl Pts',(10.1065740866009,30.8692849814572,14.9518036796165));
#51022=CARTESIAN_POINT('Ctrl Pts',(10.2660951669675,30.7697885322026,14.8212561902164));
#51023=CARTESIAN_POINT('Ctrl Pts',(10.4261869573617,30.6759975409703,14.6846181247282));
#51024=CARTESIAN_POINT('Ctrl Pts',(10.8065549509411,30.4531560631967,14.3599747017995));
#51025=CARTESIAN_POINT('Ctrl Pts',(11.1894211925257,30.2632188670013,14.0000944173254));
#51026=CARTESIAN_POINT('Ctrl Pts',(11.6023503255242,30.0893332260782,13.576802484847));
#51027=CARTESIAN_POINT('Ctrl Pts',(11.7531893954247,30.0258144615982,13.4221779832339));
#51028=CARTESIAN_POINT('Ctrl Pts',(11.9080270687775,29.9645492825341,13.2589920660579));
#51029=CARTESIAN_POINT('Ctrl Pts',(12.0681766131679,29.9049332499845,13.0857139522985));
#51030=CARTESIAN_POINT('Ctrl Pts',(12.1838435903474,29.8618759543631,12.9605649504314));
#51031=CARTESIAN_POINT('Ctrl Pts',(12.310086541016,29.8159567574697,12.8227195457579));
#51032=CARTESIAN_POINT('Ctrl Pts',(12.5127093730712,29.7480815967021,12.594280846792));
#51033=CARTESIAN_POINT('Ctrl Pts',(12.7975492664042,29.6526651356996,12.2731499357953));
#51034=CARTESIAN_POINT('Ctrl Pts',(13.1874566943566,29.5335094649651,11.8182959611235));
#51035=CARTESIAN_POINT('Ctrl Pts',(13.6431584568239,29.4049045698753,11.2769918204713));
#51036=CARTESIAN_POINT('Ctrl Pts',(14.069523646534,29.2845788327183,10.7705350506522));
#51037=CARTESIAN_POINT('Ctrl Pts',(14.53311408767,29.1791240620733,10.1666991941896));
#51038=CARTESIAN_POINT('Ctrl Pts',(15.,29.0858399764131,9.50651949277382));
#51039=CARTESIAN_POINT('Origin',(15.,8.5,0.));
#51040=CARTESIAN_POINT('',(15.,29.9016733813822,6.49999453793157));
#51041=CARTESIAN_POINT('Ctrl Pts',(15.,15.4997804972258,3.0608496769456));
#51042=CARTESIAN_POINT('Ctrl Pts',(15.,20.6459887015956,4.32127283870946));
#51043=CARTESIAN_POINT('Ctrl Pts',(15.,25.8455102356798,5.54875033084932));
#51044=CARTESIAN_POINT('Ctrl Pts',(15.,29.9016733813822,6.49999453793159));
#51045=CARTESIAN_POINT('Origin',(15.,0.,0.));
#51046=CARTESIAN_POINT('Ctrl Pts',(15.,30.6,0.));
#51047=CARTESIAN_POINT('Ctrl Pts',(15.,30.6,30.6));
#51048=CARTESIAN_POINT('Ctrl Pts',(15.,0.,30.6));
#51049=CARTESIAN_POINT('Ctrl Pts',(15.,-30.6,30.6));
#51050=CARTESIAN_POINT('Ctrl Pts',(15.,-30.6,0.));
#51051=CARTESIAN_POINT('Ctrl Pts',(15.,-30.6,-30.6));
#51052=CARTESIAN_POINT('Ctrl Pts',(15.,0.,-30.6));
#51053=CARTESIAN_POINT('Ctrl Pts',(15.,30.6,-30.6));
#51054=CARTESIAN_POINT('Ctrl Pts',(15.,30.6,0.));
#51055=CARTESIAN_POINT('Ctrl Pts',(14.7843073131059,30.7357147434939,0.));
#51056=CARTESIAN_POINT('Ctrl Pts',(14.7843073131059,30.7357147434939,30.7357147434939));
#51057=CARTESIAN_POINT('Ctrl Pts',(14.7843073131059,0.,30.7357147434939));
#51058=CARTESIAN_POINT('Ctrl Pts',(14.7843073131059,-30.7357147434939,30.7357147434939));
#51059=CARTESIAN_POINT('Ctrl Pts',(14.7843073131059,-30.7357147434939,0.));
#51060=CARTESIAN_POINT('Ctrl Pts',(14.7843073131059,-30.7357147434939,-30.7357147434939));
#51061=CARTESIAN_POINT('Ctrl Pts',(14.7843073131059,0.,-30.7357147434939));
#51062=CARTESIAN_POINT('Ctrl Pts',(14.7843073131059,30.7357147434939,-30.7357147434939));
#51063=CARTESIAN_POINT('Ctrl Pts',(14.7843073131059,30.7357147434939,0.));
#51064=CARTESIAN_POINT('Ctrl Pts',(14.3560298066371,31.009955402806,0.));
#51065=CARTESIAN_POINT('Ctrl Pts',(14.3560298066371,31.009955402806,31.009955402806));
#51066=CARTESIAN_POINT('Ctrl Pts',(14.3560298066371,0.,31.009955402806));
#51067=CARTESIAN_POINT('Ctrl Pts',(14.3560298066371,-31.009955402806,31.009955402806));
#51068=CARTESIAN_POINT('Ctrl Pts',(14.3560298066371,-31.009955402806,0.));
#51069=CARTESIAN_POINT('Ctrl Pts',(14.3560298066371,-31.009955402806,-31.009955402806));
#51070=CARTESIAN_POINT('Ctrl Pts',(14.3560298066371,0.,-31.009955402806));
#51071=CARTESIAN_POINT('Ctrl Pts',(14.3560298066371,31.009955402806,-31.009955402806));
#51072=CARTESIAN_POINT('Ctrl Pts',(14.3560298066371,31.009955402806,0.));
#51073=CARTESIAN_POINT('Ctrl Pts',(13.722936818686,31.4297496100642,0.));
#51074=CARTESIAN_POINT('Ctrl Pts',(13.722936818686,31.4297496100642,31.4297496100642));
#51075=CARTESIAN_POINT('Ctrl Pts',(13.722936818686,0.,31.4297496100642));
#51076=CARTESIAN_POINT('Ctrl Pts',(13.722936818686,-31.4297496100642,31.4297496100642));
#51077=CARTESIAN_POINT('Ctrl Pts',(13.722936818686,-31.4297496100642,0.));
#51078=CARTESIAN_POINT('Ctrl Pts',(13.722936818686,-31.4297496100642,-31.4297496100642));
#51079=CARTESIAN_POINT('Ctrl Pts',(13.722936818686,0.,-31.4297496100642));
#51080=CARTESIAN_POINT('Ctrl Pts',(13.722936818686,31.4297496100642,-31.4297496100642));
#51081=CARTESIAN_POINT('Ctrl Pts',(13.722936818686,31.4297496100642,0.));
#51082=CARTESIAN_POINT('Ctrl Pts',(12.8977690042853,32.0066217236598,0.));
#51083=CARTESIAN_POINT('Ctrl Pts',(12.8977690042853,32.0066217236598,32.0066217236598));
#51084=CARTESIAN_POINT('Ctrl Pts',(12.8977690042853,0.,32.0066217236598));
#51085=CARTESIAN_POINT('Ctrl Pts',(12.8977690042853,-32.0066217236598,32.0066217236598));
#51086=CARTESIAN_POINT('Ctrl Pts',(12.8977690042853,-32.0066217236598,0.));
#51087=CARTESIAN_POINT('Ctrl Pts',(12.8977690042853,-32.0066217236598,-32.0066217236598));
#51088=CARTESIAN_POINT('Ctrl Pts',(12.8977690042853,0.,-32.0066217236598));
#51089=CARTESIAN_POINT('Ctrl Pts',(12.8977690042853,32.0066217236598,-32.0066217236598));
#51090=CARTESIAN_POINT('Ctrl Pts',(12.8977690042853,32.0066217236598,0.));
#51091=CARTESIAN_POINT('Ctrl Pts',(11.9000549946031,32.7582360586468,0.));
#51092=CARTESIAN_POINT('Ctrl Pts',(11.9000549946031,32.7582360586468,32.7582360586468));
#51093=CARTESIAN_POINT('Ctrl Pts',(11.9000549946031,0.,32.7582360586468));
#51094=CARTESIAN_POINT('Ctrl Pts',(11.9000549946031,-32.7582360586468,32.7582360586468));
#51095=CARTESIAN_POINT('Ctrl Pts',(11.9000549946031,-32.7582360586468,0.));
#51096=CARTESIAN_POINT('Ctrl Pts',(11.9000549946031,-32.7582360586468,-32.7582360586468));
#51097=CARTESIAN_POINT('Ctrl Pts',(11.9000549946031,0.,-32.7582360586468));
#51098=CARTESIAN_POINT('Ctrl Pts',(11.9000549946031,32.7582360586468,-32.7582360586468));
#51099=CARTESIAN_POINT('Ctrl Pts',(11.9000549946031,32.7582360586468,0.));
#51100=CARTESIAN_POINT('Ctrl Pts',(10.9391333834985,33.5431303769822,0.));
#51101=CARTESIAN_POINT('Ctrl Pts',(10.9391333834985,33.5431303769822,33.5431303769822));
#51102=CARTESIAN_POINT('Ctrl Pts',(10.9391333834985,0.,33.5431303769822));
#51103=CARTESIAN_POINT('Ctrl Pts',(10.9391333834985,-33.5431303769822,33.5431303769822));
#51104=CARTESIAN_POINT('Ctrl Pts',(10.9391333834985,-33.5431303769822,0.));
#51105=CARTESIAN_POINT('Ctrl Pts',(10.9391333834985,-33.5431303769822,-33.5431303769822));
#51106=CARTESIAN_POINT('Ctrl Pts',(10.9391333834985,0.,-33.5431303769822));
#51107=CARTESIAN_POINT('Ctrl Pts',(10.9391333834985,33.5431303769822,-33.5431303769822));
#51108=CARTESIAN_POINT('Ctrl Pts',(10.9391333834985,33.5431303769822,0.));
#51109=CARTESIAN_POINT('Ctrl Pts',(10.0180552497783,34.3640644838406,0.));
#51110=CARTESIAN_POINT('Ctrl Pts',(10.0180552497783,34.3640644838406,34.3640644838406));
#51111=CARTESIAN_POINT('Ctrl Pts',(10.0180552497783,0.,34.3640644838406));
#51112=CARTESIAN_POINT('Ctrl Pts',(10.0180552497783,-34.3640644838406,34.3640644838406));
#51113=CARTESIAN_POINT('Ctrl Pts',(10.0180552497783,-34.3640644838406,0.));
#51114=CARTESIAN_POINT('Ctrl Pts',(10.0180552497783,-34.3640644838406,-34.3640644838406));
#51115=CARTESIAN_POINT('Ctrl Pts',(10.0180552497783,0.,-34.3640644838406));
#51116=CARTESIAN_POINT('Ctrl Pts',(10.0180552497783,34.3640644838406,-34.3640644838406));
#51117=CARTESIAN_POINT('Ctrl Pts',(10.0180552497783,34.3640644838406,0.));
#51118=CARTESIAN_POINT('Ctrl Pts',(9.13857394886632,35.2226243491956,0.));
#51119=CARTESIAN_POINT('Ctrl Pts',(9.13857394886632,35.2226243491956,35.2226243491956));
#51120=CARTESIAN_POINT('Ctrl Pts',(9.13857394886632,0.,35.2226243491956));
#51121=CARTESIAN_POINT('Ctrl Pts',(9.13857394886632,-35.2226243491956,35.2226243491956));
#51122=CARTESIAN_POINT('Ctrl Pts',(9.13857394886632,-35.2226243491956,0.));
#51123=CARTESIAN_POINT('Ctrl Pts',(9.13857394886632,-35.2226243491956,-35.2226243491956));
#51124=CARTESIAN_POINT('Ctrl Pts',(9.13857394886632,0.,-35.2226243491956));
#51125=CARTESIAN_POINT('Ctrl Pts',(9.13857394886632,35.2226243491956,-35.2226243491956));
#51126=CARTESIAN_POINT('Ctrl Pts',(9.13857394886632,35.2226243491956,0.));
#51127=CARTESIAN_POINT('Ctrl Pts',(8.29915429043693,36.1174213408745,0.));
#51128=CARTESIAN_POINT('Ctrl Pts',(8.29915429043693,36.1174213408745,36.1174213408745));
#51129=CARTESIAN_POINT('Ctrl Pts',(8.29915429043693,0.,36.1174213408745));
#51130=CARTESIAN_POINT('Ctrl Pts',(8.29915429043693,-36.1174213408745,36.1174213408745));
#51131=CARTESIAN_POINT('Ctrl Pts',(8.29915429043693,-36.1174213408745,0.));
#51132=CARTESIAN_POINT('Ctrl Pts',(8.29915429043693,-36.1174213408745,-36.1174213408745));
#51133=CARTESIAN_POINT('Ctrl Pts',(8.29915429043693,0.,-36.1174213408745));
#51134=CARTESIAN_POINT('Ctrl Pts',(8.29915429043693,36.1174213408745,-36.1174213408745));
#51135=CARTESIAN_POINT('Ctrl Pts',(8.29915429043693,36.1174213408745,0.));
#51136=CARTESIAN_POINT('Ctrl Pts',(7.4968190344241,37.0457624433751,0.));
#51137=CARTESIAN_POINT('Ctrl Pts',(7.4968190344241,37.0457624433751,37.0457624433751));
#51138=CARTESIAN_POINT('Ctrl Pts',(7.4968190344241,0.,37.0457624433751));
#51139=CARTESIAN_POINT('Ctrl Pts',(7.4968190344241,-37.0457624433751,37.0457624433751));
#51140=CARTESIAN_POINT('Ctrl Pts',(7.4968190344241,-37.0457624433751,0.));
#51141=CARTESIAN_POINT('Ctrl Pts',(7.4968190344241,-37.0457624433751,-37.0457624433751));
#51142=CARTESIAN_POINT('Ctrl Pts',(7.4968190344241,0.,-37.0457624433751));
#51143=CARTESIAN_POINT('Ctrl Pts',(7.4968190344241,37.0457624433751,-37.0457624433751));
#51144=CARTESIAN_POINT('Ctrl Pts',(7.4968190344241,37.0457624433751,0.));
#51145=CARTESIAN_POINT('Ctrl Pts',(6.88220761950379,37.8130900244198,0.));
#51146=CARTESIAN_POINT('Ctrl Pts',(6.88220761950379,37.8130900244197,37.8130900244197));
#51147=CARTESIAN_POINT('Ctrl Pts',(6.88220761950379,0.,37.8130900244198));
#51148=CARTESIAN_POINT('Ctrl Pts',(6.88220761950379,-37.8130900244197,37.8130900244197));
#51149=CARTESIAN_POINT('Ctrl Pts',(6.88220761950379,-37.8130900244198,0.));
#51150=CARTESIAN_POINT('Ctrl Pts',(6.88220761950379,-37.8130900244197,-37.8130900244197));
#51151=CARTESIAN_POINT('Ctrl Pts',(6.88220761950379,0.,-37.8130900244198));
#51152=CARTESIAN_POINT('Ctrl Pts',(6.88220761950379,37.8130900244197,-37.8130900244197));
#51153=CARTESIAN_POINT('Ctrl Pts',(6.88220761950379,37.8130900244198,0.));
#51154=CARTESIAN_POINT('Ctrl Pts',(6.43560997955544,38.4015756548256,0.));
#51155=CARTESIAN_POINT('Ctrl Pts',(6.43560997955544,38.4015756548256,38.4015756548256));
#51156=CARTESIAN_POINT('Ctrl Pts',(6.43560997955544,0.,38.4015756548256));
#51157=CARTESIAN_POINT('Ctrl Pts',(6.43560997955544,-38.4015756548256,38.4015756548256));
#51158=CARTESIAN_POINT('Ctrl Pts',(6.43560997955544,-38.4015756548256,0.));
#51159=CARTESIAN_POINT('Ctrl Pts',(6.43560997955544,-38.4015756548256,-38.4015756548256));
#51160=CARTESIAN_POINT('Ctrl Pts',(6.43560997955544,0.,-38.4015756548256));
#51161=CARTESIAN_POINT('Ctrl Pts',(6.43560997955544,38.4015756548256,-38.4015756548256));
#51162=CARTESIAN_POINT('Ctrl Pts',(6.43560997955544,38.4015756548256,0.));
#51163=CARTESIAN_POINT('Ctrl Pts',(6.14415685965718,38.7995786531943,0.));
#51164=CARTESIAN_POINT('Ctrl Pts',(6.14415685965718,38.7995786531942,38.7995786531942));
#51165=CARTESIAN_POINT('Ctrl Pts',(6.14415685965718,0.,38.7995786531943));
#51166=CARTESIAN_POINT('Ctrl Pts',(6.14415685965718,-38.7995786531942,38.7995786531942));
#51167=CARTESIAN_POINT('Ctrl Pts',(6.14415685965718,-38.7995786531943,0.));
#51168=CARTESIAN_POINT('Ctrl Pts',(6.14415685965718,-38.7995786531942,-38.7995786531942));
#51169=CARTESIAN_POINT('Ctrl Pts',(6.14415685965718,0.,-38.7995786531943));
#51170=CARTESIAN_POINT('Ctrl Pts',(6.14415685965718,38.7995786531942,-38.7995786531942));
#51171=CARTESIAN_POINT('Ctrl Pts',(6.14415685965718,38.7995786531943,0.));
#51172=CARTESIAN_POINT('Ctrl Pts',(6.,39.,0.));
#51173=CARTESIAN_POINT('Ctrl Pts',(6.,39.,39.));
#51174=CARTESIAN_POINT('Ctrl Pts',(6.,0.,39.));
#51175=CARTESIAN_POINT('Ctrl Pts',(6.,-39.,39.));
#51176=CARTESIAN_POINT('Ctrl Pts',(6.,-39.,0.));
#51177=CARTESIAN_POINT('Ctrl Pts',(6.,-39.,-39.));
#51178=CARTESIAN_POINT('Ctrl Pts',(6.,0.,-39.));
#51179=CARTESIAN_POINT('Ctrl Pts',(6.,39.,-39.));
#51180=CARTESIAN_POINT('Ctrl Pts',(6.,39.,0.));
#51181=CARTESIAN_POINT('Ctrl Pts',(15.,29.9016733813822,6.49999453793157));
#51182=CARTESIAN_POINT('Ctrl Pts',(14.0108432136945,30.1922309374725,8.0933373864441));
#51183=CARTESIAN_POINT('Ctrl Pts',(13.3692319443824,30.326239798997,9.13849504564574));
#51184=CARTESIAN_POINT('Ctrl Pts',(12.3476991724842,30.7091160415085,10.4190099465543));
#51185=CARTESIAN_POINT('Ctrl Pts',(12.0250187050191,30.8300585000507,10.8234973582048));
#51186=CARTESIAN_POINT('Ctrl Pts',(11.6666317570709,30.9698130949121,11.2708210236445));
#51187=CARTESIAN_POINT('Ctrl Pts',(11.3593868751765,31.1012032550439,11.6408078210926));
#51188=CARTESIAN_POINT('Ctrl Pts',(10.6767716809131,31.3931167252689,12.4628186160575));
#51189=CARTESIAN_POINT('Ctrl Pts',(10.1321636914396,31.6767647812522,13.0594869511698));
#51190=CARTESIAN_POINT('Ctrl Pts',(9.56604173138329,32.0598326220109,13.5737294275949));
#51191=CARTESIAN_POINT('Ctrl Pts',(9.34563078589187,32.2089742397651,13.7739418878736));
#51192=CARTESIAN_POINT('Ctrl Pts',(9.12222951098694,32.3737089207443,13.9612461574834));
#51193=CARTESIAN_POINT('Ctrl Pts',(8.88860711505277,32.5596655696803,14.1470079451216));
#51194=CARTESIAN_POINT('Ctrl Pts',(8.7583060070074,32.6633814711798,14.2506151642196));
#51195=CARTESIAN_POINT('Ctrl Pts',(8.62340343546547,32.7728839871607,14.3558447365466));
#51196=CARTESIAN_POINT('Ctrl Pts',(8.40819516300415,32.9604697380598,14.5166358456818));
#51197=CARTESIAN_POINT('Ctrl Pts',(8.02443006829124,33.2949776202952,14.8033628126358));
#51198=CARTESIAN_POINT('Ctrl Pts',(7.46417034513341,33.8242878903061,15.1962236527291));
#51199=CARTESIAN_POINT('Ctrl Pts',(6.85957019142019,34.4815104721779,15.6187306288434));
#51200=CARTESIAN_POINT('Ctrl Pts',(6.58024553736738,34.7851466343415,15.813928420662));
#51201=CARTESIAN_POINT('Ctrl Pts',(6.28976782192773,35.1265095516122,15.9958523276561));
#51202=CARTESIAN_POINT('Ctrl Pts',(6.,35.4893251315053,16.1712028529206));
#51203=CARTESIAN_POINT('Ctrl Pts',(2.09999999999999,14.6089664780085,6.03638282506164));
#51204=CARTESIAN_POINT('Ctrl Pts',(2.73333333333333,14.6089664780085,6.03638282506164));
#51205=CARTESIAN_POINT('Ctrl Pts',(3.36803666141114,14.6089514020126,6.03642739040373));
#51206=CARTESIAN_POINT('Ctrl Pts',(4.25277476731229,14.6089413613359,6.03645479962891));
#51207=CARTESIAN_POINT('Ctrl Pts',(4.77267392779604,14.60580914364,6.04427548151238));
#51208=CARTESIAN_POINT('Ctrl Pts',(5.76857452348673,14.5967723861308,6.06697519718139));
#51209=CARTESIAN_POINT('Ctrl Pts',(6.48509174407547,14.5970648927013,6.06638586537466));
#51210=CARTESIAN_POINT('Ctrl Pts',(6.99867014586152,14.6094270147457,6.03482055846387));
#51211=CARTESIAN_POINT('Ctrl Pts',(7.1248094424352,14.6126643615689,6.02686070999685));
#51212=CARTESIAN_POINT('Ctrl Pts',(7.37171227452388,14.6196411713314,6.01016358539879));
#51213=CARTESIAN_POINT('Ctrl Pts',(7.68212033066544,14.6296737194089,5.98681197306643));
#51214=CARTESIAN_POINT('Ctrl Pts',(8.05074799119104,14.6437937592098,5.95400947356552));
#51215=CARTESIAN_POINT('Ctrl Pts',(8.41504720380524,14.6600693966795,5.91546519208662));
#51216=CARTESIAN_POINT('Ctrl Pts',(9.01075539007779,14.6909192905048,5.83998490346081));
#51217=CARTESIAN_POINT('Ctrl Pts',(9.46310502651324,14.7214690610296,5.75973149002296));
#51218=CARTESIAN_POINT('Ctrl Pts',(10.2678550742082,14.7879867129576,5.569756534774));
#51219=CARTESIAN_POINT('Ctrl Pts',(10.9804987763497,14.8775467668719,5.33214922536331));
#51220=CARTESIAN_POINT('Ctrl Pts',(11.7910302654894,14.9989457804806,4.98237890778244));
#51221=CARTESIAN_POINT('Ctrl Pts',(12.2471584184909,15.0672903894667,4.76911662962923));
#51222=CARTESIAN_POINT('Ctrl Pts',(12.4732540604029,15.1001958841229,4.65911473846363));
#51223=CARTESIAN_POINT('Ctrl Pts',(12.8351237302837,15.1512383265106,4.48055499444762));
#51224=CARTESIAN_POINT('Ctrl Pts',(13.2802523785554,15.2185532647417,4.23828041374628));
#51225=CARTESIAN_POINT('Ctrl Pts',(14.1612572158898,15.3652875432003,3.68611012476648));
#51226=CARTESIAN_POINT('Ctrl Pts',(14.7820737708942,15.470296535549,3.22798797004085));
#51227=CARTESIAN_POINT('Ctrl Pts',(15.1979896574214,15.5282753821398,2.91077002204977));
#51228=CARTESIAN_POINT('Ctrl Pts',(2.09999999999999,21.5789877761254,9.39296817478263));
#51229=CARTESIAN_POINT('Ctrl Pts',(2.73333333333333,21.5789877761254,9.39296817478263));
#51230=CARTESIAN_POINT('Ctrl Pts',(3.36872402064119,21.5789856176355,9.39296797552278));
#51231=CARTESIAN_POINT('Ctrl Pts',(4.25416148268258,21.5789790511069,9.392979870206));
#51232=CARTESIAN_POINT('Ctrl Pts',(4.78310686396947,21.5740656337635,9.40460628784076));
#51233=CARTESIAN_POINT('Ctrl Pts',(5.7749467285248,21.5599997188704,9.43810307140346));
#51234=CARTESIAN_POINT('Ctrl Pts',(6.47498060646073,21.5606222109823,9.43679310319786));
#51235=CARTESIAN_POINT('Ctrl Pts',(6.96728310384879,21.5793773776101,9.39141943079971));
#51236=CARTESIAN_POINT('Ctrl Pts',(7.09310109124563,21.5844095945329,9.37968238548475));
#51237=CARTESIAN_POINT('Ctrl Pts',(7.33630061315444,21.5951630588673,9.35526265367197));
#51238=CARTESIAN_POINT('Ctrl Pts',(7.64237634935319,21.6106299965699,9.32107331035839));
#51239=CARTESIAN_POINT('Ctrl Pts',(8.00393183687127,21.6323236359645,9.2732461684707));
#51240=CARTESIAN_POINT('Ctrl Pts',(8.36002509556223,21.6573098677089,9.21712208992312));
#51241=CARTESIAN_POINT('Ctrl Pts',(8.93969220933936,21.7045540211068,9.10766060638776));
#51242=CARTESIAN_POINT('Ctrl Pts',(9.37530742884795,21.7512776632157,8.99163168810944));
#51243=CARTESIAN_POINT('Ctrl Pts',(10.1434139136649,21.8525564909802,8.71920853681163));
#51244=CARTESIAN_POINT('Ctrl Pts',(10.8343055464128,21.9900141967434,8.37636376802415));
#51245=CARTESIAN_POINT('Ctrl Pts',(11.6346923207873,22.1797979536336,7.864444884977));
#51246=CARTESIAN_POINT('Ctrl Pts',(12.0872652828465,22.2874582208771,7.55098281250724));
#51247=CARTESIAN_POINT('Ctrl Pts',(12.312256311387,22.339612685259,7.38883923970189));
#51248=CARTESIAN_POINT('Ctrl Pts',(12.6725939224516,22.4207763450689,7.12541325842979));
#51249=CARTESIAN_POINT('Ctrl Pts',(13.1110177472958,22.5275914879739,6.77118204758255));
#51250=CARTESIAN_POINT('Ctrl Pts',(13.9921364194962,22.7634712687919,5.95549963705341));
#51251=CARTESIAN_POINT('Ctrl Pts',(14.6125773377935,22.9346542951002,5.27532892793625));
#51252=CARTESIAN_POINT('Ctrl Pts',(15.0291266285127,23.0308726257289,4.80457770404129));
#51253=CARTESIAN_POINT('Ctrl Pts',(2.09999999999999,28.5490090742423,12.7495535245036));
#51254=CARTESIAN_POINT('Ctrl Pts',(2.73333333333333,28.5490090742423,12.7495535245036));
#51255=CARTESIAN_POINT('Ctrl Pts',(3.36945962045071,28.5489988659933,12.7495858434391));
#51256=CARTESIAN_POINT('Ctrl Pts',(4.25562677475033,28.548983910761,12.7496231050857));
#51257=CARTESIAN_POINT('Ctrl Pts',(4.79359981952435,28.5422019513635,12.7652539921132));
#51258=CARTESIAN_POINT('Ctrl Pts',(5.78147410742106,28.5231249848973,12.8095146599695));
#51259=CARTESIAN_POINT('Ctrl Pts',(6.46488413675066,28.5242644790789,12.807150202051));
#51260=CARTESIAN_POINT('Ctrl Pts',(6.93656514263953,28.5485127737679,12.7498643501742));
#51261=CARTESIAN_POINT('Ctrl Pts',(7.06207703364772,28.5553238593071,12.7343866375677));
#51262=CARTESIAN_POINT('Ctrl Pts',(7.30170817267462,28.5696861826432,12.7025998999942));
#51263=CARTESIAN_POINT('Ctrl Pts',(7.60368716963869,28.5903497015348,12.6580956050301));
#51264=CARTESIAN_POINT('Ctrl Pts',(7.95862452315423,28.6192058724396,12.5961222713689));
#51265=CARTESIAN_POINT('Ctrl Pts',(8.30733312679259,28.6523112124029,12.523726394015));
#51266=CARTESIAN_POINT('Ctrl Pts',(8.8731250253757,28.7147191108611,12.3829612054092));
#51267=CARTESIAN_POINT('Ctrl Pts',(9.29620381707367,28.7758759281063,12.2351772427441));
#51268=CARTESIAN_POINT('Ctrl Pts',(10.0462912732546,28.9085823331564,11.8884246619425));
#51269=CARTESIAN_POINT('Ctrl Pts',(10.740532795554,29.0943838012938,11.4407282263606));
#51270=CARTESIAN_POINT('Ctrl Pts',(11.5482388974608,29.3552929061951,10.7609358700024));
#51271=CARTESIAN_POINT('Ctrl Pts',(12.0041928460984,29.5034651889877,10.3446320328701));
#51272=CARTESIAN_POINT('Ctrl Pts',(12.230425106128,29.5753278301561,10.1293404338719));
#51273=CARTESIAN_POINT('Ctrl Pts',(12.5924623870156,29.6872159910832,9.77975755752727));
#51274=CARTESIAN_POINT('Ctrl Pts',(13.0427831926884,29.8375237688369,9.30259724740986));
#51275=CARTESIAN_POINT('Ctrl Pts',(13.9385931985019,30.1676318405281,8.20544467893018));
#51276=CARTESIAN_POINT('Ctrl Pts',(14.5670688438605,30.4064540621557,7.29435991172798));
#51277=CARTESIAN_POINT('Ctrl Pts',(14.9853697475044,30.5407333311124,6.66741354323698));
#51278=CARTESIAN_POINT('Ctrl Pts',(2.09999999999999,35.5190303723591,16.1061388742246));
#51279=CARTESIAN_POINT('Ctrl Pts',(2.73333333333333,35.5190303723591,16.1061388742246));
#51280=CARTESIAN_POINT('Ctrl Pts',(3.37021074703255,35.5190179918661,16.1061910341859));
#51281=CARTESIAN_POINT('Ctrl Pts',(4.25713143432193,35.5189972061824,16.1062482951899));
#51282=CARTESIAN_POINT('Ctrl Pts',(4.80403829546565,35.510266996621,16.1260480687564));
#51283=CARTESIAN_POINT('Ctrl Pts',(5.78815131161474,35.4862201834073,16.180988197307));
#51284=CARTESIAN_POINT('Ctrl Pts',(6.45447278497571,35.4880475600299,16.1772104845916));
#51285=CARTESIAN_POINT('Ctrl Pts',(6.90692970616558,35.5170694427124,16.1095128073425));
#51286=CARTESIAN_POINT('Ctrl Pts',(7.03216558775775,35.5256482290679,16.0903194135008));
#51287=CARTESIAN_POINT('Ctrl Pts',(7.26851607471023,35.5434898324498,16.0514394705235));
#51288=CARTESIAN_POINT('Ctrl Pts',(7.5668550388522,35.5691915200528,15.9969586081747));
#51289=CARTESIAN_POINT('Ctrl Pts',(7.91607160146964,35.6049494436263,15.9213993037407));
#51290=CARTESIAN_POINT('Ctrl Pts',(8.25886737580142,35.6458980270327,15.8333363661135));
#51291=CARTESIAN_POINT('Ctrl Pts',(8.81429360289333,35.723066410625,15.6621703423368));
#51292=CARTESIAN_POINT('Ctrl Pts',(9.23055663723524,35.7987202743156,15.4825835430176));
#51293=CARTESIAN_POINT('Ctrl Pts',(9.97651644615983,35.9658910107846,15.054823514641));
#51294=CARTESIAN_POINT('Ctrl Pts',(10.6790340006355,36.2049767460737,14.4905374879589));
#51295=CARTESIAN_POINT('Ctrl Pts',(11.4920994849111,36.5390136314546,13.6363007393238));
#51296=CARTESIAN_POINT('Ctrl Pts',(11.9504512738392,36.7283002504095,13.1145784039871));
#51297=CARTESIAN_POINT('Ctrl Pts',(12.1774805106591,36.8199606829071,12.8453218913326));
#51298=CARTESIAN_POINT('Ctrl Pts',(12.5406793815449,36.96265437758,12.4084300684841));
#51299=CARTESIAN_POINT('Ctrl Pts',(12.9976763399582,37.1577232826404,11.8030567245028));
#51300=CARTESIAN_POINT('Ctrl Pts',(13.8994020122616,37.5811368967158,10.4228391106914));
#51301=CARTESIAN_POINT('Ctrl Pts',(14.5324532885843,37.8867466021208,9.28021827726047));
#51302=CARTESIAN_POINT('Ctrl Pts',(14.9514110803021,38.0583529465017,8.49716491833391));
#51303=CARTESIAN_POINT('Ctrl Pts',(2.798152196741,35.1047471537606,15.9066502643122));
#51304=CARTESIAN_POINT('Ctrl Pts',(2.93286303103765,34.8223265530396,15.7706503227344));
#51305=CARTESIAN_POINT('Ctrl Pts',(3.06773152562602,34.5397254804734,15.6345646039347));
#51306=CARTESIAN_POINT('Ctrl Pts',(3.20258456668168,34.2572087160036,15.4985198290696));
#51307=CARTESIAN_POINT('Origin',(2.9,0.,0.));
#51308=CARTESIAN_POINT('Ctrl Pts',(3.19857191619793,37.5892075716104,0.899903760279396));
#51309=CARTESIAN_POINT('Ctrl Pts',(3.06444712372839,37.9029327677378,0.899921831100886));
#51310=CARTESIAN_POINT('Ctrl Pts',(2.93032447855964,38.2166010036509,0.899939693238254));
#51311=CARTESIAN_POINT('Ctrl Pts',(2.79631192480608,38.5299083490545,0.899954961404293));
#51312=CARTESIAN_POINT('Ctrl Pts',(2.09999999999998,6.75299193722314,-7.02449612538514));
#51313=CARTESIAN_POINT('Ctrl Pts',(2.73333333333332,6.75299193722314,-7.02449612538514));
#51314=CARTESIAN_POINT('Ctrl Pts',(3.36629680224277,6.75294648044154,-7.02452016539764));
#51315=CARTESIAN_POINT('Ctrl Pts',(4.12414743392493,6.75293267299237,-7.02452736897372));
#51316=CARTESIAN_POINT('Ctrl Pts',(4.36789509311751,6.75382103504332,-7.02368998068708));
#51317=CARTESIAN_POINT('Ctrl Pts',(4.86512395930617,6.75788793280844,-7.01986881358228));
#51318=CARTESIAN_POINT('Ctrl Pts',(5.74554025010893,6.76750052914464,-7.01085632454488));
#51319=CARTESIAN_POINT('Ctrl Pts',(6.51830366083575,6.76765825457168,-7.01071350589478));
#51320=CARTESIAN_POINT('Ctrl Pts',(7.10303189226247,6.75024197486783,-7.02690235429379));
#51321=CARTESIAN_POINT('Ctrl Pts',(7.23018703713608,6.7463685680123,-7.03058370260869));
#51322=CARTESIAN_POINT('Ctrl Pts',(7.42486685339525,6.74004512713713,-7.03670244791982));
#51323=CARTESIAN_POINT('Ctrl Pts',(7.6194364855123,6.73325250401511,-7.04336236931274));
#51324=CARTESIAN_POINT('Ctrl Pts',(8.01068306999147,6.71849387075291,-7.0579132628484));
#51325=CARTESIAN_POINT('Ctrl Pts',(8.60074918882448,6.69138911852921,-7.08463511606578));
#51326=CARTESIAN_POINT('Ctrl Pts',(9.25145738716207,6.64822816144239,-7.12531658480113));
#51327=CARTESIAN_POINT('Ctrl Pts',(9.76258194382415,6.60305748460113,-7.16601134101606));
#51328=CARTESIAN_POINT('Ctrl Pts',(10.0140805571163,6.57639478329963,-7.18937328759642));
#51329=CARTESIAN_POINT('Ctrl Pts',(10.7176652140345,6.49442351251533,-7.26012459111955));
#51330=CARTESIAN_POINT('Ctrl Pts',(11.8207747103308,6.31202427192381,-7.42265737436954));
#51331=CARTESIAN_POINT('Ctrl Pts',(12.8079604271039,6.07976122230612,-7.61409929856026));
#51332=CARTESIAN_POINT('Ctrl Pts',(13.5603806430126,5.88952590137785,-7.75631007302585));
#51333=CARTESIAN_POINT('Ctrl Pts',(14.1415267869189,5.72554047740206,-7.87660644726836));
#51334=CARTESIAN_POINT('Ctrl Pts',(15.2007169695464,5.37141982919035,-8.12566684501762));
#51335=CARTESIAN_POINT('Ctrl Pts',(15.9285176347281,5.07939082457031,-8.3118546564427));
#51336=CARTESIAN_POINT('Ctrl Pts',(16.6748049519623,4.76690229253182,-8.48846939426682));
#51337=CARTESIAN_POINT('Ctrl Pts',(17.2498356711401,4.50587852518841,-8.62929368175018));
#51338=CARTESIAN_POINT('Ctrl Pts',(18.2985117640075,3.9647261188096,-8.89613004054933));
#51339=CARTESIAN_POINT('Ctrl Pts',(19.0237320074819,3.53448198826109,-9.07450848842596));
#51340=CARTESIAN_POINT('Ctrl Pts',(19.7682744015967,3.07986955814412,-9.23156441073578));
#51341=CARTESIAN_POINT('Ctrl Pts',(20.3332383300351,2.7118628485122,-9.34724050739632));
#51342=CARTESIAN_POINT('Ctrl Pts',(21.372378830394,1.96371839940456,-9.54011298855374));
#51343=CARTESIAN_POINT('Ctrl Pts',(22.0963025405429,1.38682032165031,-9.63797649524687));
#51344=CARTESIAN_POINT('Ctrl Pts',(23.2302948553031,0.477375867824664,-9.72705857836219));
#51345=CARTESIAN_POINT('Ctrl Pts',(23.8854423668127,-0.0855090234660345,
-9.73358440568022));
#51346=CARTESIAN_POINT('Ctrl Pts',(24.5000000001022,-0.653978160206666,
-9.69209888135266));
#51347=CARTESIAN_POINT('Ctrl Pts',(2.09999999999998,9.36161601894518,-10.2956072597364));
#51348=CARTESIAN_POINT('Ctrl Pts',(2.73333333333332,9.36161601894518,-10.2956072597364));
#51349=CARTESIAN_POINT('Ctrl Pts',(3.36609438168516,9.36156585800923,-10.2956375248605));
#51350=CARTESIAN_POINT('Ctrl Pts',(4.12372361563831,9.36155092417073,-10.2956464147504));
#51351=CARTESIAN_POINT('Ctrl Pts',(4.36461784942786,9.36284448355378,-10.2944948929266));
#51352=CARTESIAN_POINT('Ctrl Pts',(4.85995591676349,9.36878888517195,-10.2892169831617));
#51353=CARTESIAN_POINT('Ctrl Pts',(5.74107832803173,9.38288286660015,-10.2767239120257));
#51354=CARTESIAN_POINT('Ctrl Pts',(6.52361564496404,9.38322607140847,-10.2764377689791));
#51355=CARTESIAN_POINT('Ctrl Pts',(7.11998100333695,9.35737516337016,-10.2991928575083));
#51356=CARTESIAN_POINT('Ctrl Pts',(7.24728410350207,9.35169382747716,-10.3042998764577));
#51357=CARTESIAN_POINT('Ctrl Pts',(7.4435678678656,9.34237505256982,-10.3128318292894));
#51358=CARTESIAN_POINT('Ctrl Pts',(7.63948101177056,9.33237103854479,-10.3221128622443));
#51359=CARTESIAN_POINT('Ctrl Pts',(8.0340967935931,9.31060889220749,-10.3424138549802));
#51360=CARTESIAN_POINT('Ctrl Pts',(8.63042364409642,9.27061026833392,-10.3797388678114));
#51361=CARTESIAN_POINT('Ctrl Pts',(9.29098306564,9.20676833650965,-10.4366867439073));
#51362=CARTESIAN_POINT('Ctrl Pts',(9.81197049062606,9.13980195102037,-10.4937819496382));
#51363=CARTESIAN_POINT('Ctrl Pts',(10.069143776842,9.1002104487285,-10.5266151541551));
#51364=CARTESIAN_POINT('Ctrl Pts',(10.7899979265155,8.97839988105312,-10.6261584553481));
#51365=CARTESIAN_POINT('Ctrl Pts',(11.9162899768689,8.70761596878294,-10.8543740998181));
#51366=CARTESIAN_POINT('Ctrl Pts',(12.9132370071959,8.36589560061933,-11.1201717547005));
#51367=CARTESIAN_POINT('Ctrl Pts',(13.6696754081786,8.08747451286091,-11.3161896788352));
#51368=CARTESIAN_POINT('Ctrl Pts',(14.2631204889818,7.84486957224345,-11.4840253590975));
#51369=CARTESIAN_POINT('Ctrl Pts',(15.3328909170884,7.32460265515443,-11.8280126795526));
#51370=CARTESIAN_POINT('Ctrl Pts',(16.0654084078213,6.89829469358604,-12.0827574614016));
#51371=CARTESIAN_POINT('Ctrl Pts',(16.8131418270019,6.44426633978414,-12.3219400191413));
#51372=CARTESIAN_POINT('Ctrl Pts',(17.3939906627799,6.06256663230004,-12.514066674993));
#51373=CARTESIAN_POINT('Ctrl Pts',(18.4452288839039,5.2762145869006,-12.8733663676658));
#51374=CARTESIAN_POINT('Ctrl Pts',(19.1721282346241,4.6539325222597,-13.1101502920758));
#51375=CARTESIAN_POINT('Ctrl Pts',(19.9175012294455,3.99789509083657,-13.3148682619423));
#51376=CARTESIAN_POINT('Ctrl Pts',(20.4827544940035,3.466823258858,-13.4651313654059));
#51377=CARTESIAN_POINT('Ctrl Pts',(21.519538834352,2.39128782352223,-13.7085532256609));
#51378=CARTESIAN_POINT('Ctrl Pts',(22.243410118146,1.5640378022019,-13.8238924709145));
#51379=CARTESIAN_POINT('Ctrl Pts',(23.3781373608504,0.261264463150115,-13.9119182156481));
#51380=CARTESIAN_POINT('Ctrl Pts',(24.0312127056184,-0.541258504051994,
-13.8980156514996));
#51381=CARTESIAN_POINT('Ctrl Pts',(24.6419825553303,-1.34841806297972,-13.8153739167048));
#51382=CARTESIAN_POINT('Ctrl Pts',(2.09999999999998,15.4484055429633,-17.9281999065559));
#51383=CARTESIAN_POINT('Ctrl Pts',(2.73333333333332,15.4484055429633,-17.9281999065559));
#51384=CARTESIAN_POINT('Ctrl Pts',(3.36560383820943,15.4482542660188,-17.9282842178703));
#51385=CARTESIAN_POINT('Ctrl Pts',(4.12271164892521,15.4482089930623,-17.9283090301052));
#51386=CARTESIAN_POINT('Ctrl Pts',(4.35694416238013,15.4504098665771,-17.9264523289363));
#51387=CARTESIAN_POINT('Ctrl Pts',(4.84788036531876,15.4606575463775,-17.9178309694623));
#51388=CARTESIAN_POINT('Ctrl Pts',(5.73060854685652,15.485197672036,-17.8972160956483));
#51389=CARTESIAN_POINT('Ctrl Pts',(6.53602142225768,15.4861289234307,-17.8964252059536));
#51390=CARTESIAN_POINT('Ctrl Pts',(7.15927193639697,15.4394328734173,-17.9354092414246));
#51391=CARTESIAN_POINT('Ctrl Pts',(7.28691515507382,15.4295142084321,-17.9438564347644));
#51392=CARTESIAN_POINT('Ctrl Pts',(7.48689772923258,15.41303282797,-17.9581538640174));
#51393=CARTESIAN_POINT('Ctrl Pts',(7.68589884468759,15.3953696129726,-17.9736779025854));
#51394=CARTESIAN_POINT('Ctrl Pts',(8.08824873453489,15.356840805821,-18.0077261400577));
#51395=CARTESIAN_POINT('Ctrl Pts',(8.69882087827138,15.2857078414599,-18.0705698025253));
#51396=CARTESIAN_POINT('Ctrl Pts',(9.38132108146395,15.1714461091176,-18.1670963317517));
#51397=CARTESIAN_POINT('Ctrl Pts',(9.92332887561784,15.0508171497738,-18.2645410332219));
#51398=CARTESIAN_POINT('Ctrl Pts',(10.1920703899024,14.9791813953041,-18.3208470995776));
#51399=CARTESIAN_POINT('Ctrl Pts',(10.9468728975028,14.7580401386903,-18.4921370629072));
#51400=CARTESIAN_POINT('Ctrl Pts',(12.1070803455683,14.2700737980981,-18.8807886500581));
#51401=CARTESIAN_POINT('Ctrl Pts',(13.1092903106678,13.669858687101,-19.3206148967827));
#51402=CARTESIAN_POINT('Ctrl Pts',(13.8683686220617,13.1837700651208,-19.6422817166552));
#51403=CARTESIAN_POINT('Ctrl Pts',(14.4658593195641,12.7565083867518,-19.9207911761091));
#51404=CARTESIAN_POINT('Ctrl Pts',(15.5292642023136,11.8549986940082,-20.4808296687727));
#51405=CARTESIAN_POINT('Ctrl Pts',(16.2562125089207,11.1195209746368,-20.8922494630454));
#51406=CARTESIAN_POINT('Ctrl Pts',(17.0019278536568,10.3355434884947,-21.2762452283177));
#51407=CARTESIAN_POINT('Ctrl Pts',(17.571102235943,9.68442584412187,-21.5819298232724));
#51408=CARTESIAN_POINT('Ctrl Pts',(18.6069001071236,8.34497393440998,-22.1498934640546));
#51409=CARTESIAN_POINT('Ctrl Pts',(19.324410136667,7.28445042254237,-22.5206154711307));
#51410=CARTESIAN_POINT('Ctrl Pts',(20.0667019463849,6.16093662590418,-22.8369405220828));
#51411=CARTESIAN_POINT('Ctrl Pts',(20.6168083009691,5.26926327642183,-23.0642318020815));
#51412=CARTESIAN_POINT('Ctrl Pts',(21.6393821249845,3.45112699200824,-23.4269677091127));
#51413=CARTESIAN_POINT('Ctrl Pts',(22.355423454672,2.04984247969421,-23.5861493055354));
#51414=CARTESIAN_POINT('Ctrl Pts',(23.4866230007993,-0.166763625493847,
-23.6784015849194));
#51415=CARTESIAN_POINT('Ctrl Pts',(24.1251264448473,-1.50769880146339,-23.6212865253562));
#51416=CARTESIAN_POINT('Ctrl Pts',(24.7275462447973,-2.86016104503983,-23.4511481200426));
#51417=CARTESIAN_POINT('Ctrl Pts',(2.09999999999998,21.5351950669813,-25.5607925533754));
#51418=CARTESIAN_POINT('Ctrl Pts',(2.73333333333332,21.5351950669813,-25.5607925533754));
#51419=CARTESIAN_POINT('Ctrl Pts',(3.36505757484791,21.5350703650623,-25.5608567667729));
#51420=CARTESIAN_POINT('Ctrl Pts',(4.12163108581741,21.5350353954978,-25.560873804661));
#51421=CARTESIAN_POINT('Ctrl Pts',(4.34918564951889,21.5380828728627,-25.5583623704001));
#51422=CARTESIAN_POINT('Ctrl Pts',(4.83578055685505,21.5525165407171,-25.5464973559168));
#51423=CARTESIAN_POINT('Ctrl Pts',(5.71990630918781,21.5875843019598,-25.5177015341715));
#51424=CARTESIAN_POINT('Ctrl Pts',(6.54861467977253,21.5899024265319,-25.5158130206185));
#51425=CARTESIAN_POINT('Ctrl Pts',(7.19737718820032,21.5199952205941,-25.572922103257));
#51426=CARTESIAN_POINT('Ctrl Pts',(7.32533517773902,21.5058054333461,-25.5847352647941));
#51427=CARTESIAN_POINT('Ctrl Pts',(7.5287921094654,21.4818075562725,-25.6050786014901));
#51428=CARTESIAN_POINT('Ctrl Pts',(7.73064555922848,21.4561637232329,-25.6270995800213));
#51429=CARTESIAN_POINT('Ctrl Pts',(8.14007691415316,21.4000011169923,-25.6755745536324));
#51430=CARTESIAN_POINT('Ctrl Pts',(8.76314309124191,21.2960181027815,-25.7653002467248));
#51431=CARTESIAN_POINT('Ctrl Pts',(9.4626157237208,21.1278957466071,-25.9040486107134));
#51432=CARTESIAN_POINT('Ctrl Pts',(10.0174850844879,20.9503131071729,-26.0442833898104));
#51433=CARTESIAN_POINT('Ctrl Pts',(10.2917439720134,20.8451238836403,-26.1251447081148));
#51434=CARTESIAN_POINT('Ctrl Pts',(11.0595344553679,20.5214871941961,-26.3704086438438));
#51435=CARTESIAN_POINT('Ctrl Pts',(12.2112380684354,19.8253512247695,-26.9121436740289));
#51436=CARTESIAN_POINT('Ctrl Pts',(13.2033849117556,18.9800507080956,-27.5171566231235));
#51437=CARTESIAN_POINT('Ctrl Pts',(13.9587773933514,18.2915509251392,-27.961398750055));
#51438=CARTESIAN_POINT('Ctrl Pts',(14.5428578718472,17.6981445922241,-28.3395188819555));
#51439=CARTESIAN_POINT('Ctrl Pts',(15.5916238649149,16.4391156082604,-29.1041678052385));
#51440=CARTESIAN_POINT('Ctrl Pts',(16.312400049336,15.4069402374363,-29.668803308567));
#51441=CARTESIAN_POINT('Ctrl Pts',(17.056455937744,14.2976159276549,-30.1984376782621));
#51442=CARTESIAN_POINT('Ctrl Pts',(17.6163953201452,13.3949790764644,-30.6123038825733));
#51443=CARTESIAN_POINT('Ctrl Pts',(18.6452863355316,11.5178862779835,-31.3895589768448));
#51444=CARTESIAN_POINT('Ctrl Pts',(19.3595097225576,10.0270239113276,-31.8973975158089));
#51445=CARTESIAN_POINT('Ctrl Pts',(20.1009956523856,8.43910743895403,-32.3304198138232));
#51446=CARTESIAN_POINT('Ctrl Pts',(20.6467087769493,7.19557321337572,-32.6373262144115));
#51447=CARTESIAN_POINT('Ctrl Pts',(21.6664645546449,4.63991827379282,-33.1285294116352));
#51448=CARTESIAN_POINT('Ctrl Pts',(22.3810936914814,2.66633276714268,-33.3391354765121));
#51449=CARTESIAN_POINT('Ctrl Pts',(23.5117886219139,-0.463686149823179,
-33.4478182016441));
#51450=CARTESIAN_POINT('Ctrl Pts',(24.1480627906507,-2.34324698531702,-33.355023097548));
#51451=CARTESIAN_POINT('Ctrl Pts',(24.7493903499091,-4.24322991552065,-33.1044542694871));
#51452=CARTESIAN_POINT('Ctrl Pts',(2.09999999999998,25.0133605092774,-29.9222740658437));
#51453=CARTESIAN_POINT('Ctrl Pts',(2.73333333333332,25.0133605092774,-29.9222740658437));
#51454=CARTESIAN_POINT('Ctrl Pts',(3.36472971107534,25.013251165713,-29.9223277377518));
#51455=CARTESIAN_POINT('Ctrl Pts',(4.12099543456558,25.0132219827751,-29.9223407668436));
#51456=CARTESIAN_POINT('Ctrl Pts',(4.34472654423455,25.0167312931454,-29.9194727333837));
#51457=CARTESIAN_POINT('Ctrl Pts',(4.82887687085582,25.0335070742804,-29.9057944106773));
#51458=CARTESIAN_POINT('Ctrl Pts',(5.71369265357388,25.0746209309229,-29.8722994997285));
#51459=CARTESIAN_POINT('Ctrl Pts',(6.55595753081649,25.0778849396657,-29.8696640285394));
#51460=CARTESIAN_POINT('Ctrl Pts',(7.21857014796824,24.9940353943491,-29.9376703562618));
#51461=CARTESIAN_POINT('Ctrl Pts',(7.34669496716987,24.9773954267909,-29.9514140474994));
#51462=CARTESIAN_POINT('Ctrl Pts',(7.55201908987345,24.9490050308752,-29.9752888612808));
#51463=CARTESIAN_POINT('Ctrl Pts',(7.75538136776272,24.9187155839832,-30.0010890760549));
#51464=CARTESIAN_POINT('Ctrl Pts',(8.16852342416032,24.852261565673,-30.0579755062707));
#51465=CARTESIAN_POINT('Ctrl Pts',(8.79787876017354,24.7290969956901,-30.1633810071747));
#51466=CARTESIAN_POINT('Ctrl Pts',(9.50485227440166,24.5297789011458,-30.3265656499729));
#51467=CARTESIAN_POINT('Ctrl Pts',(10.0642596293231,24.3199216659945,-30.4910276389621));
#51468=CARTESIAN_POINT('Ctrl Pts',(10.3399826652695,24.1960548694606,-30.5855364272996));
#51469=CARTESIAN_POINT('Ctrl Pts',(11.1101489081078,23.8160012772372,-30.871434727323));
#51470=CARTESIAN_POINT('Ctrl Pts',(12.2544520762226,23.0072865685853,-31.4960965077243));
#51471=CARTESIAN_POINT('Ctrl Pts',(13.2427910811612,22.0238011148559,-32.1947581271007));
#51472=CARTESIAN_POINT('Ctrl Pts',(13.9963706129132,21.2205661293469,-32.7087935562777));
#51473=CARTESIAN_POINT('Ctrl Pts',(14.5753869953058,20.5339755367801,-33.1430744875865));
#51474=CARTESIAN_POINT('Ctrl Pts',(15.6192748726438,19.0705105601026,-34.025466524286));
#51475=CARTESIAN_POINT('Ctrl Pts',(16.3374370627988,17.8688444541749,-34.678170573092));
#51476=CARTESIAN_POINT('Ctrl Pts',(17.0806842060506,16.573933856076,-35.2914329668221));
#51477=CARTESIAN_POINT('Ctrl Pts',(17.6370784162494,15.52656213101,-35.7679955458421));
#51478=CARTESIAN_POINT('Ctrl Pts',(18.6628686849426,13.3407406140021,-36.6661078330889));
#51479=CARTESIAN_POINT('Ctrl Pts',(19.3755242818045,11.6037884542861,-37.2528622744394));
#51480=CARTESIAN_POINT('Ctrl Pts',(20.1166807260025,9.75072239293528,-37.7530069912839));
#51481=CARTESIAN_POINT('Ctrl Pts',(20.6600607371703,8.30504525023832,-38.1060328053929));
#51482=CARTESIAN_POINT('Ctrl Pts',(21.6778468485764,5.32712143347218,-38.6712798616524));
#51483=CARTESIAN_POINT('Ctrl Pts',(22.3918418174935,3.02641427127417,-38.9118000510999));
#51484=CARTESIAN_POINT('Ctrl Pts',(23.5225304573588,-0.625454001463374,
-39.0305666347567));
#51485=CARTESIAN_POINT('Ctrl Pts',(24.157514841919,-2.81332401857134,-38.9179235041683));
#51486=CARTESIAN_POINT('Ctrl Pts',(24.7577717974218,-5.02641089220852,-38.6216026000469));
#51487=CARTESIAN_POINT('',(24.5,-0.653978160124863,-9.69209888145294));
#51488=CARTESIAN_POINT('Ctrl Pts',(24.5,-0.653978160124861,-9.69209888145294));
#51489=CARTESIAN_POINT('Ctrl Pts',(23.8274939346292,-0.0568713776825579,
-9.92072428837519));
#51490=CARTESIAN_POINT('Ctrl Pts',(23.3366347313518,0.36306026833911,-10.07387674794));
#51491=CARTESIAN_POINT('Ctrl Pts',(22.5855494187791,1.01440792710674,-10.3088927153609));
#51492=CARTESIAN_POINT('Ctrl Pts',(22.2454144272946,1.30937592429666,-10.4153215760233));
#51493=CARTESIAN_POINT('Ctrl Pts',(21.8382660744817,1.67447889633593,-10.5406724665088));
#51494=CARTESIAN_POINT('Ctrl Pts',(21.3802156950691,2.09338387047635,-10.6833058014315));
#51495=CARTESIAN_POINT('Ctrl Pts',(20.7694693293112,2.65193529200826,-10.8734874819961));
#51496=CARTESIAN_POINT('Ctrl Pts',(20.1629003033437,3.21491192658957,-11.0664040289027));
#51497=CARTESIAN_POINT('Ctrl Pts',(19.5574857571565,3.76869085487531,-11.2860183244349));
#51498=CARTESIAN_POINT('Ctrl Pts',(18.6418529411432,4.60622963346666,-11.6181643838934));
#51499=CARTESIAN_POINT('Ctrl Pts',(17.7734813312658,5.48886970291495,-11.9591596836358));
#51500=CARTESIAN_POINT('Ctrl Pts',(16.962125309523,6.31350499047669,-12.3453577907039));
#51501=CARTESIAN_POINT('Ctrl Pts',(16.8133360659434,6.46472943126141,-12.4161801210775));
#51502=CARTESIAN_POINT('Ctrl Pts',(16.665620536455,6.61523128891394,-12.4887778929881));
#51503=CARTESIAN_POINT('Ctrl Pts',(16.5183901926363,6.7654651816002,-12.5635998093483));
#51504=CARTESIAN_POINT('Ctrl Pts',(15.7264522886975,7.57355888693799,-12.9660597240242));
#51505=CARTESIAN_POINT('Ctrl Pts',(14.9462259719268,8.45630023657397,-13.3952652048773));
#51506=CARTESIAN_POINT('Ctrl Pts',(14.2963150414942,9.19178199464821,-13.806242544063));
#51507=CARTESIAN_POINT('Ctrl Pts',(13.990835093413,9.53748310344734,-13.9994156857325));
#51508=CARTESIAN_POINT('Ctrl Pts',(13.7077063566926,9.85948540296888,-14.1905588167449));
#51509=CARTESIAN_POINT('Ctrl Pts',(13.4460198946299,10.1567774063765,-14.377323000521));
#51510=CARTESIAN_POINT('Ctrl Pts',(12.8373295404644,10.8482872896864,-14.811741947042));
#51511=CARTESIAN_POINT('Ctrl Pts',(12.3530827408093,11.4368508716292,-15.185241342805));
#51512=CARTESIAN_POINT('Ctrl Pts',(11.9770275686809,11.8938113412781,-15.4929541616242));
#51513=CARTESIAN_POINT('Ctrl Pts',(11.6553972428173,12.2846378892233,-15.756133028781));
#51514=CARTESIAN_POINT('Ctrl Pts',(11.368420561492,12.6371055267151,-16.0048905246756));
#51515=CARTESIAN_POINT('Ctrl Pts',(11.0710856781083,13.0022863177644,-16.2795265088952));
#51516=CARTESIAN_POINT('Ctrl Pts',(10.8141787015496,13.31781435759,-16.5168209008521));
#51517=CARTESIAN_POINT('Ctrl Pts',(10.557680266175,13.633060973974,-16.766807974016));
#51518=CARTESIAN_POINT('Ctrl Pts',(10.2957959918397,13.9533753754527,-17.0392327535223));
#51519=CARTESIAN_POINT('Ctrl Pts',(9.71459276345166,14.6642533566189,-17.643828664231));
#51520=CARTESIAN_POINT('Ctrl Pts',(9.09527967376015,15.4163405024385,-18.3675428588812));
#51521=CARTESIAN_POINT('Ctrl Pts',(8.43168033652333,16.2610296723031,-19.2501379487015));
#51522=CARTESIAN_POINT('Ctrl Pts',(7.97964340480089,16.836423105025,-19.8513524978554));
#51523=CARTESIAN_POINT('Ctrl Pts',(7.52291961074422,17.4368467103674,-20.5091832448366));
#51524=CARTESIAN_POINT('Ctrl Pts',(7.10363554125516,18.0137184170276,-21.1546025206863));
#51525=CARTESIAN_POINT('Ctrl Pts',(6.56327799554033,18.7571689849997,-21.9863946187741));
#51526=CARTESIAN_POINT('Ctrl Pts',(6.08559840020807,19.4238605072403,-22.8142482171243));
#51527=CARTESIAN_POINT('Ctrl Pts',(5.61708670825923,20.1096693259461,-23.6903418871945));
#51528=CARTESIAN_POINT('Ctrl Pts',(5.04102956502001,20.9529034985418,-24.7675402270935));
#51529=CARTESIAN_POINT('Ctrl Pts',(4.50102820502495,21.7942496273475,-25.8856366973652));
#51530=CARTESIAN_POINT('Ctrl Pts',(4.00000000000001,22.6717457083367,-26.9859819793801));
#51531=CARTESIAN_POINT('Ctrl Pts',(3.72183418897161,23.1589226907791,-27.5968825927851));
#51532=CARTESIAN_POINT('Ctrl Pts',(3.45538353518261,23.6483861031357,-28.2106502986174));
#51533=CARTESIAN_POINT('Ctrl Pts',(3.2,24.1401481407882,-28.8273003894017));
#51534=CARTESIAN_POINT('',(24.5,-2.74456356862312,-26.8601446537018));
#51535=CARTESIAN_POINT('Ctrl Pts',(24.5,-2.74456356862309,-26.8601446537018));
#51536=CARTESIAN_POINT('Ctrl Pts',(24.5,-2.60355257661784,-25.6295076340102));
#51537=CARTESIAN_POINT('Ctrl Pts',(24.5,-2.46403488201538,-24.4198369473708));
#51538=CARTESIAN_POINT('Ctrl Pts',(24.5,-1.8827407509511,-19.4217612240443));
#51539=CARTESIAN_POINT('Ctrl Pts',(24.5,-1.25682129644897,-14.1166108279068));
#51540=CARTESIAN_POINT('Ctrl Pts',(24.5,-0.653978160124862,-9.69209888145293));
#51541=CARTESIAN_POINT('',(10.2670750393577,21.2938329649397,-26.7016219748491));
#51542=CARTESIAN_POINT('Ctrl Pts',(10.2670750393577,21.2938329649397,-26.7016219748491));
#51543=CARTESIAN_POINT('Ctrl Pts',(11.2293198185888,20.3809543843202,-26.3034024647587));
#51544=CARTESIAN_POINT('Ctrl Pts',(12.092802582344,19.4083234525969,-26.1769225550568));
#51545=CARTESIAN_POINT('Ctrl Pts',(14.3080979519049,16.7229516930375,-26.1226250533543));
#51546=CARTESIAN_POINT('Ctrl Pts',(14.8952017874601,15.9502790457014,-26.200370237811));
#51547=CARTESIAN_POINT('Ctrl Pts',(17.0803363586062,12.6346433376763,-26.6151103878942));
#51548=CARTESIAN_POINT('Ctrl Pts',(17.6922811489506,11.6274647466155,-26.7485362699767));
#51549=CARTESIAN_POINT('Ctrl Pts',(19.0755427322033,9.15735669344811,-27.067694655141));
#51550=CARTESIAN_POINT('Ctrl Pts',(20.2687424742408,6.9356814778935,-27.3229116595642));
#51551=CARTESIAN_POINT('Ctrl Pts',(22.3267279388309,2.40858489185046,-27.4185519724605));
#51552=CARTESIAN_POINT('Ctrl Pts',(23.4192562717209,-0.0469403629655241,
-27.32111731319));
#51553=CARTESIAN_POINT('Ctrl Pts',(24.5,-2.74456356862309,-26.8601446537018));
#51554=CARTESIAN_POINT('Ctrl Pts',(6.,25.0681110272506,-29.8762415562171));
#51555=CARTESIAN_POINT('Ctrl Pts',(7.51604047332548,23.7203706882541,-28.1913747515183));
#51556=CARTESIAN_POINT('Ctrl Pts',(9.08449301626627,22.3720336796495,-27.2810033999414));
#51557=CARTESIAN_POINT('Ctrl Pts',(9.8624969752411,21.6716883636697,-26.8795174907072));
#51558=CARTESIAN_POINT('Ctrl Pts',(10.0667253012217,21.4839041282495,-26.7845355705259));
#51559=CARTESIAN_POINT('Ctrl Pts',(10.2670750393577,21.2938329649397,-26.7016219748491));
#51560=CARTESIAN_POINT('Origin',(24.5,5.29966331579923,-6.64556760097826));
#51561=CARTESIAN_POINT('',(24.5,-3.12544889498789,-9.19761041611355));
#51562=CARTESIAN_POINT('Ctrl Pts',(24.5,-3.12544889498789,-9.19761041611355));
#51563=CARTESIAN_POINT('Ctrl Pts',(24.5,-2.86474614381472,-9.2862000702423));
#51564=CARTESIAN_POINT('Ctrl Pts',(24.5,-2.60012121793576,-9.36375841858885));
#51565=CARTESIAN_POINT('Ctrl Pts',(24.5,-1.78027869528961,-9.56652528394258));
#51566=CARTESIAN_POINT('Ctrl Pts',(24.5,-1.21867492867614,-9.65399574628659));
#51567=CARTESIAN_POINT('Ctrl Pts',(24.5,-0.653978160124863,-9.69209888145294));
#51568=CARTESIAN_POINT('',(24.5,-7.88307893260268,-25.8235757892348));
#51569=CARTESIAN_POINT('Ctrl Pts',(24.5,-3.12544889498789,-9.19761041611355));
#51570=CARTESIAN_POINT('Ctrl Pts',(24.5,-4.24788855647684,-13.3567531368014));
#51571=CARTESIAN_POINT('Ctrl Pts',(24.5,-5.84332298292785,-18.8793734697304));
#51572=CARTESIAN_POINT('Ctrl Pts',(24.5,-7.88307893260268,-25.8235757892348));
#51573=CARTESIAN_POINT('Origin',(24.5,0.,0.));
#51574=CARTESIAN_POINT('Ctrl Pts',(24.5,-7.88307920268519,-25.8235757067876));
#51575=CARTESIAN_POINT('Ctrl Pts',(24.5,5.71692116672878,-29.9752037108234));
#51576=CARTESIAN_POINT('Ctrl Pts',(24.5,16.8342246501858,-21.1094500266368));
#51577=CARTESIAN_POINT('Ctrl Pts',(24.5,37.9436746768226,-4.27522537645101));
#51578=CARTESIAN_POINT('Ctrl Pts',(24.5,21.1094500266368,16.8342246501858));
#51579=CARTESIAN_POINT('Ctrl Pts',(24.5,4.27522537645101,37.9436746768226));
#51580=CARTESIAN_POINT('Ctrl Pts',(24.5,-16.8342246501858,21.1094500266368));
#51581=CARTESIAN_POINT('Ctrl Pts',(24.5,-37.9436746768226,4.27522537645101));
#51582=CARTESIAN_POINT('Ctrl Pts',(24.5,-21.1094500266368,-16.8342246501858));
#51583=CARTESIAN_POINT('Ctrl Pts',(24.5,-15.8898724606626,-23.3793678972715));
#51584=CARTESIAN_POINT('Ctrl Pts',(24.5,-7.88307920268519,-25.8235757067876));
#51585=CARTESIAN_POINT('Ctrl Pts',(24.3078118955742,-7.89265172758991,-25.8549336083419));
#51586=CARTESIAN_POINT('Ctrl Pts',(24.3078118955742,5.72386329794929,-30.0116029878912));
#51587=CARTESIAN_POINT('Ctrl Pts',(24.3078118955742,16.8546666666329,-21.1350835044834));
#51588=CARTESIAN_POINT('Ctrl Pts',(24.3078118955742,37.9897501711163,-4.28041683785043));
#51589=CARTESIAN_POINT('Ctrl Pts',(24.3078118955742,21.1350835044834,16.8546666666329));
#51590=CARTESIAN_POINT('Ctrl Pts',(24.3078118955742,4.28041683785043,37.9897501711163));
#51591=CARTESIAN_POINT('Ctrl Pts',(24.3078118955742,-16.8546666666329,21.1350835044834));
#51592=CARTESIAN_POINT('Ctrl Pts',(24.3078118955742,-37.9897501711163,4.28041683785043));
#51593=CARTESIAN_POINT('Ctrl Pts',(24.3078118955742,-21.1350835044834,-16.8546666666329));
#51594=CARTESIAN_POINT('Ctrl Pts',(24.3078118955742,-15.9091677380474,-23.4077577657098));
#51595=CARTESIAN_POINT('Ctrl Pts',(24.3078118955742,-7.89265172758991,-25.8549336083419));
#51596=CARTESIAN_POINT('Ctrl Pts',(23.9225830034177,-7.91301273816933,-25.9216326842544));
#51597=CARTESIAN_POINT('Ctrl Pts',(23.9225830034177,5.73862939243657,-30.0890252012401));
#51598=CARTESIAN_POINT('Ctrl Pts',(23.9225830034177,16.8981473697169,-21.1896065816043));
#51599=CARTESIAN_POINT('Ctrl Pts',(23.9225830034177,38.0877539513211,-4.29145921188743));
#51600=CARTESIAN_POINT('Ctrl Pts',(23.9225830034177,21.1896065816043,16.8981473697169));
#51601=CARTESIAN_POINT('Ctrl Pts',(23.9225830034177,4.29145921188743,38.0877539513211));
#51602=CARTESIAN_POINT('Ctrl Pts',(23.9225830034177,-16.8981473697169,21.1896065816043));
#51603=CARTESIAN_POINT('Ctrl Pts',(23.9225830034177,-38.0877539513211,4.29145921188743));
#51604=CARTESIAN_POINT('Ctrl Pts',(23.9225830034177,-21.1896065816043,-16.8981473697169));
#51605=CARTESIAN_POINT('Ctrl Pts',(23.9225830034177,-15.9502092971843,-23.4681437576372));
#51606=CARTESIAN_POINT('Ctrl Pts',(23.9225830034177,-7.91301273816933,-25.9216326842544));
#51607=CARTESIAN_POINT('Ctrl Pts',(23.3421815947946,-7.9472021240383,-26.0336310762095));
#51608=CARTESIAN_POINT('Ctrl Pts',(23.3421815947946,5.76342402137866,-30.2190294520944));
#51609=CARTESIAN_POINT('Ctrl Pts',(23.3421815947946,16.9711584086233,-21.2811595286045));
#51610=CARTESIAN_POINT('Ctrl Pts',(23.3421815947946,38.2523179372279,-4.31000111998122));
#51611=CARTESIAN_POINT('Ctrl Pts',(23.3421815947946,21.2811595286045,16.9711584086233));
#51612=CARTESIAN_POINT('Ctrl Pts',(23.3421815947946,4.31000111998122,38.2523179372279));
#51613=CARTESIAN_POINT('Ctrl Pts',(23.3421815947946,-16.9711584086233,21.2811595286045));
#51614=CARTESIAN_POINT('Ctrl Pts',(23.3421815947946,-38.2523179372279,4.31000111998122));
#51615=CARTESIAN_POINT('Ctrl Pts',(23.3421815947946,-21.2811595286045,-16.9711584086233));
#51616=CARTESIAN_POINT('Ctrl Pts',(23.3421815947946,-16.0191246241775,-23.5695414741716));
#51617=CARTESIAN_POINT('Ctrl Pts',(23.3421815947946,-7.9472021240383,-26.0336310762095));
#51618=CARTESIAN_POINT('Ctrl Pts',(22.5631762070947,-8.00011358475547,-26.2069596799766));
#51619=CARTESIAN_POINT('Ctrl Pts',(22.5631762070947,5.80179616530353,-30.4202239057914));
#51620=CARTESIAN_POINT('Ctrl Pts',(22.5631762070947,17.0841502222764,-21.4228467814061));
#51621=CARTESIAN_POINT('Ctrl Pts',(22.5631762070947,38.5069970036825,-4.33869655912968));
#51622=CARTESIAN_POINT('Ctrl Pts',(22.5631762070947,21.4228467814061,17.0841502222764));
#51623=CARTESIAN_POINT('Ctrl Pts',(22.5631762070947,4.33869655912968,38.5069970036825));
#51624=CARTESIAN_POINT('Ctrl Pts',(22.5631762070947,-17.0841502222764,21.4228467814061));
#51625=CARTESIAN_POINT('Ctrl Pts',(22.5631762070947,-38.5069970036825,4.33869655912968));
#51626=CARTESIAN_POINT('Ctrl Pts',(22.5631762070947,-21.4228467814061,-17.0841502222764));
#51627=CARTESIAN_POINT('Ctrl Pts',(22.5631762070947,-16.1257779180092,-23.7264644828441));
#51628=CARTESIAN_POINT('Ctrl Pts',(22.5631762070947,-8.00011358475547,-26.2069596799766));
#51629=CARTESIAN_POINT('Ctrl Pts',(21.5808622776984,-8.07867607201863,-26.4643165180079));
#51630=CARTESIAN_POINT('Ctrl Pts',(21.5808622776984,5.85877079853982,-30.7189557210115));
#51631=CARTESIAN_POINT('Ctrl Pts',(21.5808622776984,17.2519195070522,-21.633222810393));
#51632=CARTESIAN_POINT('Ctrl Pts',(21.5808622776984,38.8851423174451,-4.38130330334077));
#51633=CARTESIAN_POINT('Ctrl Pts',(21.5808622776984,21.633222810393,17.2519195070522));
#51634=CARTESIAN_POINT('Ctrl Pts',(21.5808622776984,4.38130330334077,38.8851423174451));
#51635=CARTESIAN_POINT('Ctrl Pts',(21.5808622776984,-17.2519195070522,21.633222810393));
#51636=CARTESIAN_POINT('Ctrl Pts',(21.5808622776984,-38.8851423174451,4.38130330334077));
#51637=CARTESIAN_POINT('Ctrl Pts',(21.5808622776984,-21.633222810393,-17.2519195070522));
#51638=CARTESIAN_POINT('Ctrl Pts',(21.5808622776984,-16.2841358224153,-23.9594624326839));
#51639=CARTESIAN_POINT('Ctrl Pts',(21.5808622776984,-8.07867607201863,-26.4643165180079));
#51640=CARTESIAN_POINT('Ctrl Pts',(20.5902243197586,-8.16999801768733,-26.7634710890877));
#51641=CARTESIAN_POINT('Ctrl Pts',(20.5902243197586,5.92499877250238,-31.0662050450771));
#51642=CARTESIAN_POINT('Ctrl Pts',(20.5902243197586,17.4469364679823,-21.8777663445708));
#51643=CARTESIAN_POINT('Ctrl Pts',(20.5902243197586,39.3247028125531,-4.43082987658853));
#51644=CARTESIAN_POINT('Ctrl Pts',(20.5902243197586,21.8777663445708,17.4469364679823));
#51645=CARTESIAN_POINT('Ctrl Pts',(20.5902243197586,4.43082987658853,39.3247028125531));
#51646=CARTESIAN_POINT('Ctrl Pts',(20.5902243197586,-17.4469364679823,21.8777663445708));
#51647=CARTESIAN_POINT('Ctrl Pts',(20.5902243197586,-39.3247028125531,4.43082987658853));
#51648=CARTESIAN_POINT('Ctrl Pts',(20.5902243197586,-21.8777663445708,-17.4469364679823));
#51649=CARTESIAN_POINT('Ctrl Pts',(20.5902243197586,-16.4682128857335,-24.2303019498304));
#51650=CARTESIAN_POINT('Ctrl Pts',(20.5902243197586,-8.16999801768733,-26.7634710890877));
#51651=CARTESIAN_POINT('Ctrl Pts',(19.591895069338,-8.27451080226189,-27.1058365195744));
#51652=CARTESIAN_POINT('Ctrl Pts',(19.591895069338,6.000792930466,-31.4636121911249));
#51653=CARTESIAN_POINT('Ctrl Pts',(19.591895069338,17.6701223131461,-22.157632542334));
#51654=CARTESIAN_POINT('Ctrl Pts',(19.591895069338,39.8277548554801,-4.48751022918787));
#51655=CARTESIAN_POINT('Ctrl Pts',(19.591895069338,22.157632542334,17.6701223131461));
#51656=CARTESIAN_POINT('Ctrl Pts',(19.591895069338,4.48751022918787,39.8277548554801));
#51657=CARTESIAN_POINT('Ctrl Pts',(19.591895069338,-17.6701223131461,22.157632542334));
#51658=CARTESIAN_POINT('Ctrl Pts',(19.591895069338,-39.8277548554801,4.48751022918787));
#51659=CARTESIAN_POINT('Ctrl Pts',(19.591895069338,-22.157632542334,-17.6701223131461));
#51660=CARTESIAN_POINT('Ctrl Pts',(19.591895069338,-16.6788786388865,-24.540262407884));
#51661=CARTESIAN_POINT('Ctrl Pts',(19.591895069338,-8.27451080226189,-27.1058365195744));
#51662=CARTESIAN_POINT('Ctrl Pts',(18.5871162949016,-8.39271031247285,-27.4930372468484));
#51663=CARTESIAN_POINT('Ctrl Pts',(18.5871162949016,6.08651289654117,-31.9130627555549));
#51664=CARTESIAN_POINT('Ctrl Pts',(18.5871162949016,17.9225360029332,-22.47414929801));
#51665=CARTESIAN_POINT('Ctrl Pts',(18.5871162949016,40.3966853009432,-4.55161329507688));
#51666=CARTESIAN_POINT('Ctrl Pts',(18.5871162949016,22.47414929801,17.9225360029332));
#51667=CARTESIAN_POINT('Ctrl Pts',(18.5871162949016,4.55161329507688,40.3966853009432));
#51668=CARTESIAN_POINT('Ctrl Pts',(18.5871162949016,-17.9225360029332,22.47414929801));
#51669=CARTESIAN_POINT('Ctrl Pts',(18.5871162949016,-40.3966853009432,4.55161329507688));
#51670=CARTESIAN_POINT('Ctrl Pts',(18.5871162949016,-22.47414929801,-17.9225360029332));
#51671=CARTESIAN_POINT('Ctrl Pts',(18.5871162949016,-16.9171326375936,-24.8908144908262));
#51672=CARTESIAN_POINT('Ctrl Pts',(18.5871162949016,-8.39271031247285,-27.4930372468484));
#51673=CARTESIAN_POINT('Ctrl Pts',(17.577868433379,-8.52509880948018,-27.9267185897952));
#51674=CARTESIAN_POINT('Ctrl Pts',(17.577868433379,6.18252291766525,-32.4164665733692));
#51675=CARTESIAN_POINT('Ctrl Pts',(17.577868433379,18.2052501102534,-22.8286615754873));
#51676=CARTESIAN_POINT('Ctrl Pts',(17.577868433379,41.0339116857407,-4.62341146523394));
#51677=CARTESIAN_POINT('Ctrl Pts',(17.577868433379,22.8286615754873,18.2052501102534));
#51678=CARTESIAN_POINT('Ctrl Pts',(17.577868433379,4.62341146523394,41.0339116857407));
#51679=CARTESIAN_POINT('Ctrl Pts',(17.577868433379,-18.2052501102534,22.8286615754873));
#51680=CARTESIAN_POINT('Ctrl Pts',(17.577868433379,-41.0339116857407,4.62341146523394));
#51681=CARTESIAN_POINT('Ctrl Pts',(17.577868433379,-22.8286615754873,-18.2052501102534));
#51682=CARTESIAN_POINT('Ctrl Pts',(17.577868433379,-17.1839872864711,-25.2834477877042));
#51683=CARTESIAN_POINT('Ctrl Pts',(17.577868433379,-8.52509880948018,-27.9267185897952));
#51684=CARTESIAN_POINT('Ctrl Pts',(16.5668667015923,-8.67209622266927,-28.4082561629427));
#51685=CARTESIAN_POINT('Ctrl Pts',(16.5668667015923,6.28912753260161,-32.9754204151378));
#51686=CARTESIAN_POINT('Ctrl Pts',(16.5668667015923,18.5191613894625,-23.2222938691605));
#51687=CARTESIAN_POINT('Ctrl Pts',(16.5668667015923,41.7414552586229,-4.703132479698));
#51688=CARTESIAN_POINT('Ctrl Pts',(16.5668667015923,23.2222938691605,18.5191613894625));
#51689=CARTESIAN_POINT('Ctrl Pts',(16.5668667015923,4.703132479698,41.7414552586229));
#51690=CARTESIAN_POINT('Ctrl Pts',(16.5668667015923,-18.5191613894625,23.2222938691605));
#51691=CARTESIAN_POINT('Ctrl Pts',(16.5668667015923,-41.7414552586229,4.703132479698));
#51692=CARTESIAN_POINT('Ctrl Pts',(16.5668667015923,-23.2222938691605,-18.5191613894625));
#51693=CARTESIAN_POINT('Ctrl Pts',(16.5668667015923,-17.480289034502,-25.7194077107917));
#51694=CARTESIAN_POINT('Ctrl Pts',(16.5668667015923,-8.67209622266927,-28.4082561629427));
#51695=CARTESIAN_POINT('Ctrl Pts',(15.5576189940876,-8.83393595783092,-28.9384145624536));
#51696=CARTESIAN_POINT('Ctrl Pts',(15.5576189940876,6.40649601054971,-33.5908118003118));
#51697=CARTESIAN_POINT('Ctrl Pts',(15.5576189940876,18.8647682759327,-23.6556711972172));
#51698=CARTESIAN_POINT('Ctrl Pts',(15.5576189940876,42.5204394731498,-4.79090292128453));
#51699=CARTESIAN_POINT('Ctrl Pts',(15.5576189940876,23.6556711972172,18.8647682759327));
#51700=CARTESIAN_POINT('Ctrl Pts',(15.5576189940876,4.79090292128453,42.5204394731498));
#51701=CARTESIAN_POINT('Ctrl Pts',(15.5576189940876,-18.8647682759327,23.6556711972172));
#51702=CARTESIAN_POINT('Ctrl Pts',(15.5576189940876,-42.5204394731498,4.79090292128453));
#51703=CARTESIAN_POINT('Ctrl Pts',(15.5576189940876,-23.6556711972172,-18.8647682759327));
#51704=CARTESIAN_POINT('Ctrl Pts',(15.5576189940876,-17.80650835625,-26.1993864870359));
#51705=CARTESIAN_POINT('Ctrl Pts',(15.5576189940876,-8.83393595783092,-28.9384145624536));
#51706=CARTESIAN_POINT('Ctrl Pts',(14.5544447688713,-9.01056601144323,-29.5170234339714));
#51707=CARTESIAN_POINT('Ctrl Pts',(14.5544447688713,6.53459063781575,-34.262442986851));
#51708=CARTESIAN_POINT('Ctrl Pts',(14.5544447688713,19.2419597167431,-24.1286543036994));
#51709=CARTESIAN_POINT('Ctrl Pts',(14.5544447688713,43.3706140204425,-4.88669458695624));
#51710=CARTESIAN_POINT('Ctrl Pts',(14.5544447688713,24.1286543036994,19.2419597167431));
#51711=CARTESIAN_POINT('Ctrl Pts',(14.5544447688713,4.88669458695624,43.3706140204425));
#51712=CARTESIAN_POINT('Ctrl Pts',(14.5544447688713,-19.2419597167431,24.1286543036994));
#51713=CARTESIAN_POINT('Ctrl Pts',(14.5544447688713,-43.3706140204425,4.88669458695624));
#51714=CARTESIAN_POINT('Ctrl Pts',(14.5544447688713,-24.1286543036994,-19.2419597167431));
#51715=CARTESIAN_POINT('Ctrl Pts',(14.5544447688713,-18.1625404285478,-26.7232298861623));
#51716=CARTESIAN_POINT('Ctrl Pts',(14.5544447688713,-9.01056601144323,-29.5170234339714));
#51717=CARTESIAN_POINT('Ctrl Pts',(13.5625963827217,-9.20148423244017,-30.1424378192589));
#51718=CARTESIAN_POINT('Ctrl Pts',(13.5625963827217,6.67304724730406,-34.9884045583829));
#51719=CARTESIAN_POINT('Ctrl Pts',(13.5625963827217,19.6496633740883,-24.6398985195302));
#51720=CARTESIAN_POINT('Ctrl Pts',(13.5625963827217,44.2895618936185,-4.99023514544194));
#51721=CARTESIAN_POINT('Ctrl Pts',(13.5625963827217,24.6398985195302,19.6496633740883));
#51722=CARTESIAN_POINT('Ctrl Pts',(13.5625963827217,4.99023514544194,44.2895618936185));
#51723=CARTESIAN_POINT('Ctrl Pts',(13.5625963827217,-19.6496633740883,24.6398985195302));
#51724=CARTESIAN_POINT('Ctrl Pts',(13.5625963827217,-44.2895618936185,4.99023514544194));
#51725=CARTESIAN_POINT('Ctrl Pts',(13.5625963827217,-24.6398985195302,-19.6496633740883));
#51726=CARTESIAN_POINT('Ctrl Pts',(13.5625963827217,-18.5473730686949,-27.2894486456364));
#51727=CARTESIAN_POINT('Ctrl Pts',(13.5625963827217,-9.20148423244017,-30.1424378192589));
#51728=CARTESIAN_POINT('Ctrl Pts',(12.5880795783847,-9.40573585110567,-30.8115300612911));
#51729=CARTESIAN_POINT('Ctrl Pts',(12.5880795783847,6.82117342643589,-35.7650660278856));
#51730=CARTESIAN_POINT('Ctrl Pts',(12.5880795783847,20.0858403482595,-25.1868471453426));
#51731=CARTESIAN_POINT('Ctrl Pts',(12.5880795783847,45.2726874936021,-5.10100679708315));
#51732=CARTESIAN_POINT('Ctrl Pts',(12.5880795783847,25.1868471453426,20.0858403482595));
#51733=CARTESIAN_POINT('Ctrl Pts',(12.5880795783847,5.10100679708315,45.2726874936021));
#51734=CARTESIAN_POINT('Ctrl Pts',(12.5880795783847,-20.0858403482595,25.1868471453426));
#51735=CARTESIAN_POINT('Ctrl Pts',(12.5880795783847,-45.2726874936021,5.10100679708315));
#51736=CARTESIAN_POINT('Ctrl Pts',(12.5880795783847,-25.1868471453426,-20.0858403482595));
#51737=CARTESIAN_POINT('Ctrl Pts',(12.5880795783847,-18.9590817534653,-27.895211141942));
#51738=CARTESIAN_POINT('Ctrl Pts',(12.5880795783847,-9.40573585110567,-30.8115300612911));
#51739=CARTESIAN_POINT('Ctrl Pts',(11.6370973936883,-9.62212179125491,-31.5203721981841));
#51740=CARTESIAN_POINT('Ctrl Pts',(11.6370973936883,6.97809958810636,-36.587867939342));
#51741=CARTESIAN_POINT('Ctrl Pts',(11.6370973936883,20.5479300259039,-25.766289273552));
#51742=CARTESIAN_POINT('Ctrl Pts',(11.6370973936883,46.3142192994558,-5.21835924764817));
#51743=CARTESIAN_POINT('Ctrl Pts',(11.6370973936883,25.766289273552,20.5479300259039));
#51744=CARTESIAN_POINT('Ctrl Pts',(11.6370973936883,5.21835924764817,46.3142192994558));
#51745=CARTESIAN_POINT('Ctrl Pts',(11.6370973936883,-20.5479300259039,25.766289273552));
#51746=CARTESIAN_POINT('Ctrl Pts',(11.6370973936883,-46.3142192994558,5.21835924764817));
#51747=CARTESIAN_POINT('Ctrl Pts',(11.6370973936883,-25.766289273552,-20.5479300259039));
#51748=CARTESIAN_POINT('Ctrl Pts',(11.6370973936883,-19.3952495126426,-28.5369611957563));
#51749=CARTESIAN_POINT('Ctrl Pts',(11.6370973936883,-9.62212179125491,-31.5203721981841));
#51750=CARTESIAN_POINT('Ctrl Pts',(10.7155646400367,-9.84933794718583,-32.2646922098985));
#51751=CARTESIAN_POINT('Ctrl Pts',(10.7155646400367,7.14287997631073,-37.4518514647263));
#51752=CARTESIAN_POINT('Ctrl Pts',(10.7155646400367,21.0331475043468,-26.3747327466602));
#51753=CARTESIAN_POINT('Ctrl Pts',(10.7155646400367,47.4078802510069,-5.34158524231338));
#51754=CARTESIAN_POINT('Ctrl Pts',(10.7155646400367,26.3747327466602,21.0331475043468));
#51755=CARTESIAN_POINT('Ctrl Pts',(10.7155646400367,5.34158524231338,47.4078802510069));
#51756=CARTESIAN_POINT('Ctrl Pts',(10.7155646400367,-21.0331475043468,26.3747327466602));
#51757=CARTESIAN_POINT('Ctrl Pts',(10.7155646400367,-47.4078802510069,5.34158524231338));
#51758=CARTESIAN_POINT('Ctrl Pts',(10.7155646400367,-26.3747327466602,-21.0331475043468));
#51759=CARTESIAN_POINT('Ctrl Pts',(10.7155646400367,-19.8532476686822,-29.2108311347902));
#51760=CARTESIAN_POINT('Ctrl Pts',(10.7155646400367,-9.84933794718583,-32.2646922098985));
#51761=CARTESIAN_POINT('Ctrl Pts',(9.82859575068344,-10.0861224473418,-33.0403564279984));
#51762=CARTESIAN_POINT('Ctrl Pts',(9.82859575068344,7.31459946384724,-38.3522183702525));
#51763=CARTESIAN_POINT('Ctrl Pts',(9.82859575068344,21.5387980714436,-27.0087985025163));
#51764=CARTESIAN_POINT('Ctrl Pts',(9.82859575068344,48.5475965739599,-5.47000043107263));
#51765=CARTESIAN_POINT('Ctrl Pts',(9.82859575068344,27.0087985025163,21.5387980714436));
#51766=CARTESIAN_POINT('Ctrl Pts',(9.82859575068344,5.47000043107263,48.5475965739599));
#51767=CARTESIAN_POINT('Ctrl Pts',(9.82859575068344,-21.5387980714436,27.0087985025163));
#51768=CARTESIAN_POINT('Ctrl Pts',(9.82859575068344,-48.5475965739599,5.47000043107263));
#51769=CARTESIAN_POINT('Ctrl Pts',(9.82859575068344,-27.0087985025163,-21.5387980714436));
#51770=CARTESIAN_POINT('Ctrl Pts',(9.82859575068344,-20.3305326751374,-29.913078543345));
#51771=CARTESIAN_POINT('Ctrl Pts',(9.82859575068344,-10.0861224473418,-33.0403564279984));
#51772=CARTESIAN_POINT('Ctrl Pts',(8.97989469943246,-10.3313960385027,-33.8438294094779));
#51773=CARTESIAN_POINT('Ctrl Pts',(8.97989469943246,7.49247536092943,-39.2848648236118));
#51774=CARTESIAN_POINT('Ctrl Pts',(8.97989469943246,22.0625769943999,-27.6655964976071));
#51775=CARTESIAN_POINT('Ctrl Pts',(8.97989469943246,49.7281734920069,-5.6030195032072));
#51776=CARTESIAN_POINT('Ctrl Pts',(8.97989469943246,27.6655964976071,22.0625769943999));
#51777=CARTESIAN_POINT('Ctrl Pts',(8.97989469943246,5.6030195032072,49.7281734920069));
#51778=CARTESIAN_POINT('Ctrl Pts',(8.97989469943246,-22.0625769943999,27.6655964976071));
#51779=CARTESIAN_POINT('Ctrl Pts',(8.97989469943246,-49.7281734920069,5.6030195032072));
#51780=CARTESIAN_POINT('Ctrl Pts',(8.97989469943246,-27.6655964976071,-22.0625769943999));
#51781=CARTESIAN_POINT('Ctrl Pts',(8.97989469943246,-20.8249290881771,-30.6405026089669));
#51782=CARTESIAN_POINT('Ctrl Pts',(8.97989469943246,-10.3313960385027,-33.8438294094779));
#51783=CARTESIAN_POINT('Ctrl Pts',(8.1713316609345,-10.5843692822308,-34.6725250933902));
#51784=CARTESIAN_POINT('Ctrl Pts',(8.1713316609345,7.6759351555732,-40.2467890056693));
#51785=CARTESIAN_POINT('Ctrl Pts',(8.1713316609345,22.6027984365432,-28.3430127596098));
#51786=CARTESIAN_POINT('Ctrl Pts',(8.1713316609345,50.945811196153,-5.74021432306657));
#51787=CARTESIAN_POINT('Ctrl Pts',(8.1713316609345,28.3430127596098,22.6027984365432));
#51788=CARTESIAN_POINT('Ctrl Pts',(8.1713316609345,5.74021432306657,50.945811196153));
#51789=CARTESIAN_POINT('Ctrl Pts',(8.1713316609345,-22.6027984365432,28.3430127596098));
#51790=CARTESIAN_POINT('Ctrl Pts',(8.1713316609345,-50.945811196153,5.74021432306657));
#51791=CARTESIAN_POINT('Ctrl Pts',(8.1713316609345,-28.3430127596098,-22.6027984365432));
#51792=CARTESIAN_POINT('Ctrl Pts',(8.1713316609345,-21.3348456417785,-31.3907620420157));
#51793=CARTESIAN_POINT('Ctrl Pts',(8.1713316609345,-10.5843692822308,-34.6725250933902));
#51794=CARTESIAN_POINT('Ctrl Pts',(7.40358438374929,-10.8444940039127,-35.5246477564824));
#51795=CARTESIAN_POINT('Ctrl Pts',(7.40358438374929,7.86458130375168,-41.23590649671));
#51796=CARTESIAN_POINT('Ctrl Pts',(7.40358438374929,23.1582917773139,-29.039579376772));
#51797=CARTESIAN_POINT('Ctrl Pts',(7.40358438374929,52.1978711540859,-5.88128759945807));
#51798=CARTESIAN_POINT('Ctrl Pts',(7.40358438374929,29.039579376772,23.1582917773139));
#51799=CARTESIAN_POINT('Ctrl Pts',(7.40358438374929,5.88128759945807,52.1978711540859));
#51800=CARTESIAN_POINT('Ctrl Pts',(7.40358438374929,-23.1582917773139,29.039579376772));
#51801=CARTESIAN_POINT('Ctrl Pts',(7.40358438374929,-52.1978711540859,5.88128759945807));
#51802=CARTESIAN_POINT('Ctrl Pts',(7.40358438374929,-29.039579376772,-23.1582917773139));
#51803=CARTESIAN_POINT('Ctrl Pts',(7.40358438374929,-21.8591773838701,-32.1622310848871));
#51804=CARTESIAN_POINT('Ctrl Pts',(7.40358438374929,-10.8444940039127,-35.5246477564824));
#51805=CARTESIAN_POINT('Ctrl Pts',(6.82198164612729,-11.058045141737,-36.2242035814446));
#51806=CARTESIAN_POINT('Ctrl Pts',(6.82198164612729,8.01945162645387,-42.0479291460297));
#51807=CARTESIAN_POINT('Ctrl Pts',(6.82198164612729,23.6143277673129,-29.6114304207775));
#51808=CARTESIAN_POINT('Ctrl Pts',(6.82198164612729,53.2257581880904,-5.99710265346456));
#51809=CARTESIAN_POINT('Ctrl Pts',(6.82198164612729,29.6114304207775,23.6143277673129));
#51810=CARTESIAN_POINT('Ctrl Pts',(6.82198164612729,5.99710265346456,53.2257581880904));
#51811=CARTESIAN_POINT('Ctrl Pts',(6.82198164612729,-23.6143277673129,29.6114304207775));
#51812=CARTESIAN_POINT('Ctrl Pts',(6.82198164612729,-53.2257581880904,5.99710265346456));
#51813=CARTESIAN_POINT('Ctrl Pts',(6.82198164612729,-29.6114304207775,-23.6143277673129));
#51814=CARTESIAN_POINT('Ctrl Pts',(6.82198164612729,-22.2896310500849,-32.7955737784852));
#51815=CARTESIAN_POINT('Ctrl Pts',(6.82198164612729,-11.058045141737,-36.2242035814446));
#51816=CARTESIAN_POINT('Ctrl Pts',(6.40395249919757,-11.2211992099643,-36.7586675040324));
#51817=CARTESIAN_POINT('Ctrl Pts',(6.40395249919757,8.13777327743625,-42.6683182485135));
#51818=CARTESIAN_POINT('Ctrl Pts',(6.40395249919757,23.9627413968746,-30.048327293349));
#51819=CARTESIAN_POINT('Ctrl Pts',(6.40395249919757,54.0110686902236,-6.08558589647434));
#51820=CARTESIAN_POINT('Ctrl Pts',(6.40395249919757,30.048327293349,23.9627413968746));
#51821=CARTESIAN_POINT('Ctrl Pts',(6.40395249919757,6.08558589647434,54.0110686902236));
#51822=CARTESIAN_POINT('Ctrl Pts',(6.40395249919757,-23.9627413968746,30.048327293349));
#51823=CARTESIAN_POINT('Ctrl Pts',(6.40395249919757,-54.0110686902236,6.08558589647434));
#51824=CARTESIAN_POINT('Ctrl Pts',(6.40395249919757,-30.048327293349,-23.9627413968746));
#51825=CARTESIAN_POINT('Ctrl Pts',(6.40395249919757,-22.6184996646089,-33.2794505589853));
#51826=CARTESIAN_POINT('Ctrl Pts',(6.40395249919757,-11.2211992099643,-36.7586675040324));
#51827=CARTESIAN_POINT('Ctrl Pts',(6.13331019225912,-11.3312924070318,-37.1193133806217));
#51828=CARTESIAN_POINT('Ctrl Pts',(6.13331019225912,8.21761442991556,-43.086944767977));
#51829=CARTESIAN_POINT('Ctrl Pts',(6.13331019225912,24.1978441485076,-30.3431368191721));
#51830=CARTESIAN_POINT('Ctrl Pts',(6.13331019225912,54.5409809676797,-6.14529267066448));
#51831=CARTESIAN_POINT('Ctrl Pts',(6.13331019225912,30.3431368191721,24.1978441485076));
#51832=CARTESIAN_POINT('Ctrl Pts',(6.13331019225912,6.14529267066448,54.5409809676797));
#51833=CARTESIAN_POINT('Ctrl Pts',(6.13331019225912,-24.1978441485076,30.3431368191721));
#51834=CARTESIAN_POINT('Ctrl Pts',(6.13331019225912,-54.5409809676797,6.14529267066448));
#51835=CARTESIAN_POINT('Ctrl Pts',(6.13331019225912,-30.3431368191721,-24.1978441485076));
#51836=CARTESIAN_POINT('Ctrl Pts',(6.13331019225912,-22.8404138196251,-33.6059612144093));
#51837=CARTESIAN_POINT('Ctrl Pts',(6.13331019225912,-11.3312924070318,-37.1193133806217));
#51838=CARTESIAN_POINT('Ctrl Pts',(6.,-11.3866699594342,-37.3007204653599));
#51839=CARTESIAN_POINT('Ctrl Pts',(6.,8.25777501860823,-43.2975164711894));
#51840=CARTESIAN_POINT('Ctrl Pts',(6.,24.3161022724906,-30.4914278162532));
#51841=CARTESIAN_POINT('Ctrl Pts',(6.,54.8075300887437,-6.17532554376256));
#51842=CARTESIAN_POINT('Ctrl Pts',(6.,30.4914278162532,24.3161022724906));
#51843=CARTESIAN_POINT('Ctrl Pts',(6.,6.17532554376256,54.8075300887437));
#51844=CARTESIAN_POINT('Ctrl Pts',(6.,-24.3161022724906,30.4914278162532));
#51845=CARTESIAN_POINT('Ctrl Pts',(6.,-54.8075300887437,6.17532554376256));
#51846=CARTESIAN_POINT('Ctrl Pts',(6.,-30.4914278162532,-24.3161022724906));
#51847=CARTESIAN_POINT('Ctrl Pts',(6.,-22.9520379987349,-33.7701980738366));
#51848=CARTESIAN_POINT('Ctrl Pts',(6.,-11.3866699594342,-37.3007204653599));
#51849=CARTESIAN_POINT('Ctrl Pts',(24.5,-7.88307893260267,-25.8235757892348));
#51850=CARTESIAN_POINT('Ctrl Pts',(23.5178991898112,-5.12440787864319,-26.8408810021941));
#51851=CARTESIAN_POINT('Ctrl Pts',(22.3947886245986,-2.29122169990625,-27.4715439015176));
#51852=CARTESIAN_POINT('Ctrl Pts',(21.1743874927566,0.532981741024215,-27.7985414433729));
#51853=CARTESIAN_POINT('Ctrl Pts',(20.5031871793438,2.08624663502909,-27.9783846497186));
#51854=CARTESIAN_POINT('Ctrl Pts',(19.8411792966416,3.6507154806329,-28.0507750408847));
#51855=CARTESIAN_POINT('Ctrl Pts',(19.1295827650275,5.18988031863482,-28.0566862810056));
#51856=CARTESIAN_POINT('Ctrl Pts',(18.8261415870923,5.84621571479024,-28.0592069701682));
#51857=CARTESIAN_POINT('Ctrl Pts',(18.5104994276276,6.50331037286216,-28.0498981370496));
#51858=CARTESIAN_POINT('Ctrl Pts',(18.2016639423759,7.11415464453783,-28.0364358938641));
#51859=CARTESIAN_POINT('Ctrl Pts',(17.6747132403632,8.15640799025529,-28.013465934659));
#51860=CARTESIAN_POINT('Ctrl Pts',(17.2016343370993,9.08626906934427,-27.9569617268139));
#51861=CARTESIAN_POINT('Ctrl Pts',(16.872935292646,9.71033923360541,-27.916829044088));
#51862=CARTESIAN_POINT('Ctrl Pts',(16.6342454025477,10.1635174263466,-27.8876860764072));
#51863=CARTESIAN_POINT('Ctrl Pts',(16.5014949770664,10.4082918220469,-27.8702638626044));
#51864=CARTESIAN_POINT('Ctrl Pts',(16.3424569562979,10.698116742743,-27.8501213404638));
#51865=CARTESIAN_POINT('Ctrl Pts',(15.993118510103,11.334738017173,-27.8058768424938));
#51866=CARTESIAN_POINT('Ctrl Pts',(15.6312480487537,11.9648274577435,-27.7609569624451));
#51867=CARTESIAN_POINT('Ctrl Pts',(15.2503296894305,12.58375600882,-27.7280544894048));
#51868=CARTESIAN_POINT('Ctrl Pts',(14.7484414179076,13.3992404114303,-27.684703033853));
#51869=CARTESIAN_POINT('Ctrl Pts',(14.2669345517206,14.1852815321393,-27.6314704530746));
#51870=CARTESIAN_POINT('Ctrl Pts',(13.7912435751455,14.9172443259166,-27.6009121644364));
#51871=CARTESIAN_POINT('Ctrl Pts',(13.5533980868579,15.2832257228053,-27.5856330201174));
#51872=CARTESIAN_POINT('Ctrl Pts',(13.3161115657262,15.6377572992835,-27.5758360909478));
#51873=CARTESIAN_POINT('Ctrl Pts',(13.0766514227367,15.9813914150943,-27.5754070621212));
#51874=CARTESIAN_POINT('Ctrl Pts',(12.9188702359555,16.2078132234764,-27.5751243734174));
#51875=CARTESIAN_POINT('Ctrl Pts',(12.7601526360409,16.4295109353367,-27.5789102998031));
#51876=CARTESIAN_POINT('Ctrl Pts',(12.5997389313808,16.6466716884716,-27.5879931844747));
#51877=CARTESIAN_POINT('Ctrl Pts',(12.5166971934814,16.7590898037572,-27.5926951426389));
#51878=CARTESIAN_POINT('Ctrl Pts',(12.4397215765388,16.861779476413,-27.59820158806));
#51879=CARTESIAN_POINT('Ctrl Pts',(12.3478597934844,16.9819818549666,-27.606669709847));
#51880=CARTESIAN_POINT('Ctrl Pts',(11.9116121727781,17.5528177336491,-27.6468844526771));
#51881=CARTESIAN_POINT('Ctrl Pts',(10.7144663992386,19.17879676418,-27.7119011061896));
#51882=CARTESIAN_POINT('Ctrl Pts',(9.56604185022482,20.3673840450418,-28.2355768679772));
#51883=CARTESIAN_POINT('Ctrl Pts',(9.07284645450855,20.8778274823851,-28.4604714636071));
#51884=CARTESIAN_POINT('Ctrl Pts',(8.57333454992941,21.3352833188185,-28.7628944317207));
#51885=CARTESIAN_POINT('Ctrl Pts',(8.00348148263335,21.8507631464374,-29.1850206512921));
#51886=CARTESIAN_POINT('Ctrl Pts',(7.63919428966136,22.1802914234861,-29.4548712223124));
#51887=CARTESIAN_POINT('Ctrl Pts',(7.24388644384718,22.5359692004009,-29.7845767075602));
#51888=CARTESIAN_POINT('Ctrl Pts',(6.94254646282516,22.8138796544531,-30.0547884375835));
#51889=CARTESIAN_POINT('Ctrl Pts',(6.91433564865254,22.8398970456712,-30.0800850904774));
#51890=CARTESIAN_POINT('Ctrl Pts',(6.88669635040547,22.8654448722984,-30.1050387574276));
#51891=CARTESIAN_POINT('Ctrl Pts',(6.85962514029878,22.8905248103199,-30.129631969423));
#51892=CARTESIAN_POINT('Ctrl Pts',(6.4400006207374,23.279283085308,-30.5108456177005));
#51893=CARTESIAN_POINT('Ctrl Pts',(6.15412442492902,23.5258752447222,-30.8298076941652));
#51894=CARTESIAN_POINT('Ctrl Pts',(6.,23.6628748086085,-31.0011024931715));
#51895=CARTESIAN_POINT('Ctrl Pts',(2.09999999999998,5.34456416452658,-8.14535940885845));
#51896=CARTESIAN_POINT('Ctrl Pts',(2.73333333333332,5.34456416452658,-8.14535940885845));
#51897=CARTESIAN_POINT('Ctrl Pts',(3.36703045510619,5.34460712586018,-8.14533631625124));
#51898=CARTESIAN_POINT('Ctrl Pts',(4.1258438026898,5.34462008683109,-8.14532944421707));
#51899=CARTESIAN_POINT('Ctrl Pts',(4.38280550094044,5.34570783050074,-8.14463189797639));
#51900=CARTESIAN_POINT('Ctrl Pts',(4.88877630191765,5.35053371396832,-8.14154574907976));
#51901=CARTESIAN_POINT('Ctrl Pts',(5.76582860138385,5.36167176813889,-8.13444079857371));
#51902=CARTESIAN_POINT('Ctrl Pts',(6.49307225725675,5.36150896502748,-8.13458573839888));
#51903=CARTESIAN_POINT('Ctrl Pts',(7.02345937097035,5.34325603592381,-8.14610072176819));
#51904=CARTESIAN_POINT('Ctrl Pts',(7.14991970135013,5.33879812318534,-8.14899078713681));
#51905=CARTESIAN_POINT('Ctrl Pts',(7.33710498699582,5.33174922546116,-8.15365385893716));
#51906=CARTESIAN_POINT('Ctrl Pts',(7.52538047832545,5.32413774318376,-8.15876542857883));
#51907=CARTESIAN_POINT('Ctrl Pts',(7.90085937976029,5.30771267984777,-8.16986641378499));
#51908=CARTESIAN_POINT('Ctrl Pts',(8.46131778044036,5.27795323293097,-8.19002168993195));
#51909=CARTESIAN_POINT('Ctrl Pts',(9.06510517903235,5.23166569178312,-8.21981836831304));
#51910=CARTESIAN_POINT('Ctrl Pts',(9.52848763525404,5.18451311071437,-8.24862090594879));
#51911=CARTESIAN_POINT('Ctrl Pts',(9.75208483560215,5.15725817655892,-8.26472591834395));
#51912=CARTESIAN_POINT('Ctrl Pts',(10.3694305746462,5.07483970414387,-8.31257577375928));
#51913=CARTESIAN_POINT('Ctrl Pts',(11.3479755118771,4.89091383636494,-8.42464079424009));
#51914=CARTESIAN_POINT('Ctrl Pts',(12.2739432230502,4.64635231866122,-8.56256142325114));
#51915=CARTESIAN_POINT('Ctrl Pts',(13.0009186596788,4.44074096877511,-8.66574892117875));
#51916=CARTESIAN_POINT('Ctrl Pts',(13.5007657464189,4.28304830756585,-8.74312201390955));
#51917=CARTESIAN_POINT('Ctrl Pts',(14.4712209115036,3.92573756082701,-8.91215537488908));
#51918=CARTESIAN_POINT('Ctrl Pts',(15.1525957863043,3.62734188705641,-9.03883135866711));
#51919=CARTESIAN_POINT('Ctrl Pts',(15.7474668256706,3.35786214483351,-9.13646540471693));
#51920=CARTESIAN_POINT('Ctrl Pts',(16.0037627434752,3.23694584628154,-9.17854126131123));
#51921=CARTESIAN_POINT('Ctrl Pts',(16.5107347057776,2.98182782255615,-9.26366275020945));
#51922=CARTESIAN_POINT('Ctrl Pts',(17.3591246875254,2.51561318345669,-9.40643332398099));
#51923=CARTESIAN_POINT('Ctrl Pts',(18.0498326782835,2.08512110773588,-9.51119006271148));
#51924=CARTESIAN_POINT('Ctrl Pts',(18.7837576316761,1.61772190021554,-9.59472621339316));
#51925=CARTESIAN_POINT('Ctrl Pts',(19.2874983687974,1.27668484968537,-9.6462243441966));
#51926=CARTESIAN_POINT('Ctrl Pts',(20.2705670405104,0.551057000957825,-9.72220562049248));
#51927=CARTESIAN_POINT('Ctrl Pts',(20.968423963075,-0.0130109990231726,
-9.73577142111487));
#51928=CARTESIAN_POINT('Ctrl Pts',(22.6569785206169,-1.37366893882804,-9.67192624996041));
#51929=CARTESIAN_POINT('Ctrl Pts',(23.7241254823866,-2.3362350951335,-9.47253804281166));
#51930=CARTESIAN_POINT('Ctrl Pts',(24.6950729185821,-3.32180370011223,-9.13150534684048));
#51931=CARTESIAN_POINT('Ctrl Pts',(2.09999999999998,7.95334816354381,-11.4166710731552));
#51932=CARTESIAN_POINT('Ctrl Pts',(2.73333333333332,7.95334816354381,-11.4166710731552));
#51933=CARTESIAN_POINT('Ctrl Pts',(3.36722921888214,7.95339083450222,-11.4166436748178));
#51934=CARTESIAN_POINT('Ctrl Pts',(4.12626245611356,7.95340335909069,-11.4166357236622));
#51935=CARTESIAN_POINT('Ctrl Pts',(4.38607734488415,7.95493785056024,-11.4155904452611));
#51936=CARTESIAN_POINT('Ctrl Pts',(4.89393849803322,7.96172076053339,-11.4109823514058));
#51937=CARTESIAN_POINT('Ctrl Pts',(5.77028399864619,7.97732575169866,-11.4004072666733));
#51938=CARTESIAN_POINT('Ctrl Pts',(6.48775133512661,7.97697012330154,-11.4006984916951));
#51939=CARTESIAN_POINT('Ctrl Pts',(7.00649985389096,7.95176660573384,-11.4175960094363));
#51940=CARTESIAN_POINT('Ctrl Pts',(7.1328122089054,7.94552344412315,-11.4218945357638));
#51941=CARTESIAN_POINT('Ctrl Pts',(7.31839339846734,7.93570247397948,-11.4287944424324));
#51942=CARTESIAN_POINT('Ctrl Pts',(7.50532535803233,7.92508991461552,-11.4363618062793));
#51943=CARTESIAN_POINT('Ctrl Pts',(7.87743482519494,7.90221930046077,-11.4527758654708));
#51944=CARTESIAN_POINT('Ctrl Pts',(8.43163383044899,7.86082555090579,-11.4825467102839));
#51945=CARTESIAN_POINT('Ctrl Pts',(9.02557103671809,7.79663844533022,-11.5264740745866));
#51946=CARTESIAN_POINT('Ctrl Pts',(9.47909108553348,7.73146286135872,-11.5688495286329));
#51947=CARTESIAN_POINT('Ctrl Pts',(9.69701368850754,7.69388237767458,-11.5925048579334));
#51948=CARTESIAN_POINT('Ctrl Pts',(10.2970955435366,7.58039638756159,-11.662716724276));
#51949=CARTESIAN_POINT('Ctrl Pts',(11.2524630852568,7.32685330737253,-11.8275326519127));
#51950=CARTESIAN_POINT('Ctrl Pts',(12.1686924220656,6.98608110701113,-12.0331549997054));
#51951=CARTESIAN_POINT('Ctrl Pts',(12.8916733902102,6.69791329894401,-12.1883803970336));
#51952=CARTESIAN_POINT('Ctrl Pts',(13.3792423851727,6.48008047549737,-12.3034763709601));
#51953=CARTESIAN_POINT('Ctrl Pts',(14.3391274674842,5.98209567733816,-12.5578967665008));
#51954=CARTESIAN_POINT('Ctrl Pts',(15.0158575632568,5.56322362445193,-12.7509990333251));
#51955=CARTESIAN_POINT('Ctrl Pts',(15.6096998984311,5.18299682455851,-12.9017952037445));
#51956=CARTESIAN_POINT('Ctrl Pts',(15.8629234378176,5.01414769058628,-12.9665415390874));
#51957=CARTESIAN_POINT('Ctrl Pts',(16.366769191659,4.65589390592607,-13.0986310142571));
#51958=CARTESIAN_POINT('Ctrl Pts',(17.2116336585144,3.99947370123076,-13.3224762399715));
#51959=CARTESIAN_POINT('Ctrl Pts',(17.9015681458004,3.38939186549384,-13.491162196428));
#51960=CARTESIAN_POINT('Ctrl Pts',(18.6346321455063,2.72577662783367,-13.630803315184));
#51961=CARTESIAN_POINT('Ctrl Pts',(19.1381734987811,2.24198588579176,-13.7198489991737));
#51962=CARTESIAN_POINT('Ctrl Pts',(20.1235843849346,1.20814441723857,-13.8612245457287));
#51963=CARTESIAN_POINT('Ctrl Pts',(20.8218560196981,0.402341697820859,-13.9055220555452));
#51964=CARTESIAN_POINT('Ctrl Pts',(22.509656326961,-1.54359381676115,-13.873432467644));
#51965=CARTESIAN_POINT('Ctrl Pts',(23.5814142719248,-2.93009156681438,-13.6326211887675));
#51966=CARTESIAN_POINT('Ctrl Pts',(24.5630597774301,-4.36475478204552,-13.1847221831164));
#51967=CARTESIAN_POINT('Ctrl Pts',(2.09999999999999,14.0405108279174,-19.0497316231808));
#51968=CARTESIAN_POINT('Ctrl Pts',(2.73333333333332,14.0405108279174,-19.0497316231808));
#51969=CARTESIAN_POINT('Ctrl Pts',(3.36770544049384,14.0406593647044,-19.0496470247757));
#51970=CARTESIAN_POINT('Ctrl Pts',(4.12725475148089,14.0407035545206,-19.0496222505543));
#51971=CARTESIAN_POINT('Ctrl Pts',(4.39373035273626,14.0433198866416,-19.0477371998816));
#51972=CARTESIAN_POINT('Ctrl Pts',(4.90599112616755,14.0547497465385,-19.0395208824725));
#51973=CARTESIAN_POINT('Ctrl Pts',(5.78072777450692,14.0807920378816,-19.0208473878005));
#51974=CARTESIAN_POINT('Ctrl Pts',(6.47530496203834,14.0798518061703,-19.0216406137609));
#51975=CARTESIAN_POINT('Ctrl Pts',(6.96716149433085,14.0396024305645,-19.0501859265548));
#51976=CARTESIAN_POINT('Ctrl Pts',(7.09313355494184,14.029212756938,-19.0577571393445));
#51977=CARTESIAN_POINT('Ctrl Pts',(7.27501518208594,14.0130979804571,-19.0697412543813));
#51978=CARTESIAN_POINT('Ctrl Pts',(7.4588585143809,13.9956499602412,-19.0829112118382));
#51979=CARTESIAN_POINT('Ctrl Pts',(7.8232328589516,13.9581658333788,-19.111391624162));
#51980=CARTESIAN_POINT('Ctrl Pts',(8.36318149154488,13.8906875946527,-19.1628145686548));
#51981=CARTESIAN_POINT('Ctrl Pts',(8.93517301674487,13.7869110179481,-19.2380842355627));
#51982=CARTESIAN_POINT('Ctrl Pts',(9.36766944102217,13.6824940828447,-19.3100449969906));
#51983=CARTESIAN_POINT('Ctrl Pts',(9.57402188182549,13.6227011914904,-19.3499427790005));
#51984=CARTESIAN_POINT('Ctrl Pts',(10.1401453128135,13.4431272840522,-19.4677531472923));
#51985=CARTESIAN_POINT('Ctrl Pts',(11.0615860966997,13.0381462718132,-19.7484552766342));
#51986=CARTESIAN_POINT('Ctrl Pts',(11.9725168252953,12.4760551457986,-20.1114798309039));
#51987=CARTESIAN_POINT('Ctrl Pts',(12.6928298617397,11.9972242157899,-20.3879965049244));
#51988=CARTESIAN_POINT('Ctrl Pts',(13.1763132367642,11.6403697206645,-20.591319917764));
#51989=CARTESIAN_POINT('Ctrl Pts',(14.1425443268685,10.807707670116,-21.0504208046439));
#51990=CARTESIAN_POINT('Ctrl Pts',(14.8246630432476,10.1039973091049,-21.4016095272698));
#51991=CARTESIAN_POINT('Ctrl Pts',(15.4199295464537,9.46515875405639,-21.6773329562573));
#51992=CARTESIAN_POINT('Ctrl Pts',(15.6784405514184,9.17859896251508,-21.7979768782073));
#51993=CARTESIAN_POINT('Ctrl Pts',(16.1907883125052,8.57011255948466,-22.0441196100552));
#51994=CARTESIAN_POINT('Ctrl Pts',(17.0509810894248,7.45168253371926,-22.4641884940993));
#51995=CARTESIAN_POINT('Ctrl Pts',(17.7490528301793,6.41387004578994,-22.7837202098578));
#51996=CARTESIAN_POINT('Ctrl Pts',(18.4852578323668,5.28986633116544,-23.053856315933));
#51997=CARTESIAN_POINT('Ctrl Pts',(19.0038260606132,4.45316762536295,-23.2340669203721));
#51998=CARTESIAN_POINT('Ctrl Pts',(20.0035139458143,2.67878447452734,-23.52668999913));
#51999=CARTESIAN_POINT('Ctrl Pts',(20.7091427978092,1.29885794752446,-23.6391186363694));
#52000=CARTESIAN_POINT('Ctrl Pts',(22.403146683307,-2.02022054163564,-23.6710719995345));
#52001=CARTESIAN_POINT('Ctrl Pts',(23.5046677369882,-4.44224583503547,-23.3201179538783));
#52002=CARTESIAN_POINT('Ctrl Pts',(24.5020292171972,-6.94171785952187,-22.6001034215803));
#52003=CARTESIAN_POINT('Ctrl Pts',(2.09999999999998,20.1276734922909,-26.6827921732065));
#52004=CARTESIAN_POINT('Ctrl Pts',(2.73333333333332,20.1276734922909,-26.6827921732065));
#52005=CARTESIAN_POINT('Ctrl Pts',(3.36824035468517,20.1277999966281,-26.6827248844676));
#52006=CARTESIAN_POINT('Ctrl Pts',(4.12831946050022,20.1278353407483,-26.682706983803));
#52007=CARTESIAN_POINT('Ctrl Pts',(4.40147222634207,20.1315942338715,-26.6799317263204));
#52008=CARTESIAN_POINT('Ctrl Pts',(4.9180724847728,20.1477887080798,-26.6680072176987));
#52009=CARTESIAN_POINT('Ctrl Pts',(5.79140913132176,20.1841869107284,-26.6412944630435));
#52010=CARTESIAN_POINT('Ctrl Pts',(6.46267874194441,20.1818673038256,-26.6431805808982));
#52011=CARTESIAN_POINT('Ctrl Pts',(6.92901748474213,20.1289400767798,-26.6814764936299));
#52012=CARTESIAN_POINT('Ctrl Pts',(7.05467459429316,20.1144377758426,-26.692294551178));
#52013=CARTESIAN_POINT('Ctrl Pts',(7.23308118280245,20.0923833573486,-26.7090822928829));
#52014=CARTESIAN_POINT('Ctrl Pts',(7.41407148153067,20.0684217407377,-26.7276006746662));
#52015=CARTESIAN_POINT('Ctrl Pts',(7.77136342402986,20.0171916206279,-26.767467725355));
#52016=CARTESIAN_POINT('Ctrl Pts',(8.29881147671608,19.9253506286527,-26.8391763377014));
#52017=CARTESIAN_POINT('Ctrl Pts',(8.85382441430446,19.7854312459419,-26.9431420824863));
#52018=CARTESIAN_POINT('Ctrl Pts',(9.27345552895879,19.6450682120238,-27.0422453297518));
#52019=CARTESIAN_POINT('Ctrl Pts',(9.47428870911876,19.5645742402598,-27.0973020227195));
#52020=CARTESIAN_POINT('Ctrl Pts',(10.0274094887188,19.3220973290901,-27.2604732414786));
#52021=CARTESIAN_POINT('Ctrl Pts',(10.957336519856,18.7566911999351,-27.6644010649527));
#52022=CARTESIAN_POINT('Ctrl Pts',(11.8782898182081,17.9599375300719,-28.1936376395817));
#52023=CARTESIAN_POINT('Ctrl Pts',(12.6022503935223,17.2852478950138,-28.5944892337399));
#52024=CARTESIAN_POINT('Ctrl Pts',(13.0991012510153,16.7709190727932,-28.8970744032444));
#52025=CARTESIAN_POINT('Ctrl Pts',(14.0799616178224,15.5798854129963,-29.5722844768448));
#52026=CARTESIAN_POINT('Ctrl Pts',(14.7680852092718,14.579052621997,-30.0849315139416));
#52027=CARTESIAN_POINT('Ctrl Pts',(15.3645561107598,13.6781623100496,-30.4847911076143));
#52028=CARTESIAN_POINT('Ctrl Pts',(15.6279528535259,13.2647887968605,-30.6643324056741));
#52029=CARTESIAN_POINT('Ctrl Pts',(16.1459139527021,12.3946624979674,-31.0266453695517));
#52030=CARTESIAN_POINT('Ctrl Pts',(17.013910567048,10.7975178255105,-31.6438588656908));
#52031=CARTESIAN_POINT('Ctrl Pts',(17.7140149010249,9.32634196499537,-32.1100100091169));
#52032=CARTESIAN_POINT('Ctrl Pts',(18.4510929547942,7.73876056396156,-32.505613445104));
#52033=CARTESIAN_POINT('Ctrl Pts',(18.9739954119137,6.5405150412443,-32.774374473624));
#52034=CARTESIAN_POINT('Ctrl Pts',(19.9765231119574,4.02047707679407,-33.2090980004561));
#52035=CARTESIAN_POINT('Ctrl Pts',(20.6834924480325,2.06477337861421,-33.3821520755448));
#52036=CARTESIAN_POINT('Ctrl Pts',(22.3784539898323,-2.62828368271897,-33.4598843240797));
#52037=CARTESIAN_POINT('Ctrl Pts',(23.4839952293235,-6.08084055797285,-32.9845938002433));
#52038=CARTESIAN_POINT('Ctrl Pts',(24.4831092917558,-9.6347294289213,-31.9813971448826));
#52039=CARTESIAN_POINT('Ctrl Pts',(2.09999999999998,23.6060521576472,-31.0445410589354));
#52040=CARTESIAN_POINT('Ctrl Pts',(2.73333333333332,23.6060521576472,-31.0445410589354));
#52041=CARTESIAN_POINT('Ctrl Pts',(3.36856654542017,23.6061635860875,-31.0444839306223));
#52042=CARTESIAN_POINT('Ctrl Pts',(4.12895234149475,23.606193256038,-31.0444699032081));
#52043=CARTESIAN_POINT('Ctrl Pts',(4.40592848799383,23.6106268023555,-31.041168515519));
#52044=CARTESIAN_POINT('Ctrl Pts',(4.92497320633879,23.6295933396541,-31.0270850709477));
#52045=CARTESIAN_POINT('Ctrl Pts',(5.79761961985324,23.6718783150368,-30.9958030248401));
#52046=CARTESIAN_POINT('Ctrl Pts',(6.45533229527709,23.6686137447905,-30.998435202078));
#52047=CARTESIAN_POINT('Ctrl Pts',(6.90782015375558,23.6091196795821,-31.0417634176017));
#52048=CARTESIAN_POINT('Ctrl Pts',(7.03331040148622,23.5922768022307,-31.0544297184954));
#52049=CARTESIAN_POINT('Ctrl Pts',(7.20984968522255,23.5669255464429,-31.0738857861351));
#52050=CARTESIAN_POINT('Ctrl Pts',(7.3893310776903,23.5393269357799,-31.095393818285));
#52051=CARTESIAN_POINT('Ctrl Pts',(7.74291210335288,23.4804567813196,-31.1415999795215));
#52052=CARTESIAN_POINT('Ctrl Pts',(8.26407103775564,23.375101565528,-31.2245832648744));
#52053=CARTESIAN_POINT('Ctrl Pts',(8.8115830223524,23.2149449411146,-31.3446386044841));
#52054=CARTESIAN_POINT('Ctrl Pts',(9.22667581471618,23.0537694784089,-31.4594769231126));
#52055=CARTESIAN_POINT('Ctrl Pts',(9.42604477578941,22.9609496680068,-31.5235804262132));
#52056=CARTESIAN_POINT('Ctrl Pts',(9.97678856421979,22.6803689675826,-31.7143127377213));
#52057=CARTESIAN_POINT('Ctrl Pts',(10.9141162969295,22.0169016367236,-32.1932131535475));
#52058=CARTESIAN_POINT('Ctrl Pts',(11.8388701416734,21.084176748631,-32.8181792996892));
#52059=CARTESIAN_POINT('Ctrl Pts',(12.5646367114059,20.2966269440717,-33.2903357867815));
#52060=CARTESIAN_POINT('Ctrl Pts',(13.0665475226764,19.6905411085284,-33.6504100246034));
#52061=CARTESIAN_POINT('Ctrl Pts',(14.0522782066389,18.294866663048,-34.4482865325554));
#52062=CARTESIAN_POINT('Ctrl Pts',(14.7430221797613,17.1241308380047,-35.0527157552754));
#52063=CARTESIAN_POINT('Ctrl Pts',(15.3400953918683,16.0732499778056,-35.5231797794399));
#52064=CARTESIAN_POINT('Ctrl Pts',(15.6052823188849,15.5879425580852,-35.7359287758697));
#52065=CARTESIAN_POINT('Ctrl Pts',(16.1254560189452,14.569125220435,-36.1638827804151));
#52066=CARTESIAN_POINT('Ctrl Pts',(16.996829231524,12.699834206496,-36.8925871221106));
#52067=CARTESIAN_POINT('Ctrl Pts',(17.6980324177114,10.9811103327506,-37.4420145883602));
#52068=CARTESIAN_POINT('Ctrl Pts',(18.4354718827656,9.1283982665082,-37.9088830089142));
#52069=CARTESIAN_POINT('Ctrl Pts',(18.9606999869237,7.72463416692537,-38.2276352431276));
#52070=CARTESIAN_POINT('Ctrl Pts',(19.9652054243195,4.77933627887349,-38.7429228174106));
#52071=CARTESIAN_POINT('Ctrl Pts',(20.6728661623116,2.49477830019891,-38.9501574688157));
#52072=CARTESIAN_POINT('Ctrl Pts',(22.3680046594236,-2.98344825060076,-39.0530209806881));
#52073=CARTESIAN_POINT('Ctrl Pts',(23.4757593035169,-7.02359945440365,-38.5057313141264));
#52074=CARTESIAN_POINT('Ctrl Pts',(24.4767076204831,-11.1800381806575,-37.3402432932818));
#52075=CARTESIAN_POINT('',(3.2,22.7328514723457,-29.9495820327474));
#52076=CARTESIAN_POINT('Ctrl Pts',(3.2,22.7328514723457,-29.9495820327475));
#52077=CARTESIAN_POINT('Ctrl Pts',(3.45174020120132,22.248104974443,-29.3417291505565));
#52078=CARTESIAN_POINT('Ctrl Pts',(3.71840125348693,21.7576384332226,-28.7267035609156));
#52079=CARTESIAN_POINT('Ctrl Pts',(4.,21.2644490398942,-28.1082636227258));
#52080=CARTESIAN_POINT('Ctrl Pts',(4.62816482155513,20.1642870857335,-26.7287041672028));
#52081=CARTESIAN_POINT('Ctrl Pts',(5.32582969298372,19.112709122184,-25.3133815304913));
#52082=CARTESIAN_POINT('Ctrl Pts',(6.03866111506183,18.0956114522777,-24.0462604082467));
#52083=CARTESIAN_POINT('Ctrl Pts',(6.32798220275237,17.6827960305236,-23.5319664953119));
#52084=CARTESIAN_POINT('Ctrl Pts',(6.61604117795301,17.2794652714956,-23.0487162961897));
#52085=CARTESIAN_POINT('Ctrl Pts',(6.89476148100327,16.8874284567183,-22.6097510295672));
#52086=CARTESIAN_POINT('Ctrl Pts',(7.65522892342214,15.817785410966,-21.4120672226614));
#52087=CARTESIAN_POINT('Ctrl Pts',(8.35226708635794,14.9194503847516,-20.4715588563443));
#52088=CARTESIAN_POINT('Ctrl Pts',(8.78926323490749,14.355233051296,-19.9177206283292));
#52089=CARTESIAN_POINT('Ctrl Pts',(8.99031958628575,14.0956438562298,-19.662906727227));
#52090=CARTESIAN_POINT('Ctrl Pts',(9.18275523109629,13.8483915014505,-19.4286423508446));
#52091=CARTESIAN_POINT('Ctrl Pts',(9.37496047537633,13.6006174248028,-19.2038629336386));
#52092=CARTESIAN_POINT('Ctrl Pts',(9.48075234282032,13.4642398646018,-19.0801418853484));
#52093=CARTESIAN_POINT('Ctrl Pts',(9.58626091404298,13.327984642801,-18.9596114725911));
#52094=CARTESIAN_POINT('Ctrl Pts',(9.69257910363365,13.1899893895466,-18.8412172354227));
#52095=CARTESIAN_POINT('Ctrl Pts',(10.0319880484304,12.7494549572509,-18.4632568575979));
#52096=CARTESIAN_POINT('Ctrl Pts',(10.3788056761856,12.2902497006998,-18.1076143195385));
#52097=CARTESIAN_POINT('Ctrl Pts',(10.7756849101744,11.7648559982034,-17.731189557802));
#52098=CARTESIAN_POINT('Ctrl Pts',(10.8890930420524,11.6147248923208,-17.6236262857404));
#52099=CARTESIAN_POINT('Ctrl Pts',(11.0576203537643,11.3913842275629,-17.466093373954));
#52100=CARTESIAN_POINT('Ctrl Pts',(11.2725125506914,11.1084603654433,-17.2736114037459));
#52101=CARTESIAN_POINT('Ctrl Pts',(11.5968279603642,10.6814715330817,-16.9831175192989));
#52102=CARTESIAN_POINT('Ctrl Pts',(12.025567884929,10.1177168965354,-16.6161644397795));
#52103=CARTESIAN_POINT('Ctrl Pts',(12.532035905153,9.4869884079099,-16.2042316548138));
#52104=CARTESIAN_POINT('Ctrl Pts',(13.0988763173527,8.7810753350164,-15.7431953399735));
#52105=CARTESIAN_POINT('Ctrl Pts',(13.7495416906409,7.95432619929805,-15.2695479464202));
#52106=CARTESIAN_POINT('Ctrl Pts',(14.4398764931151,7.10916666494483,-14.8029953911254));
#52107=CARTESIAN_POINT('Ctrl Pts',(14.7901814026826,6.68029717554548,-14.5662470045378));
#52108=CARTESIAN_POINT('Ctrl Pts',(15.1459546144383,6.25591299863767,-14.3334813778935));
#52109=CARTESIAN_POINT('Ctrl Pts',(15.4570717747561,5.9001432106612,-14.1321338018072));
#52110=CARTESIAN_POINT('Ctrl Pts',(15.7998231427917,5.50819896235894,-13.9103133240047));
#52111=CARTESIAN_POINT('Ctrl Pts',(16.0676294537022,5.20198370959687,-13.7458456728629));
#52112=CARTESIAN_POINT('Ctrl Pts',(16.3615308038184,4.86844862366034,-13.5698041325856));
#52113=CARTESIAN_POINT('Ctrl Pts',(17.0296616067428,4.110217793206,-13.1696059858025));
#52114=CARTESIAN_POINT('Ctrl Pts',(17.7084691897444,3.34909561452446,-12.7911871969579));
#52115=CARTESIAN_POINT('Ctrl Pts',(18.4207032016838,2.62478996807377,-12.4048105193286));
#52116=CARTESIAN_POINT('Ctrl Pts',(18.8298642044523,2.20869410681929,-12.1828465774007));
#52117=CARTESIAN_POINT('Ctrl Pts',(19.2113759275114,1.81977531174774,-11.9848915561808));
#52118=CARTESIAN_POINT('Ctrl Pts',(19.5701113610614,1.45769348413641,-11.8009398056712));
#52119=CARTESIAN_POINT('Ctrl Pts',(20.1215476022647,0.901113276683472,-11.5181752600562));
#52120=CARTESIAN_POINT('Ctrl Pts',(20.6514912601111,0.363614694912416,-11.2519266478905));
#52121=CARTESIAN_POINT('Ctrl Pts',(21.3979544325339,-0.320646129817996,
-10.8732172390043));
#52122=CARTESIAN_POINT('Ctrl Pts',(21.8107631281271,-0.699055713757323,
-10.6637835484127));
#52123=CARTESIAN_POINT('Ctrl Pts',(22.3076315954084,-1.14579605062356,-10.4120946972692));
#52124=CARTESIAN_POINT('Ctrl Pts',(22.8472772293558,-1.62955662628835,-10.1269169192224));
#52125=CARTESIAN_POINT('Ctrl Pts',(23.3953136567549,-2.12083905484158,-9.83730499461342));
#52126=CARTESIAN_POINT('Ctrl Pts',(23.9608264582608,-2.62824069788209,-9.52568075404202));
#52127=CARTESIAN_POINT('Ctrl Pts',(24.5,-3.12544889498789,-9.19761041611355));
#52128=CARTESIAN_POINT('Ctrl Pts',(2.79761440945937,23.3193979595446,-30.6850251548975));
#52129=CARTESIAN_POINT('Ctrl Pts',(2.93206893024197,23.1240804350591,-30.4400833497039));
#52130=CARTESIAN_POINT('Ctrl Pts',(3.06672946893634,22.928527622209,-30.1948428266097));
#52131=CARTESIAN_POINT('Ctrl Pts',(3.20144293004172,22.7329275986254,-29.9495427664931));
#52132=CARTESIAN_POINT('Origin',(2.9,0.,0.));
#52133=CARTESIAN_POINT('Origin',(3.2,0.,0.));
#52134=CARTESIAN_POINT('Ctrl Pts',(2.1,-1.28155061440791,-9.65940339474764));
#52135=CARTESIAN_POINT('Ctrl Pts',(2.73333333333333,-1.28155061440791,-9.65940339474764));
#52136=CARTESIAN_POINT('Ctrl Pts',(3.36631731606888,-1.28160190790707,-9.65938099478861));
#52137=CARTESIAN_POINT('Ctrl Pts',(4.12417509565397,-1.28161736833688,-9.65937414787961));
#52138=CARTESIAN_POINT('Ctrl Pts',(4.36792464736457,-1.2804091068822,-9.6595464518039));
#52139=CARTESIAN_POINT('Ctrl Pts',(4.86515686825693,-1.27488660478215,-9.66034332028297));
#52140=CARTESIAN_POINT('Ctrl Pts',(5.74557748576906,-1.26184798249892,-9.66223911748733));
#52141=CARTESIAN_POINT('Ctrl Pts',(6.51835851955694,-1.26164230505555,-9.66227145200332));
#52142=CARTESIAN_POINT('Ctrl Pts',(7.10309338724208,-1.28515972010509,-9.658747726709));
#52143=CARTESIAN_POINT('Ctrl Pts',(7.23024869643521,-1.29045297976683,-9.65801464099689));
#52144=CARTESIAN_POINT('Ctrl Pts',(7.42492914335972,-1.29917956503778,-9.6568856789673));
#52145=CARTESIAN_POINT('Ctrl Pts',(7.61949923308775,-1.30862177632596,-9.65572731198123));
#52146=CARTESIAN_POINT('Ctrl Pts',(8.01074641232386,-1.32920013902525,-9.65326080679973));
#52147=CARTESIAN_POINT('Ctrl Pts',(8.60081577956197,-1.36699309999216,-9.64872946052249));
#52148=CARTESIAN_POINT('Ctrl Pts',(9.25152613287282,-1.42571070422604,-9.64034868889098));
#52149=CARTESIAN_POINT('Ctrl Pts',(9.76265059143103,-1.48569089122728,-9.63040536367191));
#52150=CARTESIAN_POINT('Ctrl Pts',(10.0141493386521,-1.52058012336349,-9.62412541731759));
#52151=CARTESIAN_POINT('Ctrl Pts',(10.7177310059152,-1.62700473913724,-9.60414949273162));
#52152=CARTESIAN_POINT('Ctrl Pts',(11.8208420069978,-1.8678059348864,-9.56287894547604));
#52153=CARTESIAN_POINT('Ctrl Pts',(12.8080068087818,-2.16229044149045,-9.50065093843371));
#52154=CARTESIAN_POINT('Ctrl Pts',(13.560404949554,-2.3920805659028,-9.44058642082993));
#52155=CARTESIAN_POINT('Ctrl Pts',(14.1415309352711,-2.58837046806001,-9.38738192823919));
#52156=CARTESIAN_POINT('Ctrl Pts',(15.2007195797304,-3.00388456952685,-9.26580533995201));
#52157=CARTESIAN_POINT('Ctrl Pts',(15.9284992208669,-3.33152214815673,-9.15357602363817));
#52158=CARTESIAN_POINT('Ctrl Pts',(16.6747671783401,-3.66443059394905,-9.01938328351392));
#52159=CARTESIAN_POINT('Ctrl Pts',(17.2497798582943,-3.93726930925875,-8.90311266260874));
#52160=CARTESIAN_POINT('Ctrl Pts',(18.2984578568314,-4.48329425942222,-8.64639146157842));
#52161=CARTESIAN_POINT('Ctrl Pts',(19.0236730578911,-4.89100422008468,-8.42123413259578));
#52162=CARTESIAN_POINT('Ctrl Pts',(19.7682055319328,-5.29723443513983,-8.16373299921013));
#52163=CARTESIAN_POINT('Ctrl Pts',(20.3331603255054,-5.61711561770474,-7.94814232298995));
#52164=CARTESIAN_POINT('Ctrl Pts',(21.3723035139214,-6.23437055880962,-7.48347305814291));
#52165=CARTESIAN_POINT('Ctrl Pts',(22.0962492277569,-6.67058221462383,-7.09344903901532));
#52166=CARTESIAN_POINT('Ctrl Pts',(23.230243247065,-7.3072573440811,-6.43796882578206));
#52167=CARTESIAN_POINT('Ctrl Pts',(23.8854423668127,-7.66333672971863,-6.00193696589197));
#52168=CARTESIAN_POINT('Ctrl Pts',(24.5000000001022,-7.98533675016187,-5.53162409663373));
#52169=CARTESIAN_POINT('Ctrl Pts',(2.1,-2.21255777005862,-13.7384122607767));
#52170=CARTESIAN_POINT('Ctrl Pts',(2.73333333333334,-2.21255777005862,-13.7384122607767));
#52171=CARTESIAN_POINT('Ctrl Pts',(3.36612146729749,-2.21261791852302,-13.7383900087247));
#52172=CARTESIAN_POINT('Ctrl Pts',(4.12376029167732,-2.21263571619322,-13.738383314838));
#52173=CARTESIAN_POINT('Ctrl Pts',(4.36465706155994,-2.21092930027329,-13.7386765514597));
#52174=CARTESIAN_POINT('Ctrl Pts',(4.85999961632898,-2.20309745300305,-13.740033035105));
#52175=CARTESIAN_POINT('Ctrl Pts',(5.74112770525578,-2.18454375550621,-13.7432623997142));
#52176=CARTESIAN_POINT('Ctrl Pts',(6.52368850139862,-2.18411163742531,-13.7433502946453));
#52177=CARTESIAN_POINT('Ctrl Pts',(7.12006273833317,-2.21802212159882,-13.7373260594817));
#52178=CARTESIAN_POINT('Ctrl Pts',(7.24736606576941,-2.22555725019054,-13.7360683688785));
#52179=CARTESIAN_POINT('Ctrl Pts',(7.44365067907975,-2.23803816094386,-13.7341021683655));
#52180=CARTESIAN_POINT('Ctrl Pts',(7.63956445145365,-2.25153194017601,-13.7320672730228));
#52181=CARTESIAN_POINT('Ctrl Pts',(8.03418103434733,-2.28097257160256,-13.7277103278323));
#52182=CARTESIAN_POINT('Ctrl Pts',(8.63051246970729,-2.33509483691623,-13.7197091635916));
#52183=CARTESIAN_POINT('Ctrl Pts',(9.29107501673555,-2.41942454694128,-13.7053013523184));
#52184=CARTESIAN_POINT('Ctrl Pts',(9.81206255454758,-2.50581650276758,-13.6885430133877));
#52185=CARTESIAN_POINT('Ctrl Pts',(10.0692361367767,-2.55617164041776,-13.6780601778355));
#52186=CARTESIAN_POINT('Ctrl Pts',(10.7900877092649,-2.7099459022409,-13.6448883888619));
#52187=CARTESIAN_POINT('Ctrl Pts',(11.9163843329042,-3.05720701099178,-13.5754688821817));
#52188=CARTESIAN_POINT('Ctrl Pts',(12.9133076943621,-3.47807008854133,-13.4740241097693));
#52189=CARTESIAN_POINT('Ctrl Pts',(13.6697202365407,-3.80490979930021,-13.378562011322));
#52190=CARTESIAN_POINT('Ctrl Pts',(14.2631414165878,-4.08738507427771,-13.2935308185664));
#52191=CARTESIAN_POINT('Ctrl Pts',(15.3329106576864,-4.68070912639053,-13.101240706448));
#52192=CARTESIAN_POINT('Ctrl Pts',(16.0654025907068,-5.14567124856755,-12.9267704504935));
#52193=CARTESIAN_POINT('Ctrl Pts',(16.8131118314614,-5.61574596327599,-12.7209271490644));
#52194=CARTESIAN_POINT('Ctrl Pts',(17.3939372393177,-6.00393438452058,-12.5422941481349));
#52195=CARTESIAN_POINT('Ctrl Pts',(18.4451742590423,-6.77513244775298,-12.1515155544068));
#52196=CARTESIAN_POINT('Ctrl Pts',(19.1720636185852,-7.34823939444788,-11.812629885177));
#52197=CARTESIAN_POINT('Ctrl Pts',(19.9174234244712,-7.91731656489557,-11.4273658819217));
#52198=CARTESIAN_POINT('Ctrl Pts',(20.4826637954952,-8.36590489807333,-11.1058515767196));
#52199=CARTESIAN_POINT('Ctrl Pts',(21.5194458983524,-9.22680492945096,-10.4167337199079));
#52200=CARTESIAN_POINT('Ctrl Pts',(22.243344548252,-9.83277155091188,-9.84187194559463));
#52201=CARTESIAN_POINT('Ctrl Pts',(23.3780871572094,-10.71385497485,-8.87822042993801));
#52202=CARTESIAN_POINT('Ctrl Pts',(24.0312127056184,-11.2033753376215,-8.24209808616164));
#52203=CARTESIAN_POINT('Ctrl Pts',(24.6419825553303,-11.6420191810575,-7.55950905276451));
#52204=CARTESIAN_POINT('Ctrl Pts',(2.1,-4.38490779991026,-23.2560996148446));
#52205=CARTESIAN_POINT('Ctrl Pts',(2.73333333333333,-4.38490779991026,-23.2560996148446));
#52206=CARTESIAN_POINT('Ctrl Pts',(3.36564008017942,-4.38508116042703,-23.2560287329169));
#52207=CARTESIAN_POINT('Ctrl Pts',(4.12276128472868,-4.38513262027402,-23.2560072996302));
#52208=CARTESIAN_POINT('Ctrl Pts',(4.35699735286594,-4.38230977740128,-23.2565699804445));
#52209=CARTESIAN_POINT('Ctrl Pts',(4.84793951429674,-4.36918210570372,-23.2592057903194));
#52210=CARTESIAN_POINT('Ctrl Pts',(5.73067499683022,-4.33776730212203,-23.2655376571851));
#52211=CARTESIAN_POINT('Ctrl Pts',(6.53611671636356,-4.33658160877012,-23.265767496589));
#52212=CARTESIAN_POINT('Ctrl Pts',(7.15937822818369,-4.39617994653139,-23.2535633235265));
#52213=CARTESIAN_POINT('Ctrl Pts',(7.28702172240692,-4.40896850912345,-23.2510752985911));
#52214=CARTESIAN_POINT('Ctrl Pts',(7.48700530829323,-4.43042311822182,-23.2471037568475));
#52215=CARTESIAN_POINT('Ctrl Pts',(7.68600700139787,-4.45357347133899,-23.2429730262749));
#52216=CARTESIAN_POINT('Ctrl Pts',(8.08835779392234,-4.50421621750767,-23.2340785398084));
#52217=CARTESIAN_POINT('Ctrl Pts',(8.69893195391736,-4.59770266101496,-23.2176455238328));
#52218=CARTESIAN_POINT('Ctrl Pts',(9.38143254163704,-4.74441292400085,-23.1884943501166));
#52219=CARTESIAN_POINT('Ctrl Pts',(9.92343839876597,-4.89580885444304,-23.1549384812191));
#52220=CARTESIAN_POINT('Ctrl Pts',(10.1921791819974,-4.98449489776192,-23.134037511346));
#52221=CARTESIAN_POINT('Ctrl Pts',(10.9469680088848,-5.25628971829095,-23.0679401690825));
#52222=CARTESIAN_POINT('Ctrl Pts',(12.107158260859,-5.8643925878101,-22.9287500587564));
#52223=CARTESIAN_POINT('Ctrl Pts',(13.1093288009718,-6.58246121751017,-22.7337196703867));
#52224=CARTESIAN_POINT('Ctrl Pts',(13.868363784104,-7.13699217373245,-22.5542454574039));
#52225=CARTESIAN_POINT('Ctrl Pts',(14.4658194679741,-7.62110550283362,-22.3938560929523));
#52226=CARTESIAN_POINT('Ctrl Pts',(15.5292195040136,-8.62103895016778,-22.038206914543));
#52227=CARTESIAN_POINT('Ctrl Pts',(16.2561491669276,-9.40122850868889,-21.7197205453348));
#52228=CARTESIAN_POINT('Ctrl Pts',(17.0018532435041,-10.1902220748077,-21.3462154347651));
#52229=CARTESIAN_POINT('Ctrl Pts',(17.5710203116058,-10.8351560227674,-21.0277573312478));
#52230=CARTESIAN_POINT('Ctrl Pts',(18.6068243381709,-12.1143416642866,-20.3346523661785));
#52231=CARTESIAN_POINT('Ctrl Pts',(19.3243654506886,-13.065403566866,-19.7366577355752));
#52232=CARTESIAN_POINT('Ctrl Pts',(20.066678302647,-14.0132094185406,-19.0554988265218));
#52233=CARTESIAN_POINT('Ctrl Pts',(20.6168033619827,-14.7468573051219,-18.5000859105222));
#52234=CARTESIAN_POINT('Ctrl Pts',(21.6393889693043,-16.1640493530773,-17.3047719379402));
#52235=CARTESIAN_POINT('Ctrl Pts',(22.355483248933,-17.162221968649,-16.3084425572014));
#52236=CARTESIAN_POINT('Ctrl Pts',(23.4867251715054,-18.6164016930582,-14.6329535278187));
#52237=CARTESIAN_POINT('Ctrl Pts',(24.1253025812515,-19.4078682665568,-13.5489185574));
#52238=CARTESIAN_POINT('Ctrl Pts',(24.7277223812015,-20.1180951211746,-12.3854414359051));
#52239=CARTESIAN_POINT('Ctrl Pts',(2.1,-6.55725782976191,-32.7737869689125));
#52240=CARTESIAN_POINT('Ctrl Pts',(2.73333333333334,-6.55725782976191,-32.7737869689125));
#52241=CARTESIAN_POINT('Ctrl Pts',(3.36510076549686,-6.55740130038319,-32.7737235429482));
#52242=CARTESIAN_POINT('Ctrl Pts',(4.12169087089434,-6.55744105729207,-32.7737050579337));
#52243=CARTESIAN_POINT('Ctrl Pts',(4.34924984699947,-6.55357866493385,-32.774521358146));
#52244=CARTESIAN_POINT('Ctrl Pts',(4.83585190383048,-6.53530567363434,-32.7784073324155));
#52245=CARTESIAN_POINT('Ctrl Pts',(5.71998614385741,-6.49093149495111,-32.7878690946995));
#52246=CARTESIAN_POINT('Ctrl Pts',(6.54872736208918,-6.48802766186921,-32.7884974133419));
#52247=CARTESIAN_POINT('Ctrl Pts',(7.19750250780191,-6.57627048209899,-32.7694462450512));
#52248=CARTESIAN_POINT('Ctrl Pts',(7.32546084490579,-6.59435371051836,-32.765717554002));
#52249=CARTESIAN_POINT('Ctrl Pts',(7.52891895171438,-6.62522183456192,-32.7596388835674));
#52250=CARTESIAN_POINT('Ctrl Pts',(7.73077307336616,-6.65842767110204,-32.7533193763253));
#52251=CARTESIAN_POINT('Ctrl Pts',(8.14020547050341,-6.73134435356068,-32.7396330973257));
#52252=CARTESIAN_POINT('Ctrl Pts',(8.76327382634538,-6.86633080121424,-32.714277000723));
#52253=CARTESIAN_POINT('Ctrl Pts',(9.46274681600517,-7.07963379346393,-32.6693403316508));
#52254=CARTESIAN_POINT('Ctrl Pts',(10.017614109892,-7.29999454273279,-32.617935281249));
#52255=CARTESIAN_POINT('Ctrl Pts',(10.2918722028545,-7.42879902723335,-32.586110997956));
#52256=CARTESIAN_POINT('Ctrl Pts',(11.0596479948439,-7.8223339461195,-32.4860007673529));
#52257=CARTESIAN_POINT('Ctrl Pts',(12.211331411252,-8.67991526033185,-32.2795014435999));
#52258=CARTESIAN_POINT('Ctrl Pts',(13.2034376761732,-9.67994219031867,-31.9958455494954));
#52259=CARTESIAN_POINT('Ctrl Pts',(13.9587869858217,-10.4565075782823,-31.7345428390373));
#52260=CARTESIAN_POINT('Ctrl Pts',(14.5428320694722,-11.1220898054817,-31.5063608409992));
#52261=CARTESIAN_POINT('Ctrl Pts',(15.5915904941101,-12.5049041760033,-30.9987636124804));
#52262=CARTESIAN_POINT('Ctrl Pts',(16.3123392972128,-13.5898788951704,-30.5438307640613));
#52263=CARTESIAN_POINT('Ctrl Pts',(17.0563791111118,-14.6955951922712,-30.0067575635175));
#52264=CARTESIAN_POINT('Ctrl Pts',(17.6163059289884,-15.5819349355565,-29.5590986201794));
#52265=CARTESIAN_POINT('Ctrl Pts',(18.6451985583325,-17.3599656796549,-28.5761389977681));
#52266=CARTESIAN_POINT('Ctrl Pts',(19.3594303438975,-18.6865488395582,-27.7271731514842));
#52267=CARTESIAN_POINT('Ctrl Pts',(20.1009222175396,-20.0151479025086,-26.7556821733498));
#52268=CARTESIAN_POINT('Ctrl Pts',(20.6466402308937,-21.030426465412,-25.9748073051926));
#52269=CARTESIAN_POINT('Ctrl Pts',(21.6664010977576,-23.0078930048959,-24.2829755073075));
#52270=CARTESIAN_POINT('Ctrl Pts',(22.3810504024336,-24.4030893583186,-22.8712638027695));
#52271=CARTESIAN_POINT('Ctrl Pts',(23.5117580694457,-26.4396142021185,-20.4918798317284));
#52272=CARTESIAN_POINT('Ctrl Pts',(24.1480627906507,-27.5389977546928,-18.9644924777646));
#52273=CARTESIAN_POINT('Ctrl Pts',(24.7493903499091,-28.5277151370773,-17.3227988978198));
#52274=CARTESIAN_POINT('Ctrl Pts',(2.1,-7.79860070396284,-38.2124654569512));
#52275=CARTESIAN_POINT('Ctrl Pts',(2.73333333333333,-7.79860070396284,-38.2124654569512));
#52276=CARTESIAN_POINT('Ctrl Pts',(3.36477451767734,-7.79872668178171,-38.2124076368945));
#52277=CARTESIAN_POINT('Ctrl Pts',(4.12105795390395,-7.79875982746218,-38.2123912207539));
#52278=CARTESIAN_POINT('Ctrl Pts',(4.34479378544621,-7.79433071314039,-38.2133462736395));
#52279=CARTESIAN_POINT('Ctrl Pts',(4.82895151376368,-7.77317986564745,-38.2179328211141));
#52280=CARTESIAN_POINT('Ctrl Pts',(5.71377591256104,-7.72136220442836,-38.2291918165454));
#52281=CARTESIAN_POINT('Ctrl Pts',(6.55607299317545,-7.71728578679096,-38.2300939740762));
#52282=CARTESIAN_POINT('Ctrl Pts',(7.21869808515308,-7.82274179205237,-38.2069365723915));
#52283=CARTESIAN_POINT('Ctrl Pts',(7.34682327184808,-7.84386203725498,-38.2024959214673));
#52284=CARTESIAN_POINT('Ctrl Pts',(7.55214855896988,-7.8802299041422,-38.1951848870786));
#52285=CARTESIAN_POINT('Ctrl Pts',(7.75551147978984,-7.91928693575672,-38.1875896312606));
#52286=CARTESIAN_POINT('Ctrl Pts',(8.16865455442754,-8.00519656802901,-38.1711016701523));
#52287=CARTESIAN_POINT('Ctrl Pts',(8.79801144190279,-8.16440073086343,-38.1405254358603));
#52288=CARTESIAN_POINT('Ctrl Pts',(9.50498474714468,-8.41625819933518,-38.0864351163565));
#52289=CARTESIAN_POINT('Ctrl Pts',(10.0643900034903,-8.67568279563254,-38.024902443149));
#52290=CARTESIAN_POINT('Ctrl Pts',(10.3401121837103,-8.82680225521101,-37.9869846363453));
#52291=CARTESIAN_POINT('Ctrl Pts',(11.1102644279334,-9.28727841432574,-37.868102320491));
#52292=CARTESIAN_POINT('Ctrl Pts',(12.2545468430399,-10.2798783318648,-37.6252922831318));
#52293=CARTESIAN_POINT('Ctrl Pts',(13.2428517544314,-11.4392785377615,-37.2919891637173));
#52294=CARTESIAN_POINT('Ctrl Pts',(13.9963939127891,-12.3419444861523,-36.9844996268006));
#52295=CARTESIAN_POINT('Ctrl Pts',(14.5753802005105,-13.1095340012662,-36.7184795152973));
#52296=CARTESIAN_POINT('Ctrl Pts',(15.6192625879179,-14.7118683070092,-36.1244593262902));
#52297=CARTESIAN_POINT('Ctrl Pts',(16.3374020123066,-15.9713792188489,-35.5919214093329));
#52298=CARTESIAN_POINT('Ctrl Pts',(17.0806356432168,-17.2581947700535,-34.9618903427716));
#52299=CARTESIAN_POINT('Ctrl Pts',(17.6370189134984,-18.2837979918633,-34.4401616107928));
#52300=CARTESIAN_POINT('Ctrl Pts',(18.6628099255013,-20.3488100760065,-33.291180187705));
#52301=CARTESIAN_POINT('Ctrl Pts',(19.3754696037404,-21.8905313156091,-32.2990136429051));
#52302=CARTESIAN_POINT('Ctrl Pts',(20.1166288096483,-23.4369295004069,-31.1620681816041));
#52303=CARTESIAN_POINT('Ctrl Pts',(20.6600107888588,-24.6143015822174,-30.2519047078682));
#52304=CARTESIAN_POINT('Ctrl Pts',(21.677799407356,-26.9129383770149,-28.276094543497));
#52305=CARTESIAN_POINT('Ctrl Pts',(22.3918093779893,-28.5354767163545,-26.6272808649087));
#52306=CARTESIAN_POINT('Ctrl Pts',(23.5225085832192,-30.905250682406,-23.8461862521349));
#52307=CARTESIAN_POINT('Ctrl Pts',(24.157514841919,-32.1813366627448,-22.0653831262647));
#52308=CARTESIAN_POINT('Ctrl Pts',(24.7577717974218,-33.3295007473295,-20.1503690732212));
#52309=CARTESIAN_POINT('',(24.5,-7.98533675018927,-5.53162409676021));
#52310=CARTESIAN_POINT('Ctrl Pts',(24.5,-7.98533675018927,-5.53162409676021));
#52311=CARTESIAN_POINT('Ctrl Pts',(23.8274939346105,-7.79179330153433,-6.14100658734753));
#52312=CARTESIAN_POINT('Ctrl Pts',(23.3366347313968,-7.64970961728591,-6.56481136530389));
#52313=CARTESIAN_POINT('Ctrl Pts',(22.5855494187791,-7.42734387677876,-7.22058552996049));
#52314=CARTESIAN_POINT('Ctrl Pts',(22.2454144274572,-7.32664377261339,-7.51755810558866));
#52315=CARTESIAN_POINT('Ctrl Pts',(21.8382660749244,-7.19700906555054,-7.88116210508794));
#52316=CARTESIAN_POINT('Ctrl Pts',(21.3802156956577,-7.04734131796725,-8.29760563162483));
#52317=CARTESIAN_POINT('Ctrl Pts',(20.7694693297003,-6.84778022801936,-8.85287505606244));
#52318=CARTESIAN_POINT('Ctrl Pts',(20.1629003035383,-6.64759826746033,-9.41330941265572));
#52319=CARTESIAN_POINT('Ctrl Pts',(19.5574857571565,-6.47402412338126,-9.98319848690682));
#52320=CARTESIAN_POINT('Ctrl Pts',(18.641852941883,-6.2115094825428,-10.8451023519009));
#52321=CARTESIAN_POINT('Ctrl Pts',(17.7734813325897,-5.92779326145821,-11.7477852370966));
#52322=CARTESIAN_POINT('Ctrl Pts',(16.9621253116777,-5.71558340812137,-12.6333016467232));
#52323=CARTESIAN_POINT('Ctrl Pts',(16.8133360673648,-5.67666763884139,-12.7956906769628));
#52324=CARTESIAN_POINT('Ctrl Pts',(16.6656205371618,-5.63959048888305,-12.9586217386495));
#52325=CARTESIAN_POINT('Ctrl Pts',(16.5183901926363,-5.60441931851976,-13.1227300282793));
#52326=CARTESIAN_POINT('Ctrl Pts',(15.726452288601,-5.41523696599741,-14.0054527804615));
#52327=CARTESIAN_POINT('Ctrl Pts',(14.9462259717426,-5.20042309417513,-14.9632129988162));
#52328=CARTESIAN_POINT('Ctrl Pts',(14.2963150412798,-5.06317274092078,-15.7944759718845));
#52329=CARTESIAN_POINT('Ctrl Pts',(13.9908350932728,-4.99866046883726,-16.1851974660009));
#52330=CARTESIAN_POINT('Ctrl Pts',(13.7077063566251,-4.94733703640913,-16.556124793982));
#52331=CARTESIAN_POINT('Ctrl Pts',(13.4460198946299,-4.90799662279406,-16.905002605579));
#52332=CARTESIAN_POINT('Ctrl Pts',(12.8373295399395,-4.81648967155765,-17.7165025863783));
#52333=CARTESIAN_POINT('Ctrl Pts',(12.3530827400008,-4.74153986672384,-18.4095331888858));
#52334=CARTESIAN_POINT('Ctrl Pts',(11.977027567753,-4.69720924336388,-18.958655074939));
#52335=CARTESIAN_POINT('Ctrl Pts',(11.655397242359,-4.65929440036105,-19.4283049133829));
#52336=CARTESIAN_POINT('Ctrl Pts',(11.368420561205,-4.63402086471352,-19.8589729704981));
#52337=CARTESIAN_POINT('Ctrl Pts',(11.0710856781053,-4.62105342435355,-20.3157155446813));
#52338=CARTESIAN_POINT('Ctrl Pts',(10.8141787015478,-4.60984913556699,-20.7103559332398));
#52339=CARTESIAN_POINT('Ctrl Pts',(10.5576802661741,-4.60874384919066,-21.1126900533831));
#52340=CARTESIAN_POINT('Ctrl Pts',(10.2957959918397,-4.62202135570263,-21.5329760085416));
#52341=CARTESIAN_POINT('Ctrl Pts',(9.71459276345479,-4.65148830124287,-22.4657221789779));
#52342=CARTESIAN_POINT('Ctrl Pts',(9.09527967376712,-4.74839217740081,-23.5049560069573));
#52343=CARTESIAN_POINT('Ctrl Pts',(8.43168033653304,-4.91177772174176,-24.7156496305248));
#52344=CARTESIAN_POINT('Ctrl Pts',(7.97964340480655,-5.02307424663008,-25.5403614711655));
#52345=CARTESIAN_POINT('Ctrl Pts',(7.52291961074554,-5.16302904003053,-26.4199423107392));
#52346=CARTESIAN_POINT('Ctrl Pts',(7.10363554125515,-5.30796452319851,-27.2733711087693));
#52347=CARTESIAN_POINT('Ctrl Pts',(6.56327799556932,-5.49475192502499,-28.3732380588341));
#52348=CARTESIAN_POINT('Ctrl Pts',(6.08559840026265,-5.72631856597084,-29.4106367559605));
#52349=CARTESIAN_POINT('Ctrl Pts',(5.61708670833696,-5.98368137431826,-30.4930591500792));
#52350=CARTESIAN_POINT('Ctrl Pts',(5.04102956506852,-6.30012104213272,-31.8239483528715));
#52351=CARTESIAN_POINT('Ctrl Pts',(4.50102820504748,-6.64971333190113,-33.1788609907931));
#52352=CARTESIAN_POINT('Ctrl Pts',(4.,-6.96288805731186,-34.5509691145741));
#52353=CARTESIAN_POINT('Ctrl Pts',(3.72183418896936,-7.13675950927916,-35.3127497193948));
#52354=CARTESIAN_POINT('Ctrl Pts',(3.45538353518157,-7.31144697863298,-36.0781055299851));
#52355=CARTESIAN_POINT('Ctrl Pts',(3.2,-7.48695481785668,-36.8470556158206));
#52356=CARTESIAN_POINT('',(24.5,-22.711314109499,-14.6012400644491));
#52357=CARTESIAN_POINT('Ctrl Pts',(24.5,-22.7113141094989,-14.6012400644491));
#52358=CARTESIAN_POINT('Ctrl Pts',(24.5,-21.6612444285481,-13.9441972658053));
#52359=CARTESIAN_POINT('Ctrl Pts',(24.5,-20.6284979425513,-13.2990592550798));
#52360=CARTESIAN_POINT('Ctrl Pts',(24.5,-16.3584140276965,-10.6372840649079));
#52361=CARTESIAN_POINT('Ctrl Pts',(24.5,-11.8204260321014,-7.81894043060838));
#52362=CARTESIAN_POINT('Ctrl Pts',(24.5,-7.98533675018928,-5.53162409676021));
#52363=CARTESIAN_POINT('',(10.2670750393577,-7.59968099677392,-33.2963779888109));
#52364=CARTESIAN_POINT('Ctrl Pts',(10.2670750393577,-7.59968099677392,-33.2963779888109));
#52365=CARTESIAN_POINT('Ctrl Pts',(11.2293198185888,-7.85751093220376,-32.3343749713692));
#52366=CARTESIAN_POINT('Ctrl Pts',(12.092802582344,-8.36505042380101,-31.4950825542866));
#52367=CARTESIAN_POINT('Ctrl Pts',(14.3080979519049,-9.99690083383536,-29.3617204319546));
#52368=CARTESIAN_POINT('Ctrl Pts',(14.8952017874601,-10.5394379824431,-28.8060939602778));
#52369=CARTESIAN_POINT('Ctrl Pts',(17.0803363586062,-12.930959939454,-26.4724118333468));
#52370=CARTESIAN_POINT('Ctrl Pts',(17.6922811489506,-13.6632420748191,-25.7681575791701));
#52371=CARTESIAN_POINT('Ctrl Pts',(19.0755427322033,-15.4528573288732,-24.0359413364337));
#52372=CARTESIAN_POINT('Ctrl Pts',(20.2687424742408,-17.037585857733,-22.4580909086129));
#52373=CARTESIAN_POINT('Ctrl Pts',(22.3267279388309,-19.9349590187757,-18.9782950332083));
#52374=CARTESIAN_POINT('Ctrl Pts',(23.4192562717209,-21.3897764892588,-16.9977385665951));
#52375=CARTESIAN_POINT('Ctrl Pts',(24.5,-22.7113141094989,-14.6012400644491));
#52376=CARTESIAN_POINT('Ctrl Pts',(6.,-7.72847464911698,-38.226570335278));
#52377=CARTESIAN_POINT('Ctrl Pts',(7.51604047332548,-7.25149509435605,-36.1223672378383));
#52378=CARTESIAN_POINT('Ctrl Pts',(9.08449301626627,-7.38041248529,-34.500587661922));
#52379=CARTESIAN_POINT('Ctrl Pts',(9.8624969752411,-7.50317632397629,-33.7027132752924));
#52380=CARTESIAN_POINT('Ctrl Pts',(10.0667253012217,-7.54599802424764,-33.4966773895357));
#52381=CARTESIAN_POINT('Ctrl Pts',(10.2670750393577,-7.59968099677392,-33.2963779888109));
#52382=CARTESIAN_POINT('Origin',(24.5,-1.89142793862867,-8.2868872535455));
#52383=CARTESIAN_POINT('',(24.5,-9.13966689904905,-3.29104195297002));
#52384=CARTESIAN_POINT('Ctrl Pts',(24.5,-9.13966689904905,-3.29104195297002));
#52385=CARTESIAN_POINT('Ctrl Pts',(24.5,-9.07110398184028,-3.48145041140664));
#52386=CARTESIAN_POINT('Ctrl Pts',(24.5,-8.99656198952293,-3.66979647783168));
#52387=CARTESIAN_POINT('Ctrl Pts',(24.5,-8.66176238807634,-4.44398568939236));
#52388=CARTESIAN_POINT('Ctrl Pts',(24.5,-8.34993106747065,-5.00530337254428));
#52389=CARTESIAN_POINT('Ctrl Pts',(24.5,-7.98533675018927,-5.53162409676021));
#52390=CARTESIAN_POINT('',(24.5,-25.1047038636482,-9.93749686382478));
#52391=CARTESIAN_POINT('Ctrl Pts',(24.5,-9.13966689904905,-3.29104195297002));
#52392=CARTESIAN_POINT('Ctrl Pts',(24.5,-13.0912453003007,-5.00666635927105));
#52393=CARTESIAN_POINT('Ctrl Pts',(24.5,-18.4037408367292,-7.20260295357725));
#52394=CARTESIAN_POINT('Ctrl Pts',(24.5,-25.1047038636482,-9.93749686382477));
#52395=CARTESIAN_POINT('Origin',(24.5,0.,0.));
#52396=CARTESIAN_POINT('Ctrl Pts',(24.5,-25.1047039675821,-9.93749660126077));
#52397=CARTESIAN_POINT('Ctrl Pts',(24.5,-19.8711159090285,-23.1589027732729));
#52398=CARTESIAN_POINT('Ctrl Pts',(24.5,-6.00806521682049,-26.3230536289092));
#52399=CARTESIAN_POINT('Ctrl Pts',(24.5,20.3149884120887,-32.3311188457297));
#52400=CARTESIAN_POINT('Ctrl Pts',(24.5,26.3230536289092,-6.00806521682049));
#52401=CARTESIAN_POINT('Ctrl Pts',(24.5,32.3311188457297,20.3149884120887));
#52402=CARTESIAN_POINT('Ctrl Pts',(24.5,6.00806521682049,26.3230536289092));
#52403=CARTESIAN_POINT('Ctrl Pts',(24.5,-20.3149884120887,32.3311188457297));
#52404=CARTESIAN_POINT('Ctrl Pts',(24.5,-26.3230536289092,6.00806521682049));
#52405=CARTESIAN_POINT('Ctrl Pts',(24.5,-28.1858992943483,-2.15359491570446));
#52406=CARTESIAN_POINT('Ctrl Pts',(24.5,-25.1047039675821,-9.93749660126077));
#52407=CARTESIAN_POINT('Ctrl Pts',(24.3078118955742,-25.1351889338974,-9.9495638317503));
#52408=CARTESIAN_POINT('Ctrl Pts',(24.3078118955742,-19.89524566176,-23.1870249280633));
#52409=CARTESIAN_POINT('Ctrl Pts',(24.3078118955742,-6.01536088802186,-26.3550180529563));
#52410=CARTESIAN_POINT('Ctrl Pts',(24.3078118955742,20.3396571649344,-32.3703789409781));
#52411=CARTESIAN_POINT('Ctrl Pts',(24.3078118955742,26.3550180529563,-6.01536088802186));
#52412=CARTESIAN_POINT('Ctrl Pts',(24.3078118955742,32.3703789409781,20.3396571649344));
#52413=CARTESIAN_POINT('Ctrl Pts',(24.3078118955742,6.01536088802186,26.3550180529563));
#52414=CARTESIAN_POINT('Ctrl Pts',(24.3078118955742,-20.3396571649344,32.3703789409781));
#52415=CARTESIAN_POINT('Ctrl Pts',(24.3078118955742,-26.3550180529563,6.01536088802186));
#52416=CARTESIAN_POINT('Ctrl Pts',(24.3078118955742,-28.22012579595,-2.15621005382945));
#52417=CARTESIAN_POINT('Ctrl Pts',(24.3078118955742,-25.1351889338974,-9.9495638317503));
#52418=CARTESIAN_POINT('Ctrl Pts',(23.9225830034177,-25.2000312537492,-9.97523114628931));
#52419=CARTESIAN_POINT('Ctrl Pts',(23.9225830034177,-19.9465702762725,-23.2468414860669));
#52420=CARTESIAN_POINT('Ctrl Pts',(23.9225830034177,-6.03087897128556,-26.4230072180579));
#52421=CARTESIAN_POINT('Ctrl Pts',(23.9225830034177,20.3921282467724,-32.4538861893435));
#52422=CARTESIAN_POINT('Ctrl Pts',(23.9225830034177,26.4230072180579,-6.03087897128556));
#52423=CARTESIAN_POINT('Ctrl Pts',(23.9225830034177,32.4538861893435,20.3921282467724));
#52424=CARTESIAN_POINT('Ctrl Pts',(23.9225830034177,6.03087897128556,26.4230072180579));
#52425=CARTESIAN_POINT('Ctrl Pts',(23.9225830034177,-20.3921282467724,32.4538861893435));
#52426=CARTESIAN_POINT('Ctrl Pts',(23.9225830034177,-26.4230072180579,6.03087897128556));
#52427=CARTESIAN_POINT('Ctrl Pts',(23.9225830034177,-28.2929264591131,-2.16177252094858));
#52428=CARTESIAN_POINT('Ctrl Pts',(23.9225830034177,-25.2000312537492,-9.97523114628931));
#52429=CARTESIAN_POINT('Ctrl Pts',(23.3421815947946,-25.3089118559866,-10.0183306632593));
#52430=CARTESIAN_POINT('Ctrl Pts',(23.3421815947946,-20.0327524941588,-23.3472830321759));
#52431=CARTESIAN_POINT('Ctrl Pts',(23.3421815947946,-6.05693630938179,-26.5371718756275));
#52432=CARTESIAN_POINT('Ctrl Pts',(23.3421815947946,20.4802355662457,-32.5941081850093));
#52433=CARTESIAN_POINT('Ctrl Pts',(23.3421815947946,26.5371718756275,-6.05693630938179));
#52434=CARTESIAN_POINT('Ctrl Pts',(23.3421815947946,32.5941081850093,20.4802355662457));
#52435=CARTESIAN_POINT('Ctrl Pts',(23.3421815947946,6.05693630938179,26.5371718756275));
#52436=CARTESIAN_POINT('Ctrl Pts',(23.3421815947946,-20.4802355662457,32.5941081850093));
#52437=CARTESIAN_POINT('Ctrl Pts',(23.3421815947946,-26.5371718756275,6.05693630938179));
#52438=CARTESIAN_POINT('Ctrl Pts',(23.3421815947946,-28.4151703897221,-2.17111279087171));
#52439=CARTESIAN_POINT('Ctrl Pts',(23.3421815947946,-25.3089118559866,-10.0183306632593));
#52440=CARTESIAN_POINT('Ctrl Pts',(22.5631762070947,-25.4774153713825,-10.0850314343064));
#52441=CARTESIAN_POINT('Ctrl Pts',(22.5631762070947,-20.1661280117444,-23.5027262724168));
#52442=CARTESIAN_POINT('Ctrl Pts',(22.5631762070947,-6.09726262078023,-26.7138529899778));
#52443=CARTESIAN_POINT('Ctrl Pts',(22.5631762070947,20.6165903691975,-32.811115610758));
#52444=CARTESIAN_POINT('Ctrl Pts',(22.5631762070947,26.7138529899778,-6.09726262078023));
#52445=CARTESIAN_POINT('Ctrl Pts',(22.5631762070947,32.811115610758,20.6165903691975));
#52446=CARTESIAN_POINT('Ctrl Pts',(22.5631762070947,6.09726262078023,26.7138529899778));
#52447=CARTESIAN_POINT('Ctrl Pts',(22.5631762070947,-20.6165903691975,32.811115610758));
#52448=CARTESIAN_POINT('Ctrl Pts',(22.5631762070947,-26.7138529899778,6.09726262078023));
#52449=CARTESIAN_POINT('Ctrl Pts',(22.5631762070947,-28.6043549792646,-2.18556778362938));
#52450=CARTESIAN_POINT('Ctrl Pts',(22.5631762070947,-25.4774153713825,-10.0850314343064));
#52451=CARTESIAN_POINT('Ctrl Pts',(21.5808622776984,-25.7276079592011,-10.1840681723743));
#52452=CARTESIAN_POINT('Ctrl Pts',(21.5808622776984,-20.3641628469109,-23.7335270746635));
#52453=CARTESIAN_POINT('Ctrl Pts',(21.5808622776984,-6.15713878527594,-26.9761876072355));
#52454=CARTESIAN_POINT('Ctrl Pts',(21.5808622776984,20.8190488219595,-33.1333263925114));
#52455=CARTESIAN_POINT('Ctrl Pts',(21.5808622776984,26.9761876072355,-6.15713878527594));
#52456=CARTESIAN_POINT('Ctrl Pts',(21.5808622776984,33.1333263925114,20.8190488219595));
#52457=CARTESIAN_POINT('Ctrl Pts',(21.5808622776984,6.15713878527594,26.9761876072355));
#52458=CARTESIAN_POINT('Ctrl Pts',(21.5808622776984,-20.8190488219595,33.1333263925114));
#52459=CARTESIAN_POINT('Ctrl Pts',(21.5808622776984,-26.9761876072355,6.15713878527594));
#52460=CARTESIAN_POINT('Ctrl Pts',(21.5808622776984,-28.8852546502407,-2.20703043404616));
#52461=CARTESIAN_POINT('Ctrl Pts',(21.5808622776984,-25.7276079592011,-10.1840681723743));
#52462=CARTESIAN_POINT('Ctrl Pts',(20.5902243197586,-26.0184347228058,-10.2991896244579));
#52463=CARTESIAN_POINT('Ctrl Pts',(20.5902243197586,-20.5943608343677,-24.0018126019847));
#52464=CARTESIAN_POINT('Ctrl Pts',(20.5902243197586,-6.22673953280079,-27.2811284065763));
#52465=CARTESIAN_POINT('Ctrl Pts',(20.5902243197586,21.0543888737755,-33.5078679393771));
#52466=CARTESIAN_POINT('Ctrl Pts',(20.5902243197586,27.2811284065763,-6.22673953280079));
#52467=CARTESIAN_POINT('Ctrl Pts',(20.5902243197586,33.5078679393771,21.0543888737755));
#52468=CARTESIAN_POINT('Ctrl Pts',(20.5902243197586,6.22673953280079,27.2811284065763));
#52469=CARTESIAN_POINT('Ctrl Pts',(20.5902243197586,-21.0543888737755,33.5078679393771));
#52470=CARTESIAN_POINT('Ctrl Pts',(20.5902243197586,-27.2811284065763,6.22673953280079));
#52471=CARTESIAN_POINT('Ctrl Pts',(20.5902243197586,-29.2117756831773,-2.23197886762493));
#52472=CARTESIAN_POINT('Ctrl Pts',(20.5902243197586,-26.0184347228058,-10.2991896244579));
#52473=CARTESIAN_POINT('Ctrl Pts',(19.591895069338,-26.3512694502151,-10.4309395935745));
#52474=CARTESIAN_POINT('Ctrl Pts',(19.591895069338,-20.8578093679748,-24.3088501636144));
#52475=CARTESIAN_POINT('Ctrl Pts',(19.591895069338,-6.30639363871179,-27.6301158469569));
#52476=CARTESIAN_POINT('Ctrl Pts',(19.591895069338,21.3237222082451,-33.9365094856687));
#52477=CARTESIAN_POINT('Ctrl Pts',(19.591895069338,27.6301158469569,-6.30639363871179));
#52478=CARTESIAN_POINT('Ctrl Pts',(19.591895069338,33.9365094856687,21.3237222082451));
#52479=CARTESIAN_POINT('Ctrl Pts',(19.591895069338,6.30639363871179,27.6301158469569));
#52480=CARTESIAN_POINT('Ctrl Pts',(19.591895069338,-21.3237222082451,33.9365094856687));
#52481=CARTESIAN_POINT('Ctrl Pts',(19.591895069338,-27.6301158469569,6.30639363871179));
#52482=CARTESIAN_POINT('Ctrl Pts',(19.591895069338,-29.5854604762956,-2.26053093410794));
#52483=CARTESIAN_POINT('Ctrl Pts',(19.591895069338,-26.3512694502151,-10.4309395935745));
#52484=CARTESIAN_POINT('Ctrl Pts',(18.5871162949016,-26.7276913580337,-10.5799432000069));
#52485=CARTESIAN_POINT('Ctrl Pts',(18.5871162949016,-21.1557584443957,-24.6560965751298));
#52486=CARTESIAN_POINT('Ctrl Pts',(18.5871162949016,-6.39647904159621,-28.0248057855197));
#52487=CARTESIAN_POINT('Ctrl Pts',(18.5871162949016,21.6283267439235,-34.4212848271159));
#52488=CARTESIAN_POINT('Ctrl Pts',(18.5871162949016,28.0248057855197,-6.39647904159621));
#52489=CARTESIAN_POINT('Ctrl Pts',(18.5871162949016,34.4212848271159,21.6283267439235));
#52490=CARTESIAN_POINT('Ctrl Pts',(18.5871162949016,6.39647904159621,28.0248057855197));
#52491=CARTESIAN_POINT('Ctrl Pts',(18.5871162949016,-21.6283267439235,34.4212848271159));
#52492=CARTESIAN_POINT('Ctrl Pts',(18.5871162949016,-28.0248057855197,6.39647904159621));
#52493=CARTESIAN_POINT('Ctrl Pts',(18.5871162949016,-30.0080820694305,-2.29282210582957));
#52494=CARTESIAN_POINT('Ctrl Pts',(18.5871162949016,-26.7276913580337,-10.5799432000069));
#52495=CARTESIAN_POINT('Ctrl Pts',(17.577868433379,-27.149299963076,-10.7468335997137));
#52496=CARTESIAN_POINT('Ctrl Pts',(17.577868433379,-21.4894741285104,-25.045027378901));
#52497=CARTESIAN_POINT('Ctrl Pts',(17.577868433379,-6.49737853829363,-28.4668753648014));
#52498=CARTESIAN_POINT('Ctrl Pts',(17.577868433379,21.9694968265077,-34.964253903095));
#52499=CARTESIAN_POINT('Ctrl Pts',(17.577868433379,28.4668753648014,-6.49737853829363));
#52500=CARTESIAN_POINT('Ctrl Pts',(17.577868433379,34.964253903095,21.9694968265077));
#52501=CARTESIAN_POINT('Ctrl Pts',(17.577868433379,6.49737853829363,28.4668753648014));
#52502=CARTESIAN_POINT('Ctrl Pts',(17.577868433379,-21.9694968265077,34.964253903095));
#52503=CARTESIAN_POINT('Ctrl Pts',(17.577868433379,-28.4668753648014,6.49737853829363));
#52504=CARTESIAN_POINT('Ctrl Pts',(17.577868433379,-30.4814362941487,-2.32898959656791));
#52505=CARTESIAN_POINT('Ctrl Pts',(17.577868433379,-27.149299963076,-10.7468335997137));
#52506=CARTESIAN_POINT('Ctrl Pts',(16.5668667015923,-27.617432585777,-10.9321401603104));
#52507=CARTESIAN_POINT('Ctrl Pts',(16.5668667015923,-21.8600149490077,-25.4768762430872));
#52508=CARTESIAN_POINT('Ctrl Pts',(16.5668667015923,-6.60941217672811,-28.9577268063763));
#52509=CARTESIAN_POINT('Ctrl Pts',(16.5668667015923,22.3483146296482,-35.5671389831044));
#52510=CARTESIAN_POINT('Ctrl Pts',(16.5668667015923,28.9577268063763,-6.60941217672811));
#52511=CARTESIAN_POINT('Ctrl Pts',(16.5668667015923,35.5671389831044,22.3483146296482));
#52512=CARTESIAN_POINT('Ctrl Pts',(16.5668667015923,6.60941217672811,28.9577268063763));
#52513=CARTESIAN_POINT('Ctrl Pts',(16.5668667015923,-22.3483146296482,35.5671389831044));
#52514=CARTESIAN_POINT('Ctrl Pts',(16.5668667015923,-28.9577268063763,6.60941217672811));
#52515=CARTESIAN_POINT('Ctrl Pts',(16.5668667015923,-31.007024605283,-2.36914812771116));
#52516=CARTESIAN_POINT('Ctrl Pts',(16.5668667015923,-27.617432585777,-10.9321401603104));
#52517=CARTESIAN_POINT('Ctrl Pts',(15.5576189940876,-28.1328325376183,-11.1361571157115));
#52518=CARTESIAN_POINT('Ctrl Pts',(15.5576189940876,-22.2679692589159,-25.952328867004));
#52519=CARTESIAN_POINT('Ctrl Pts',(15.5576189940876,-6.73275784642441,-29.4981394951766));
#52520=CARTESIAN_POINT('Ctrl Pts',(15.5576189940876,22.7653816487522,-36.230897341601));
#52521=CARTESIAN_POINT('Ctrl Pts',(15.5576189940876,29.4981394951766,-6.73275784642441));
#52522=CARTESIAN_POINT('Ctrl Pts',(15.5576189940876,36.230897341601,22.7653816487522));
#52523=CARTESIAN_POINT('Ctrl Pts',(15.5576189940876,6.73275784642441,29.4981394951766));
#52524=CARTESIAN_POINT('Ctrl Pts',(15.5576189940876,-22.7653816487522,36.230897341601));
#52525=CARTESIAN_POINT('Ctrl Pts',(15.5576189940876,-29.4981394951766,6.73275784642441));
#52526=CARTESIAN_POINT('Ctrl Pts',(15.5576189940876,-31.5856815437464,-2.41336146387609));
#52527=CARTESIAN_POINT('Ctrl Pts',(15.5576189940876,-28.1328325376183,-11.1361571157115));
#52528=CARTESIAN_POINT('Ctrl Pts',(14.5544447688713,-28.6953342065352,-11.3588189097037));
#52529=CARTESIAN_POINT('Ctrl Pts',(14.5544447688713,-22.7132059713864,-26.4712324747531));
#52530=CARTESIAN_POINT('Ctrl Pts',(14.5544447688713,-6.86737591305398,-30.0879397818628));
#52531=CARTESIAN_POINT('Ctrl Pts',(14.5544447688713,23.2205638688088,-36.9553156949167));
#52532=CARTESIAN_POINT('Ctrl Pts',(14.5544447688713,30.0879397818628,-6.86737591305398));
#52533=CARTESIAN_POINT('Ctrl Pts',(14.5544447688713,36.9553156949167,23.2205638688088));
#52534=CARTESIAN_POINT('Ctrl Pts',(14.5544447688713,6.86737591305398,30.0879397818628));
#52535=CARTESIAN_POINT('Ctrl Pts',(14.5544447688713,-23.2205638688088,36.9553156949167));
#52536=CARTESIAN_POINT('Ctrl Pts',(14.5544447688713,-30.0879397818628,6.86737591305398));
#52537=CARTESIAN_POINT('Ctrl Pts',(14.5544447688713,-32.2172211712787,-2.46161539811165));
#52538=CARTESIAN_POINT('Ctrl Pts',(14.5544447688713,-28.6953342065352,-11.3588189097037));
#52539=CARTESIAN_POINT('Ctrl Pts',(13.5625963827217,-29.303338426322,-11.599492525114));
#52540=CARTESIAN_POINT('Ctrl Pts',(13.5625963827217,-23.1944592990561,-27.0321118473983));
#52541=CARTESIAN_POINT('Ctrl Pts',(13.5625963827217,-7.01288366368501,-30.7254508915224));
#52542=CARTESIAN_POINT('Ctrl Pts',(13.5625963827217,23.7125672278374,-37.7383345552074));
#52543=CARTESIAN_POINT('Ctrl Pts',(13.5625963827217,30.7254508915224,-7.01288366368501));
#52544=CARTESIAN_POINT('Ctrl Pts',(13.5625963827217,37.7383345552074,23.7125672278374));
#52545=CARTESIAN_POINT('Ctrl Pts',(13.5625963827217,7.01288366368501,30.7254508915224));
#52546=CARTESIAN_POINT('Ctrl Pts',(13.5625963827217,-23.7125672278374,37.7383345552074));
#52547=CARTESIAN_POINT('Ctrl Pts',(13.5625963827217,-30.7254508915224,7.01288366368501));
#52548=CARTESIAN_POINT('Ctrl Pts',(13.5625963827217,-32.8998480499537,-2.51377274671653));
#52549=CARTESIAN_POINT('Ctrl Pts',(13.5625963827217,-29.303338426322,-11.599492525114));
#52550=CARTESIAN_POINT('Ctrl Pts',(12.5880795783847,-29.953804607069,-11.8569743687062));
#52551=CARTESIAN_POINT('Ctrl Pts',(12.5880795783847,-23.7093225250562,-27.6321620633528));
#52552=CARTESIAN_POINT('Ctrl Pts',(12.5880795783847,-7.16855342343643,-31.4074846721918));
#52553=CARTESIAN_POINT('Ctrl Pts',(12.5880795783847,24.2389312487553,-38.5760380956282));
#52554=CARTESIAN_POINT('Ctrl Pts',(12.5880795783847,31.4074846721918,-7.16855342343643));
#52555=CARTESIAN_POINT('Ctrl Pts',(12.5880795783847,38.5760380956282,24.2389312487553));
#52556=CARTESIAN_POINT('Ctrl Pts',(12.5880795783847,7.16855342343643,31.4074846721918));
#52557=CARTESIAN_POINT('Ctrl Pts',(12.5880795783847,-24.2389312487553,38.5760380956282));
#52558=CARTESIAN_POINT('Ctrl Pts',(12.5880795783847,-31.4074846721918,7.16855342343643));
#52559=CARTESIAN_POINT('Ctrl Pts',(12.5880795783847,-33.6301484067549,-2.56957267415257));
#52560=CARTESIAN_POINT('Ctrl Pts',(12.5880795783847,-29.953804607069,-11.8569743687062));
#52561=CARTESIAN_POINT('Ctrl Pts',(11.6370973936883,-30.6429141327405,-12.1297528718146));
#52562=CARTESIAN_POINT('Ctrl Pts',(11.6370973936883,-24.2547731018213,-28.2678604777126));
#52563=CARTESIAN_POINT('Ctrl Pts',(11.6370973936883,-7.33347131998335,-32.1300371876035));
#52564=CARTESIAN_POINT('Ctrl Pts',(11.6370973936883,24.7965658676201,-39.4635085075869));
#52565=CARTESIAN_POINT('Ctrl Pts',(11.6370973936883,32.1300371876035,-7.33347131998335));
#52566=CARTESIAN_POINT('Ctrl Pts',(11.6370973936883,39.4635085075869,24.7965658676201));
#52567=CARTESIAN_POINT('Ctrl Pts',(11.6370973936883,7.33347131998335,32.1300371876035));
#52568=CARTESIAN_POINT('Ctrl Pts',(11.6370973936883,-24.7965658676201,39.4635085075869));
#52569=CARTESIAN_POINT('Ctrl Pts',(11.6370973936883,-32.1300371876035,7.33347131998335));
#52570=CARTESIAN_POINT('Ctrl Pts',(11.6370973936883,-34.403834952449,-2.62868760228581));
#52571=CARTESIAN_POINT('Ctrl Pts',(11.6370973936883,-30.6429141327405,-12.1297528718146));
#52572=CARTESIAN_POINT('Ctrl Pts',(10.7155646400367,-31.3665139069702,-12.4161840644057));
#52573=CARTESIAN_POINT('Ctrl Pts',(10.7155646400367,-24.8275237307087,-28.9353758899551));
#52574=CARTESIAN_POINT('Ctrl Pts',(10.7155646400367,-7.50664343306871,-32.8887537885844));
#52575=CARTESIAN_POINT('Ctrl Pts',(10.7155646400367,25.3821103555157,-40.3953972216531));
#52576=CARTESIAN_POINT('Ctrl Pts',(10.7155646400367,32.8887537885844,-7.50664343306871));
#52577=CARTESIAN_POINT('Ctrl Pts',(10.7155646400367,40.3953972216531,25.3821103555157));
#52578=CARTESIAN_POINT('Ctrl Pts',(10.7155646400367,7.50664343306871,32.8887537885844));
#52579=CARTESIAN_POINT('Ctrl Pts',(10.7155646400367,-25.3821103555157,40.3953972216531));
#52580=CARTESIAN_POINT('Ctrl Pts',(10.7155646400367,-32.8887537885844,7.50664343306871));
#52581=CARTESIAN_POINT('Ctrl Pts',(10.7155646400367,-35.2162448654354,-2.6907612597485));
#52582=CARTESIAN_POINT('Ctrl Pts',(10.7155646400367,-31.3665139069702,-12.4161840644057));
#52583=CARTESIAN_POINT('Ctrl Pts',(9.82859575068344,-32.1205853335902,-12.7146772172754));
#52584=CARTESIAN_POINT('Ctrl Pts',(9.82859575068344,-25.424393573962,-29.6310011749912));
#52585=CARTESIAN_POINT('Ctrl Pts',(9.82859575068344,-7.68710803106293,-33.6794208535527));
#52586=CARTESIAN_POINT('Ctrl Pts',(9.82859575068344,25.9923128224897,-41.3665288846156));
#52587=CARTESIAN_POINT('Ctrl Pts',(9.82859575068344,33.6794208535527,-7.68710803106293));
#52588=CARTESIAN_POINT('Ctrl Pts',(9.82859575068344,41.3665288846156,25.9923128224897));
#52589=CARTESIAN_POINT('Ctrl Pts',(9.82859575068344,7.68710803106293,33.6794208535527));
#52590=CARTESIAN_POINT('Ctrl Pts',(9.82859575068344,-25.9923128224897,41.3665288846156));
#52591=CARTESIAN_POINT('Ctrl Pts',(9.82859575068344,-33.6794208535527,7.68710803106293));
#52592=CARTESIAN_POINT('Ctrl Pts',(9.82859575068344,-36.0628663320299,-2.75544891320754));
#52593=CARTESIAN_POINT('Ctrl Pts',(9.82859575068344,-32.1205853335902,-12.7146772172754));
#52594=CARTESIAN_POINT('Ctrl Pts',(8.97989469943246,-32.9016913885774,-13.0238718119093));
#52595=CARTESIAN_POINT('Ctrl Pts',(8.97989469943246,-26.0426621253832,-30.3515657037115));
#52596=CARTESIAN_POINT('Ctrl Pts',(8.97989469943246,-7.87404256435505,-34.4984345571934));
#52597=CARTESIAN_POINT('Ctrl Pts',(8.97989469943246,26.6243919928384,-42.3724771215485));
#52598=CARTESIAN_POINT('Ctrl Pts',(8.97989469943246,34.4984345571934,-7.87404256435505));
#52599=CARTESIAN_POINT('Ctrl Pts',(8.97989469943246,42.3724771215485,26.6243919928384));
#52600=CARTESIAN_POINT('Ctrl Pts',(8.97989469943246,7.87404256435505,34.4984345571934));
#52601=CARTESIAN_POINT('Ctrl Pts',(8.97989469943246,-26.6243919928384,42.3724771215485));
#52602=CARTESIAN_POINT('Ctrl Pts',(8.97989469943246,-34.4984345571934,7.87404256435505));
#52603=CARTESIAN_POINT('Ctrl Pts',(8.97989469943246,-36.9398404892439,-2.82245571921564));
#52604=CARTESIAN_POINT('Ctrl Pts',(8.97989469943246,-32.9016913885774,-13.0238718119093));
#52605=CARTESIAN_POINT('Ctrl Pts',(8.1713316609345,-33.707318001253,-13.3427726735042));
#52606=CARTESIAN_POINT('Ctrl Pts',(8.1713316609345,-26.6803394236516,-31.0947502646053));
#52607=CARTESIAN_POINT('Ctrl Pts',(8.1713316609345,-8.06684536480278,-35.3431588191374));
#52608=CARTESIAN_POINT('Ctrl Pts',(8.1713316609345,27.2763134543346,-43.4100041839401));
#52609=CARTESIAN_POINT('Ctrl Pts',(8.1713316609345,35.3431588191374,-8.06684536480278));
#52610=CARTESIAN_POINT('Ctrl Pts',(8.1713316609345,43.4100041839401,27.2763134543346));
#52611=CARTESIAN_POINT('Ctrl Pts',(8.1713316609345,8.06684536480278,35.3431588191374));
#52612=CARTESIAN_POINT('Ctrl Pts',(8.1713316609345,-27.2763134543346,43.4100041839401));
#52613=CARTESIAN_POINT('Ctrl Pts',(8.1713316609345,-35.3431588191374,8.06684536480278));
#52614=CARTESIAN_POINT('Ctrl Pts',(8.1713316609345,-37.8443447049894,-2.89156600943276));
#52615=CARTESIAN_POINT('Ctrl Pts',(8.1713316609345,-33.707318001253,-13.3427726735042));
#52616=CARTESIAN_POINT('Ctrl Pts',(7.40358438374929,-34.5357194373629,-13.6706887670958));
#52617=CARTESIAN_POINT('Ctrl Pts',(7.40358438374929,-27.3360436684578,-31.8589444308015));
#52618=CARTESIAN_POINT('Ctrl Pts',(7.40358438374929,-8.26509864276548,-36.2117631833691));
#52619=CARTESIAN_POINT('Ctrl Pts',(7.40358438374929,27.9466645406036,-44.4768618261345));
#52620=CARTESIAN_POINT('Ctrl Pts',(7.40358438374929,36.2117631833691,-8.26509864276548));
#52621=CARTESIAN_POINT('Ctrl Pts',(7.40358438374929,44.4768618261345,27.9466645406036));
#52622=CARTESIAN_POINT('Ctrl Pts',(7.40358438374929,8.26509864276548,36.2117631833691));
#52623=CARTESIAN_POINT('Ctrl Pts',(7.40358438374929,-27.9466645406036,44.4768618261345));
#52624=CARTESIAN_POINT('Ctrl Pts',(7.40358438374929,-36.2117631833691,8.26509864276548));
#52625=CARTESIAN_POINT('Ctrl Pts',(7.40358438374929,-38.7744189844407,-2.9626300268883));
#52626=CARTESIAN_POINT('Ctrl Pts',(7.40358438374929,-34.5357194373629,-13.6706887670958));
#52627=CARTESIAN_POINT('Ctrl Pts',(6.82198164612729,-35.215801161671,-13.9398936871227));
#52628=CARTESIAN_POINT('Ctrl Pts',(6.82198164612729,-27.8743484733577,-32.4863147655192));
#52629=CARTESIAN_POINT('Ctrl Pts',(6.82198164612729,-8.42785600320626,-36.9248497716085));
#52630=CARTESIAN_POINT('Ctrl Pts',(6.82198164612729,28.4969937684022,-45.3527057748147));
#52631=CARTESIAN_POINT('Ctrl Pts',(6.82198164612729,36.9248497716085,-8.42785600320626));
#52632=CARTESIAN_POINT('Ctrl Pts',(6.82198164612729,45.3527057748147,28.4969937684022));
#52633=CARTESIAN_POINT('Ctrl Pts',(6.82198164612729,8.42785600320626,36.9248497716085));
#52634=CARTESIAN_POINT('Ctrl Pts',(6.82198164612729,-28.4969937684022,45.3527057748147));
#52635=CARTESIAN_POINT('Ctrl Pts',(6.82198164612729,-36.9248497716085,8.42785600320626));
#52636=CARTESIAN_POINT('Ctrl Pts',(6.82198164612729,-39.5379697125444,-3.02097050943789));
#52637=CARTESIAN_POINT('Ctrl Pts',(6.82198164612729,-35.215801161671,-13.9398936871227));
#52638=CARTESIAN_POINT('Ctrl Pts',(6.40395249919757,-35.7353867802651,-14.1455675052848));
#52639=CARTESIAN_POINT('Ctrl Pts',(6.40395249919757,-28.285615862333,-32.9656286358978));
#52640=CARTESIAN_POINT('Ctrl Pts',(6.40395249919757,-8.55220338791416,-37.4696512606331));
#52641=CARTESIAN_POINT('Ctrl Pts',(6.40395249919757,28.9174478727189,-46.0218546485472));
#52642=CARTESIAN_POINT('Ctrl Pts',(6.40395249919757,37.4696512606331,-8.55220338791416));
#52643=CARTESIAN_POINT('Ctrl Pts',(6.40395249919757,46.0218546485472,28.9174478727189));
#52644=CARTESIAN_POINT('Ctrl Pts',(6.40395249919757,8.55220338791416,37.4696512606331));
#52645=CARTESIAN_POINT('Ctrl Pts',(6.40395249919757,-28.9174478727189,46.0218546485472));
#52646=CARTESIAN_POINT('Ctrl Pts',(6.40395249919757,-37.4696512606331,8.55220338791416));
#52647=CARTESIAN_POINT('Ctrl Pts',(6.40395249919757,-40.1213260404818,-3.06554291100543));
#52648=CARTESIAN_POINT('Ctrl Pts',(6.40395249919757,-35.7353867802651,-14.1455675052848));
#52649=CARTESIAN_POINT('Ctrl Pts',(6.13331019225912,-36.0859930662305,-14.2843522039477));
#52650=CARTESIAN_POINT('Ctrl Pts',(6.13331019225912,-28.563131110306,-33.2890603281757));
#52651=CARTESIAN_POINT('Ctrl Pts',(6.13331019225912,-8.63611058850205,-37.8372727263161));
#52652=CARTESIAN_POINT('Ctrl Pts',(6.13331019225912,29.201162137814,-46.4733833148181));
#52653=CARTESIAN_POINT('Ctrl Pts',(6.13331019225912,37.8372727263161,-8.63611058850205));
#52654=CARTESIAN_POINT('Ctrl Pts',(6.13331019225912,46.4733833148181,29.201162137814));
#52655=CARTESIAN_POINT('Ctrl Pts',(6.13331019225912,8.63611058850205,37.8372727263161));
#52656=CARTESIAN_POINT('Ctrl Pts',(6.13331019225912,-29.201162137814,46.4733833148181));
#52657=CARTESIAN_POINT('Ctrl Pts',(6.13331019225912,-37.8372727263161,8.63611058850205));
#52658=CARTESIAN_POINT('Ctrl Pts',(6.13331019225912,-40.5149635627942,-3.09561950206359));
#52659=CARTESIAN_POINT('Ctrl Pts',(6.13331019225912,-36.0859930662305,-14.2843522039477));
#52660=CARTESIAN_POINT('Ctrl Pts',(6.,-36.2623501753963,-14.3541617573767));
#52661=CARTESIAN_POINT('Ctrl Pts',(6.,-28.7027229797079,-33.4517484502831));
#52662=CARTESIAN_POINT('Ctrl Pts',(6.,-8.67831642429627,-38.0221885750911));
#52663=CARTESIAN_POINT('Ctrl Pts',(6.,29.3438721507948,-46.7005049993874));
#52664=CARTESIAN_POINT('Ctrl Pts',(6.,38.0221885750911,-8.67831642429627));
#52665=CARTESIAN_POINT('Ctrl Pts',(6.,46.7005049993874,29.3438721507948));
#52666=CARTESIAN_POINT('Ctrl Pts',(6.,8.67831642429627,38.0221885750911));
#52667=CARTESIAN_POINT('Ctrl Pts',(6.,-29.3438721507948,46.7005049993874));
#52668=CARTESIAN_POINT('Ctrl Pts',(6.,-38.0221885750911,8.67831642429627));
#52669=CARTESIAN_POINT('Ctrl Pts',(6.,-40.712965647392,-3.11074821157311));
#52670=CARTESIAN_POINT('Ctrl Pts',(6.,-36.2623501753963,-14.3541617573767));
#52671=CARTESIAN_POINT('Ctrl Pts',(24.5,-25.1047038636482,-9.93749686382478));
#52672=CARTESIAN_POINT('Ctrl Pts',(23.5178991898112,-24.1800618375919,-12.7285921692414));
#52673=CARTESIAN_POINT('Ctrl Pts',(22.3947886245986,-22.9066712578981,-15.3368782056101));
#52674=CARTESIAN_POINT('Ctrl Pts',(21.1743874927566,-21.4014661870157,-17.7488090012037));
#52675=CARTESIAN_POINT('Ctrl Pts',(20.5031871793432,-20.5736284466467,-19.0753308010405));
#52676=CARTESIAN_POINT('Ctrl Pts',(19.8411792966404,-19.6547951629279,-20.3436164685197));
#52677=CARTESIAN_POINT('Ctrl Pts',(19.1295827650255,-18.6997631766802,-21.5506695935102));
#52678=CARTESIAN_POINT('Ctrl Pts',(18.8261415870909,-18.292515504724,-22.0653848932679));
#52679=CARTESIAN_POINT('Ctrl Pts',(18.5104994276269,-17.8755457477642,-22.5733182213923));
#52680=CARTESIAN_POINT('Ctrl Pts',(18.2016639423759,-17.4841653683043,-23.0425019325362));
#52681=CARTESIAN_POINT('Ctrl Pts',(17.6747132403632,-16.8163723990388,-23.8430468756124));
#52682=CARTESIAN_POINT('Ctrl Pts',(17.2016343370993,-16.1924367304962,-24.5348117442123));
#52683=CARTESIAN_POINT('Ctrl Pts',(16.8729352926459,-15.7719583526041,-24.9977071274998));
#52684=CARTESIAN_POINT('Ctrl Pts',(16.6342454025477,-15.4666214813799,-25.3338457626079));
#52685=CARTESIAN_POINT('Ctrl Pts',(16.5014949770664,-15.3003859066593,-25.5143555186366));
#52686=CARTESIAN_POINT('Ctrl Pts',(16.3424569562979,-15.103934966335,-25.7283911089022));
#52687=CARTESIAN_POINT('Ctrl Pts',(15.993118510103,-14.6724163526426,-26.1985356703879));
#52688=CARTESIAN_POINT('Ctrl Pts',(15.6312480487537,-14.2444422357772,-26.6631523446855));
#52689=CARTESIAN_POINT('Ctrl Pts',(15.2503296894305,-13.8328224068278,-27.1265358149189));
#52690=CARTESIAN_POINT('Ctrl Pts',(14.7484414179076,-13.2904826654642,-27.737078003909));
#52691=CARTESIAN_POINT('Ctrl Pts',(14.2669345517206,-12.758775135315,-28.3184397273517));
#52692=CARTESIAN_POINT('Ctrl Pts',(13.7912435751455,-12.2785123659471,-28.871658502194));
#52693=CARTESIAN_POINT('Ctrl Pts',(13.5533980868579,-12.0383809812632,-29.1482678896151));
#52694=CARTESIAN_POINT('Ctrl Pts',(13.3161115657262,-11.8096746112359,-29.419343552208));
#52695=CARTESIAN_POINT('Ctrl Pts',(13.0766514227367,-11.5950868162136,-29.6877400273009));
#52696=CARTESIAN_POINT('Ctrl Pts',(12.9188702359555,-11.4536941128406,-29.8645874718875));
#52697=CARTESIAN_POINT('Ctrl Pts',(12.7601526360409,-11.3184278068389,-30.040278209103));
#52698=CARTESIAN_POINT('Ctrl Pts',(12.5997389313808,-11.1901315770832,-30.2157244086246));
#52699=CARTESIAN_POINT('Ctrl Pts',(12.5166971934814,-11.1237161675805,-30.3065480533187));
#52700=CARTESIAN_POINT('Ctrl Pts',(12.4397215765388,-11.06399531631,-30.3902672848899));
#52701=CARTESIAN_POINT('Ctrl Pts',(12.3478597934844,-10.9956710033332,-30.4895250762857));
#52702=CARTESIAN_POINT('Ctrl Pts',(11.9116121727781,-10.6712018064435,-30.960896019601));
#52703=CARTESIAN_POINT('Ctrl Pts',(10.7144663992385,-9.70825252947211,-32.2726748359188));
#52704=CARTESIAN_POINT('Ctrl Pts',(9.56604185022483,-9.37660667840678,-33.5284562887129));
#52705=CARTESIAN_POINT('Ctrl Pts',(9.07284645450859,-9.23418007589791,-34.0677565249154));
#52706=CARTESIAN_POINT('Ctrl Pts',(8.57333454992948,-9.18540482457354,-34.6139675361444));
#52707=CARTESIAN_POINT('Ctrl Pts',(8.00348148263344,-9.19403997702536,-35.280177286954));
#52708=CARTESIAN_POINT('Ctrl Pts',(7.6391942896614,-9.19956012884711,-35.7060619473711));
#52709=CARTESIAN_POINT('Ctrl Pts',(7.24388644384717,-9.23557279050204,-36.1897100386463));
#52710=CARTESIAN_POINT('Ctrl Pts',(6.94254646282512,-9.27355849403497,-36.5754634389434));
#52711=CARTESIAN_POINT('Ctrl Pts',(6.91433564865251,-9.27711463557301,-36.6115768595899));
#52712=CARTESIAN_POINT('Ctrl Pts',(6.88669635040545,-9.28069538863599,-36.6471093116181));
#52713=CARTESIAN_POINT('Ctrl Pts',(6.85962514029878,-9.28428605044135,-36.6820512136157));
#52714=CARTESIAN_POINT('Ctrl Pts',(6.4400006207374,-9.33994406236788,-37.2236774941018));
#52715=CARTESIAN_POINT('Ctrl Pts',(6.15412442492902,-9.43557095884828,-37.615340609517));
#52716=CARTESIAN_POINT('Ctrl Pts',(6.,-9.48407679455225,-37.8292517419395));
#52717=CARTESIAN_POINT('Ctrl Pts',(2.09999999999998,-3.03601716990075,-9.25709704779465));
#52718=CARTESIAN_POINT('Ctrl Pts',(2.73333333333332,-3.03601716990075,-9.25709704779465));
#52719=CARTESIAN_POINT('Ctrl Pts',(3.36700010948328,-3.03596462825959,-9.25711949436599));
#52720=CARTESIAN_POINT('Ctrl Pts',(4.12580403847648,-3.035948752271,-9.25712636633026));
#52721=CARTESIAN_POINT('Ctrl Pts',(4.38276376087194,-3.034724599393,-9.25754213874175));
#52722=CARTESIAN_POINT('Ctrl Pts',(4.88872719354341,-3.02930124281597,-9.25939165981087));
#52723=CARTESIAN_POINT('Ctrl Pts',(5.76577603006097,-3.01680014358279,-9.26367065608843));
#52724=CARTESIAN_POINT('Ctrl Pts',(6.49295950172122,-3.01700281594616,-9.2636387759413));
#52725=CARTESIAN_POINT('Ctrl Pts',(7.02336263943405,-3.03738330196137,-9.25654898425916));
#52726=CARTESIAN_POINT('Ctrl Pts',(7.14974440406645,-3.04241854797673,-9.25486655932582));
#52727=CARTESIAN_POINT('Ctrl Pts',(7.3995736148146,-3.05315049883967,-9.25139226428141));
#52728=CARTESIAN_POINT('Ctrl Pts',(7.71336783445791,-3.06825567663682,-9.24666612381336));
#52729=CARTESIAN_POINT('Ctrl Pts',(8.08762134632205,-3.08956528022687,-9.24001026491592));
#52730=CARTESIAN_POINT('Ctrl Pts',(8.58204140724159,-3.12288355797465,-9.22935038479259));
#52731=CARTESIAN_POINT('Ctrl Pts',(9.18586634302998,-3.17504806239954,-9.21173549473203));
#52732=CARTESIAN_POINT('Ctrl Pts',(9.64253482836406,-3.23031373876087,-9.19124308846978));
#52733=CARTESIAN_POINT('Ctrl Pts',(10.3691868352069,-3.33481918503072,-9.15051861370346));
#52734=CARTESIAN_POINT('Ctrl Pts',(11.1024062533893,-3.4863313251209,-9.09516757635316));
#52735=CARTESIAN_POINT('Ctrl Pts',(12.0425597052338,-3.73241232718711,-8.9976503328513));
#52736=CARTESIAN_POINT('Ctrl Pts',(12.4996009342521,-3.86235209382665,-8.9414277018268));
#52737=CARTESIAN_POINT('Ctrl Pts',(13.0011558990775,-4.00644645143633,-8.874918979412));
#52738=CARTESIAN_POINT('Ctrl Pts',(13.5006112777572,-4.1651105541745,-8.79993648213644));
#52739=CARTESIAN_POINT('Ctrl Pts',(14.4710715650308,-4.52003869162835,-8.62597550507522));
#52740=CARTESIAN_POINT('Ctrl Pts',(15.1518211493114,-4.80485184597868,-8.4717928050839));
#52741=CARTESIAN_POINT('Ctrl Pts',(15.8845703284776,-5.10582280931469,-8.28722797188002));
#52742=CARTESIAN_POINT('Ctrl Pts',(16.3869968088152,-5.32489776769872,-8.14702496307046));
#52743=CARTESIAN_POINT('Ctrl Pts',(17.3639569585992,-5.78783984375356,-7.83062294262033));
#52744=CARTESIAN_POINT('Ctrl Pts',(18.0500309778779,-6.13616822192816,-7.5603268394043));
#52745=CARTESIAN_POINT('Ctrl Pts',(18.7841811416569,-6.49299855871679,-7.24692816530861));
#52746=CARTESIAN_POINT('Ctrl Pts',(19.2877130443133,-6.74580743680106,-7.01244208981508));
#52747=CARTESIAN_POINT('Ctrl Pts',(20.2708116551819,-7.25764700376677,-6.49248945683397));
#52748=CARTESIAN_POINT('Ctrl Pts',(20.9685591537265,-7.61989877001792,-6.05996067164741));
#52749=CARTESIAN_POINT('Ctrl Pts',(22.6570098912121,-8.41829456543365,-4.95637665599812));
#52750=CARTESIAN_POINT('Ctrl Pts',(23.7241254823866,-8.86254721730646,-4.07948871958989));
#52751=CARTESIAN_POINT('Ctrl Pts',(24.6950729185821,-9.21040909328162,-3.09630974804701));
#52752=CARTESIAN_POINT('Ctrl Pts',(2.09999999999998,-3.65672665621579,-11.9766029963153));
#52753=CARTESIAN_POINT('Ctrl Pts',(2.73333333333332,-3.65672665621579,-11.9766029963153));
#52754=CARTESIAN_POINT('Ctrl Pts',(3.36712120601687,-3.65665584340833,-11.9766315438739));
#52755=CARTESIAN_POINT('Ctrl Pts',(4.12606819216906,-3.65663454744001,-11.9766402477875));
#52756=CARTESIAN_POINT('Ctrl Pts',(4.38492925999049,-3.65504218826977,-11.9771449683934));
#52757=CARTESIAN_POINT('Ctrl Pts',(4.89215030047201,-3.64800886033491,-11.9793835290183));
#52758=CARTESIAN_POINT('Ctrl Pts',(5.76872623835731,-3.63183832461054,-11.9845504064978));
#52759=CARTESIAN_POINT('Ctrl Pts',(6.48937126159138,-3.63217364414716,-11.9844905633463));
#52760=CARTESIAN_POINT('Ctrl Pts',(7.01201831810172,-3.65824051638801,-11.976019521284));
#52761=CARTESIAN_POINT('Ctrl Pts',(7.13827913651891,-3.66474966328796,-11.973992649138));
#52762=CARTESIAN_POINT('Ctrl Pts',(7.38675263276647,-3.67857740242105,-11.9698307262182));
#52763=CARTESIAN_POINT('Ctrl Pts',(7.69894445702103,-3.69804158026563,-11.9641827355297));
#52764=CARTESIAN_POINT('Ctrl Pts',(8.07058283408763,-3.72546787164587,-11.9562412019396));
#52765=CARTESIAN_POINT('Ctrl Pts',(8.5609042839681,-3.76830356997935,-11.9435176419542));
#52766=CARTESIAN_POINT('Ctrl Pts',(9.15816221625486,-3.83525991280854,-11.9224539215507));
#52767=CARTESIAN_POINT('Ctrl Pts',(9.60779259539962,-3.90596474603746,-11.8978913861869));
#52768=CARTESIAN_POINT('Ctrl Pts',(10.3209229382447,-4.0393084045542,-11.8490818060896));
#52769=CARTESIAN_POINT('Ctrl Pts',(11.0425587715381,-4.23303562018289,-11.7830103781896));
#52770=CARTESIAN_POINT('Ctrl Pts',(11.9743044133905,-4.5497935018951,-11.6653836085843));
#52771=CARTESIAN_POINT('Ctrl Pts',(12.4288874618463,-4.71763528480831,-11.5970273246365));
#52772=CARTESIAN_POINT('Ctrl Pts',(12.9286787374574,-4.90408555889076,-11.5157778410948));
#52773=CARTESIAN_POINT('Ctrl Pts',(13.4199974526641,-5.10750718068235,-11.4251100220548));
#52774=CARTESIAN_POINT('Ctrl Pts',(14.3833031177915,-5.5657285644765,-11.2131707854604));
#52775=CARTESIAN_POINT('Ctrl Pts',(15.0609019352795,-5.93504727306437,-11.0239005734077));
#52776=CARTESIAN_POINT('Ctrl Pts',(15.7927804449946,-6.32674632713181,-10.7954801539631));
#52777=CARTESIAN_POINT('Ctrl Pts',(16.2911437356496,-6.61047183230131,-10.6230415607221));
#52778=CARTESIAN_POINT('Ctrl Pts',(17.2659647556227,-7.21340018457687,-10.2311373480415));
#52779=CARTESIAN_POINT('Ctrl Pts',(17.9510657357558,-7.6687887141322,-9.89424383461141));
#52780=CARTESIAN_POINT('Ctrl Pts',(18.6848815503035,-8.13642726571135,-9.50186505396924));
#52781=CARTESIAN_POINT('Ctrl Pts',(19.1880112925449,-8.46802605481274,-9.20863204572925));
#52782=CARTESIAN_POINT('Ctrl Pts',(20.1723367890838,-9.14185982964497,-8.5552931434037));
#52783=CARTESIAN_POINT('Ctrl Pts',(20.8704681776515,-9.62058702907129,-8.00953397034699));
#52784=CARTESIAN_POINT('Ctrl Pts',(22.5588081046095,-10.6788873378614,-6.61393451767592));
#52785=CARTESIAN_POINT('Ctrl Pts',(23.6292145427077,-11.2779081469627,-5.49853642353553));
#52786=CARTESIAN_POINT('Ctrl Pts',(24.6070641578141,-11.7565436874769,-4.23746132912074));
#52787=CARTESIAN_POINT('Ctrl Pts',(2.09999999999998,-4.89814562884588,-17.4156148933567));
#52788=CARTESIAN_POINT('Ctrl Pts',(2.73333333333332,-4.89814562884588,-17.4156148933567));
#52789=CARTESIAN_POINT('Ctrl Pts',(3.36737232571569,-4.89802150608842,-17.4156658916616));
#52790=CARTESIAN_POINT('Ctrl Pts',(4.12660787609934,-4.89798436968063,-17.4156813973428));
#52791=CARTESIAN_POINT('Ctrl Pts',(4.38927320923596,-4.89563957363679,-17.4163681981935));
#52792=CARTESIAN_POINT('Ctrl Pts',(4.89900603841974,-4.88535460251535,-17.4193932655343));
#52793=CARTESIAN_POINT('Ctrl Pts',(5.77465260126722,-4.86184729038438,-17.4263372104577));
#52794=CARTESIAN_POINT('Ctrl Pts',(6.48219688444387,-4.8625594972863,-17.4262048870286));
#52795=CARTESIAN_POINT('Ctrl Pts',(6.98943485738849,-4.89946344728588,-17.4150979412944));
#52796=CARTESIAN_POINT('Ctrl Pts',(7.11545613477531,-4.90891054226745,-17.4123848398668));
#52797=CARTESIAN_POINT('Ctrl Pts',(7.36123936390851,-4.92882868688397,-17.4068717375096));
#52798=CARTESIAN_POINT('Ctrl Pts',(7.6702627990277,-4.95686731223262,-17.3994166487763));
#52799=CARTESIAN_POINT('Ctrl Pts',(8.0367413968953,-4.99627118676861,-17.388965573053));
#52800=CARTESIAN_POINT('Ctrl Pts',(8.51903353084918,-5.05765076313434,-17.3722391830899));
#52801=CARTESIAN_POINT('Ctrl Pts',(9.10355742307647,-5.15323263978595,-17.3445211388576));
#52802=CARTESIAN_POINT('Ctrl Pts',(9.53998094727572,-5.2533971526662,-17.3122002900072));
#52803=CARTESIAN_POINT('Ctrl Pts',(10.2287061596417,-5.44121042790069,-17.248118841033));
#52804=CARTESIAN_POINT('Ctrl Pts',(10.9322684728187,-5.71569213117839,-17.161803418548));
#52805=CARTESIAN_POINT('Ctrl Pts',(11.853432502986,-6.17162681919986,-17.0050023819074));
#52806=CARTESIAN_POINT('Ctrl Pts',(12.3052534899461,-6.41468310776573,-16.9128099061716));
#52807=CARTESIAN_POINT('Ctrl Pts',(12.8031221556086,-6.68546702830436,-16.8024678490713));
#52808=CARTESIAN_POINT('Ctrl Pts',(13.2871761296055,-6.97708915103167,-16.6812571176895));
#52809=CARTESIAN_POINT('Ctrl Pts',(14.2486052139259,-7.64348346076381,-16.3934928083832));
#52810=CARTESIAN_POINT('Ctrl Pts',(14.9265811207677,-8.1832906380615,-16.1339663223503));
#52811=CARTESIAN_POINT('Ctrl Pts',(15.6586876395449,-8.75682074682074,-15.8182194362082));
#52812=CARTESIAN_POINT('Ctrl Pts',(16.1598454115811,-9.17372704265915,-15.5797361779835));
#52813=CARTESIAN_POINT('Ctrl Pts',(17.1407792334809,-10.0631541608939,-15.0333575221981));
#52814=CARTESIAN_POINT('Ctrl Pts',(17.8296148723165,-10.7357158426118,-14.5611645715286));
#52815=CARTESIAN_POINT('Ctrl Pts',(18.5645831613832,-11.4254945580397,-14.0102872287392));
#52816=CARTESIAN_POINT('Ctrl Pts',(19.0747832425015,-11.9208360855031,-13.594485353105));
#52817=CARTESIAN_POINT('Ctrl Pts',(20.0668692671653,-12.924375055063,-12.6673387976086));
#52818=CARTESIAN_POINT('Ctrl Pts',(20.7688147271569,-13.6377206973786,-11.8912879181046));
#52819=CARTESIAN_POINT('Ctrl Pts',(22.460121536001,-15.2149112429765,-9.90766328280056));
#52820=CARTESIAN_POINT('Ctrl Pts',(23.5475247071985,-16.1319458054889,-8.29734249637728));
#52821=CARTESIAN_POINT('Ctrl Pts',(24.5367270315052,-16.8702662262976,-6.46720007277371));
#52822=CARTESIAN_POINT('Ctrl Pts',(2.09999999999998,-7.07062883094854,-26.9338857131792));
#52823=CARTESIAN_POINT('Ctrl Pts',(2.73333333333332,-7.07062883094854,-26.9338857131792));
#52824=CARTESIAN_POINT('Ctrl Pts',(3.36789866008651,-7.07046463114355,-26.933951186598));
#52825=CARTESIAN_POINT('Ctrl Pts',(4.12766416179872,-7.07041695394235,-26.9339707016016));
#52826=CARTESIAN_POINT('Ctrl Pts',(4.39699933335947,-7.0667088058488,-26.934985849138));
#52827=CARTESIAN_POINT('Ctrl Pts',(4.91111167246882,-7.05064293531159,-26.9394051279664));
#52828=CARTESIAN_POINT('Ctrl Pts',(5.78524431219031,-7.01434026039855,-26.9494462503479));
#52829=CARTESIAN_POINT('Ctrl Pts',(6.46975410539064,-7.01623847673174,-26.9490470248394));
#52830=CARTESIAN_POINT('Ctrl Pts',(6.95069999511141,-7.07036165458142,-26.93372166352));
#52831=CARTESIAN_POINT('Ctrl Pts',(7.0763178603825,-7.08492048653749,-26.9298148743264));
#52832=CARTESIAN_POINT('Ctrl Pts',(7.31752917791793,-7.11516421888208,-26.9220146572799));
#52833=CARTESIAN_POINT('Ctrl Pts',(7.62124943258259,-7.15777761960928,-26.9114950065043));
#52834=CARTESIAN_POINT('Ctrl Pts',(7.97914075673115,-7.21732108737006,-26.8968488632838));
#52835=CARTESIAN_POINT('Ctrl Pts',(8.44843546348636,-7.30970068233947,-26.8734648474066));
#52836=CARTESIAN_POINT('Ctrl Pts',(9.01308885010149,-7.45261747655674,-26.834787200002));
#52837=CARTESIAN_POINT('Ctrl Pts',(9.43131294671769,-7.60102319336957,-26.7897594463226));
#52838=CARTESIAN_POINT('Ctrl Pts',(10.0907596971815,-7.87860422770284,-26.7004946164726));
#52839=CARTESIAN_POINT('Ctrl Pts',(10.783467320144,-8.29417685100599,-26.5791525451474));
#52840=CARTESIAN_POINT('Ctrl Pts',(11.7034138999861,-8.99870155634605,-26.3527123769869));
#52841=CARTESIAN_POINT('Ctrl Pts',(12.1558320275245,-9.37558967844092,-26.2182079026623));
#52842=CARTESIAN_POINT('Ctrl Pts',(12.6542336070705,-9.7957041418195,-26.0565093323377));
#52843=CARTESIAN_POINT('Ctrl Pts',(13.1437514887892,-10.2520206694373,-25.8782496367525));
#52844=CARTESIAN_POINT('Ctrl Pts',(14.1171197855423,-11.298685793984,-25.4510876928653));
#52845=CARTESIAN_POINT('Ctrl Pts',(14.801673515149,-12.1453574316379,-25.0635325427391));
#52846=CARTESIAN_POINT('Ctrl Pts',(15.5357864365759,-13.0393873617087,-24.5925527412693));
#52847=CARTESIAN_POINT('Ctrl Pts',(16.048368284242,-13.7028332567132,-24.2302701739799));
#52848=CARTESIAN_POINT('Ctrl Pts',(17.0412321177376,-15.1050304906995,-23.4030485209266));
#52849=CARTESIAN_POINT('Ctrl Pts',(17.7361726306612,-16.1624249607158,-22.6867927333657));
#52850=CARTESIAN_POINT('Ctrl Pts',(18.4727161996985,-17.2407120307395,-21.854310708133));
#52851=CARTESIAN_POINT('Ctrl Pts',(18.992653507987,-18.0297266688986,-21.2147361058502));
#52852=CARTESIAN_POINT('Ctrl Pts',(19.993201743462,-19.6118718391751,-19.7977134333265));
#52853=CARTESIAN_POINT('Ctrl Pts',(20.6988514049915,-20.7341708993179,-18.6120452244264));
#52854=CARTESIAN_POINT('Ctrl Pts',(22.392495758694,-23.2107201272583,-15.588579749096));
#52855=CARTESIAN_POINT('Ctrl Pts',(23.493455201073,-24.679434474049,-13.0976556158903));
#52856=CARTESIAN_POINT('Ctrl Pts',(24.4910959878399,-25.8615426952525,-10.2656936020237));
#52857=CARTESIAN_POINT('Ctrl Pts',(2.09999999999998,-8.62240254673614,-33.7326505844809));
#52858=CARTESIAN_POINT('Ctrl Pts',(2.73333333333332,-8.62240254673614,-33.7326505844809));
#52859=CARTESIAN_POINT('Ctrl Pts',(3.36827652301208,-8.62225231332109,-33.7327142066686));
#52860=CARTESIAN_POINT('Ctrl Pts',(4.12841844272612,-8.62221062515808,-33.7327327108703));
#52861=CARTESIAN_POINT('Ctrl Pts',(4.40252493993054,-8.61748756225129,-33.7339916386456));
#52862=CARTESIAN_POINT('Ctrl Pts',(4.91972290753806,-8.59720819332077,-33.7394252545322));
#52863=CARTESIAN_POINT('Ctrl Pts',(5.79289024162273,-8.55181496845626,-33.7516673236045));
#52864=CARTESIAN_POINT('Ctrl Pts',(6.46065121315474,-8.55498795191946,-33.7509749771614));
#52865=CARTESIAN_POINT('Ctrl Pts',(6.92361646112076,-8.61993893328495,-33.7329735018433));
#52866=CARTESIAN_POINT('Ctrl Pts',(7.04896306476174,-8.63812452107151,-33.7282202863535));
#52867=CARTESIAN_POINT('Ctrl Pts',(7.28707567322587,-8.6754667244593,-33.7188513918404));
#52868=CARTESIAN_POINT('Ctrl Pts',(7.58726936452363,-8.72814137561322,-33.7062253222916));
#52869=CARTESIAN_POINT('Ctrl Pts',(7.93957047450264,-8.80142249811336,-33.6887386990264));
#52870=CARTESIAN_POINT('Ctrl Pts',(8.4007825112503,-8.91487937592376,-33.6608602352034));
#52871=CARTESIAN_POINT('Ctrl Pts',(8.95401946717244,-9.0897746461696,-33.6148182100539));
#52872=CARTESIAN_POINT('Ctrl Pts',(9.36430401987977,-9.27132051394991,-33.5610861019821));
#52873=CARTESIAN_POINT('Ctrl Pts',(10.0148540524883,-9.61284682840088,-33.4539650268594));
#52874=CARTESIAN_POINT('Ctrl Pts',(10.7127161292919,-10.1356319642981,-33.3060111863704));
#52875=CARTESIAN_POINT('Ctrl Pts',(11.6387106704067,-11.0248489283853,-33.027535101029));
#52876=CARTESIAN_POINT('Ctrl Pts',(12.0933528256764,-11.499599242688,-32.8619317339318));
#52877=CARTESIAN_POINT('Ctrl Pts',(12.5933109512149,-12.0280110081881,-32.6628317330708));
#52878=CARTESIAN_POINT('Ctrl Pts',(13.0908899144144,-12.6103513701059,-32.4405637422004));
#52879=CARTESIAN_POINT('Ctrl Pts',(14.0727400062371,-13.9365257971833,-31.9095619676101));
#52880=CARTESIAN_POINT('Ctrl Pts',(14.7612410141007,-15.0052037777513,-31.428066405722));
#52881=CARTESIAN_POINT('Ctrl Pts',(15.4964903549183,-16.1284628018935,-30.8447244672));
#52882=CARTESIAN_POINT('Ctrl Pts',(16.0148660701553,-16.9719590519182,-30.3908356683825));
#52883=CARTESIAN_POINT('Ctrl Pts',(17.0124971364499,-18.7417950627702,-29.3593075139289));
#52884=CARTESIAN_POINT('Ctrl Pts',(17.7100001824936,-20.0739603594528,-28.46645334904));
#52885=CARTESIAN_POINT('Ctrl Pts',(18.4472556019989,-21.4286595752151,-27.4310110272601));
#52886=CARTESIAN_POINT('Ctrl Pts',(18.970741165076,-22.4274147758341,-26.6295389239519));
#52887=CARTESIAN_POINT('Ctrl Pts',(19.9740132395736,-24.4205958470129,-24.8598580553113));
#52888=CARTESIAN_POINT('Ctrl Pts',(20.6810428764808,-25.8331306408346,-23.3798043172822));
#52889=CARTESIAN_POINT('Ctrl Pts',(22.3757637844863,-28.9472763223035,-19.6095668360326));
#52890=CARTESIAN_POINT('Ctrl Pts',(23.4815899075194,-30.8056241230732,-16.4879028202221));
#52891=CARTESIAN_POINT('Ctrl Pts',(24.4815088739376,-32.299518402771,-12.9405938991905));
#52892=CARTESIAN_POINT('Ctrl Pts',(2.09999999999998,-9.55346677620871,-37.8119095072619));
#52893=CARTESIAN_POINT('Ctrl Pts',(2.73333333333332,-9.55346677620871,-37.8119095072619));
#52894=CARTESIAN_POINT('Ctrl Pts',(3.36850564609381,-9.55333227030529,-37.8119692060198));
#52895=CARTESIAN_POINT('Ctrl Pts',(4.12887280195021,-9.55329634226044,-37.8119862483609));
#52896=CARTESIAN_POINT('Ctrl Pts',(4.40584576278457,-9.54794955963462,-37.8133947479414));
#52897=CARTESIAN_POINT('Ctrl Pts',(4.92487357234802,-9.5251083652532,-37.8194443413709));
#52898=CARTESIAN_POINT('Ctrl Pts',(5.79752076681712,-9.47428442849641,-37.833001467378));
#52899=CARTESIAN_POINT('Ctrl Pts',(6.45508636861402,-9.47833876217847,-37.8321045685465));
#52900=CARTESIAN_POINT('Ctrl Pts',(6.9076663195535,-9.54931802126756,-37.8126045589407));
#52901=CARTESIAN_POINT('Ctrl Pts',(7.03285856585593,-9.56967214728074,-37.8073454003161));
#52902=CARTESIAN_POINT('Ctrl Pts',(7.2691953296767,-9.61118811110219,-37.7970553432032));
#52903=CARTESIAN_POINT('Ctrl Pts',(7.56740105178408,-9.66979660166033,-37.7831896546061));
#52904=CARTESIAN_POINT('Ctrl Pts',(7.91660842131089,-9.75114654641155,-37.7640408695922));
#52905=CARTESIAN_POINT('Ctrl Pts',(8.37351535097609,-9.87701212539291,-37.7335242639715));
#52906=CARTESIAN_POINT('Ctrl Pts',(8.92109193346782,-10.070823088101,-37.6831357925027));
#52907=CARTESIAN_POINT('Ctrl Pts',(9.3283399907512,-10.2725679422737,-37.6241111672603));
#52908=CARTESIAN_POINT('Ctrl Pts',(9.97668494845576,-10.6540371711336,-37.5058782148325));
#52909=CARTESIAN_POINT('Ctrl Pts',(10.6788554165274,-11.2439508033002,-37.3411579803345));
#52910=CARTESIAN_POINT('Ctrl Pts',(11.6082441119523,-12.2454537985995,-37.030864103448));
#52911=CARTESIAN_POINT('Ctrl Pts',(12.0641366410534,-12.7793441548631,-36.8463749959916));
#52912=CARTESIAN_POINT('Ctrl Pts',(12.5649391142128,-13.3729973335818,-36.6246423121547));
#52913=CARTESIAN_POINT('Ctrl Pts',(13.0665672847697,-14.0319733807286,-36.3754643696926));
#52914=CARTESIAN_POINT('Ctrl Pts',(14.052339822417,-15.5260272045887,-35.7817417873778));
#52915=CARTESIAN_POINT('Ctrl Pts',(14.7427747351421,-16.7279921888766,-35.2435532673183));
#52916=CARTESIAN_POINT('Ctrl Pts',(15.478585307449,-17.9887566041688,-34.5924957389832));
#52917=CARTESIAN_POINT('Ctrl Pts',(15.9996615571876,-18.9401568844199,-34.0834579338314));
#52918=CARTESIAN_POINT('Ctrl Pts',(16.9995120437242,-20.9301248352716,-32.9291013640743));
#52919=CARTESIAN_POINT('Ctrl Pts',(17.6981753134392,-22.4269478260738,-31.9300105678004));
#52920=CARTESIAN_POINT('Ctrl Pts',(18.4357263982027,-23.9473093246625,-30.7724847771855));
#52921=CARTESIAN_POINT('Ctrl Pts',(18.9608339174453,-25.0715521287826,-29.8738096356868));
#52922=CARTESIAN_POINT('Ctrl Pts',(19.9653539792613,-27.310810104301,-27.8923455557466));
#52923=CARTESIAN_POINT('Ctrl Pts',(20.6729500616029,-28.8971249702565,-26.2354633096799));
#52924=CARTESIAN_POINT('Ctrl Pts',(22.3680345174968,-32.3930758837889,-22.016595619137));
#52925=CARTESIAN_POINT('Ctrl Pts',(23.4757593035169,-34.4841356290003,-18.5166596137722));
#52926=CARTESIAN_POINT('Ctrl Pts',(24.4767076204831,-36.1644175597347,-14.5403550674526));
#52927=CARTESIAN_POINT('',(3.2,-9.24182505978395,-36.4465179346992));
#52928=CARTESIAN_POINT('Ctrl Pts',(3.2,-9.24182505978396,-36.4465179346992));
#52929=CARTESIAN_POINT('Ctrl Pts',(3.45174020132946,-9.06882103761919,-35.6885377881604));
#52930=CARTESIAN_POINT('Ctrl Pts',(3.71840125362201,-8.8937755557219,-34.9216134221298));
#52931=CARTESIAN_POINT('Ctrl Pts',(4.,-8.71775829923915,-34.1504314334527));
#52932=CARTESIAN_POINT('Ctrl Pts',(4.62816481100596,-8.32511505038087,-32.4301489591897));
#52933=CARTESIAN_POINT('Ctrl Pts',(5.3258296688808,-7.87421940038907,-30.7255530003983));
#52934=CARTESIAN_POINT('Ctrl Pts',(6.03866107788435,-7.51769424249301,-29.1403169479585));
#52935=CARTESIAN_POINT('Ctrl Pts',(6.32798217848354,-7.37298926769682,-28.4969078141739));
#52936=CARTESIAN_POINT('Ctrl Pts',(6.61604116639212,-7.24664165658202,-27.8802695301434));
#52937=CARTESIAN_POINT('Ctrl Pts',(6.89476148100327,-7.14787574329671,-27.300072414889));
#52938=CARTESIAN_POINT('Ctrl Pts',(7.65522892931241,-6.87840036558412,-25.7170481549983));
#52939=CARTESIAN_POINT('Ctrl Pts',(8.35226709412095,-6.70318404327883,-24.4283041728914));
#52940=CARTESIAN_POINT('Ctrl Pts',(8.78926323759003,-6.62195963494359,-23.6418688208757));
#52941=CARTESIAN_POINT('Ctrl Pts',(8.99031957655721,-6.58458932305704,-23.2800399693545));
#52942=CARTESIAN_POINT('Ctrl Pts',(9.18275521872759,-6.55559338009954,-22.9406688489254));
#52943=CARTESIAN_POINT('Ctrl Pts',(9.37496045616592,-6.53433836529711,-22.6068036124997));
#52944=CARTESIAN_POINT('Ctrl Pts',(9.48075232992955,-6.52263937169636,-22.4230405193771));
#52945=CARTESIAN_POINT('Ctrl Pts',(9.5862609074853,-6.51335864091999,-22.2413624031642));
#52946=CARTESIAN_POINT('Ctrl Pts',(9.69257910363365,-6.50683293166549,-22.0596557590578));
#52947=CARTESIAN_POINT('Ctrl Pts',(10.0319880466963,-6.48600033516701,-21.4795776326612));
#52948=CARTESIAN_POINT('Ctrl Pts',(10.3788056739135,-6.49425759660125,-20.8988170113787));
#52949=CARTESIAN_POINT('Ctrl Pts',(10.7756849082151,-6.52753448251735,-20.2533506733983));
#52950=CARTESIAN_POINT('Ctrl Pts',(10.8890930402954,-6.53704334351844,-20.0689088447904));
#52951=CARTESIAN_POINT('Ctrl Pts',(11.0576203521665,-6.55312978036577,-19.7960739175289));
#52952=CARTESIAN_POINT('Ctrl Pts',(11.2725125494692,-6.57904145901406,-19.4548645888988));
#52953=CARTESIAN_POINT('Ctrl Pts',(11.5968279594503,-6.61814737718885,-18.9399113021204));
#52954=CARTESIAN_POINT('Ctrl Pts',(12.025567884427,-6.6827471737312,-18.2703586753637));
#52955=CARTESIAN_POINT('Ctrl Pts',(12.532035905153,-6.75393793425464,-17.5203993948461));
#52956=CARTESIAN_POINT('Ctrl Pts',(13.0988763177885,-6.83361483076056,-16.6810428893375));
#52957=CARTESIAN_POINT('Ctrl Pts',(13.7495416920733,-6.97877204198315,-15.7393500659831));
#52958=CARTESIAN_POINT('Ctrl Pts',(14.4398764944186,-7.14095491661005,-14.7876869742977));
#52959=CARTESIAN_POINT('Ctrl Pts',(14.7901814040927,-7.2232533275461,-14.3047731008548));
#52960=CARTESIAN_POINT('Ctrl Pts',(15.1459546154366,-7.30586903884694,-13.8278491968692));
#52961=CARTESIAN_POINT('Ctrl Pts',(15.4570717747561,-7.37026799935016,-13.4241590170948));
#52962=CARTESIAN_POINT('Ctrl Pts',(15.7998231401197,-7.44121500750863,-12.9794218621136));
#52963=CARTESIAN_POINT('Ctrl Pts',(16.0676294483849,-7.50355110660171,-12.637469237209));
#52964=CARTESIAN_POINT('Ctrl Pts',(16.3615307957941,-7.57387201213481,-12.2669409047598));
#52965=CARTESIAN_POINT('Ctrl Pts',(17.0296616012911,-7.73373369249551,-11.4246127038138));
#52966=CARTESIAN_POINT('Ctrl Pts',(17.7084691868929,-7.91242588701926,-10.5936031634317));
#52967=CARTESIAN_POINT('Ctrl Pts',(18.4207032016838,-8.06194162094658,-9.78641628469765));
#52968=CARTESIAN_POINT('Ctrl Pts',(18.8298642041889,-8.14783474920716,-9.32270718677038));
#52969=CARTESIAN_POINT('Ctrl Pts',(19.2113759272395,-8.23555418397616,-8.8952152917086));
#52970=CARTESIAN_POINT('Ctrl Pts',(19.5701113607057,-8.31748924110769,-8.49743627926558));
#52971=CARTESIAN_POINT('Ctrl Pts',(20.121547602182,-8.44343710054603,-7.88598353973464));
#52972=CARTESIAN_POINT('Ctrl Pts',(20.6514912601917,-8.57040043767199,-7.29974693210948));
#52973=CARTESIAN_POINT('Ctrl Pts',(21.3979544325339,-8.70094314511465,-6.5286488228905));
#52974=CARTESIAN_POINT('Ctrl Pts',(21.8107631282201,-8.77313580884871,-6.10221652655357));
#52975=CARTESIAN_POINT('Ctrl Pts',(22.3076315955579,-8.85489558536126,-5.5960154347174));
#52976=CARTESIAN_POINT('Ctrl Pts',(22.8472772295406,-8.93355440585529,-5.03999075031881));
#52977=CARTESIAN_POINT('Ctrl Pts',(23.3953136568816,-9.01343626952248,-4.47532059946028));
#52978=CARTESIAN_POINT('Ctrl Pts',(23.9608264583214,-9.08615837741543,-3.88432348473261));
#52979=CARTESIAN_POINT('Ctrl Pts',(24.5,-9.13966689904905,-3.29104195297002));
#52980=CARTESIAN_POINT('Ctrl Pts',(2.7975955995408,-9.45110532887384,-37.363642330079));
#52981=CARTESIAN_POINT('Ctrl Pts',(2.93204421046394,-9.3813783568972,-37.0582190820374));
#52982=CARTESIAN_POINT('Ctrl Pts',(3.06669822891363,-9.31156415154198,-36.7524257548829));
#52983=CARTESIAN_POINT('Ctrl Pts',(3.20140554545437,-9.24173281535836,-36.4465583754197));
#52984=CARTESIAN_POINT('Origin',(2.9,0.,0.));
#52985=CARTESIAN_POINT('Origin',(3.2,0.,0.));
#52986=CARTESIAN_POINT('Ctrl Pts',(2.1,-8.3510594145214,-5.02058289194443));
#52987=CARTESIAN_POINT('Ctrl Pts',(2.73333333333334,-8.3510594145214,-5.02058289194443));
#52988=CARTESIAN_POINT('Ctrl Pts',(3.36630413798689,-8.35107248850531,-5.02053567019918));
#52989=CARTESIAN_POINT('Ctrl Pts',(4.124157833359,-8.35107634006013,-5.0205214484641));
#52990=CARTESIAN_POINT('Ctrl Pts',(4.36790635424917,-8.3504576041077,-5.02157407473443));
#52991=CARTESIAN_POINT('Ctrl Pts',(4.86513593837425,-8.34763711932882,-5.02638994376713));
#52992=CARTESIAN_POINT('Ctrl Pts',(5.74555319889928,-8.3409895121078,-5.03776769314777));
#52993=CARTESIAN_POINT('Ctrl Pts',(6.51831486887852,-8.34088452878131,-5.03795859267391));
#52994=CARTESIAN_POINT('Ctrl Pts',(7.10304244324289,-8.35279167464714,-5.01737867305202));
#52995=CARTESIAN_POINT('Ctrl Pts',(7.23019749510073,-8.35551879167041,-5.01278329615679));
#52996=CARTESIAN_POINT('Ctrl Pts',(7.4248770951455,-8.36007698205955,-5.00525711413222));
#52997=CARTESIAN_POINT('Ctrl Pts',(7.61944598119582,-8.36505833151271,-4.99715327807895));
#52998=CARTESIAN_POINT('Ctrl Pts',(8.0106922175681,-8.37596024104948,-4.97952710685782));
#52999=CARTESIAN_POINT('Ctrl Pts',(8.6007456943798,-8.39597936834588,-4.94716218491378));
#53000=CARTESIAN_POINT('Ctrl Pts',(9.25144198408345,-8.42603538580927,-4.89603670853206));
#53001=CARTESIAN_POINT('Ctrl Pts',(9.7625585744136,-8.45565760052341,-4.84294672360393));
#53002=CARTESIAN_POINT('Ctrl Pts',(10.014053299629,-8.47250040429509,-4.81175577398779));
#53003=CARTESIAN_POINT('Ctrl Pts',(10.7175941211066,-8.52323302742723,-4.71611549795234));
#53004=CARTESIAN_POINT('Ctrl Pts',(11.8206443092623,-8.6410972085384,-4.50214846820936));
#53005=CARTESIAN_POINT('Ctrl Pts',(12.8076886876858,-8.77604098409547,-4.23317354676162));
#53006=CARTESIAN_POINT('Ctrl Pts',(13.5599769262593,-8.87234107283724,-4.01612216898111));
#53007=CARTESIAN_POINT('Ctrl Pts',(14.1409849758931,-8.95311652054028,-3.82954437668286));
#53008=CARTESIAN_POINT('Ctrl Pts',(15.2001160349016,-9.11712726893695,-3.42890798831576));
#53009=CARTESIAN_POINT('Ctrl Pts',(15.9274644685005,-9.23361588248013,-3.10300037073481));
#53010=CARTESIAN_POINT('Ctrl Pts',(16.5321322282548,-9.3168092748402,-2.82432638267735));
#53011=CARTESIAN_POINT('Ctrl Pts',(16.8247613473468,-9.35683848526952,-2.68420632115728));
#53012=CARTESIAN_POINT('Ctrl Pts',(17.3791193144645,-9.43288731616673,-2.40020239788725));
#53013=CARTESIAN_POINT('Ctrl Pts',(18.3031725170504,-9.55581141304687,-1.88358773747688));
#53014=CARTESIAN_POINT('Ctrl Pts',(19.0238031811775,-9.63350132918122,-1.42657286581671));
#53015=CARTESIAN_POINT('Ctrl Pts',(19.7685846204969,-9.68548144316729,-0.948296989745364));
#53016=CARTESIAN_POINT('Ctrl Pts',(20.3333458124559,-9.71634622220616,-0.563870996202872));
#53017=CARTESIAN_POINT('Ctrl Pts',(21.3725234028357,-9.73790831668593,0.208452027128235));
#53018=CARTESIAN_POINT('Ctrl Pts',(22.0963502964542,-9.70493456228337,0.792620452508349));
#53019=CARTESIAN_POINT('Ctrl Pts',(23.2302898490711,-9.58941316697602,1.6990553747534));
#53020=CARTESIAN_POINT('Ctrl Pts',(23.8854423668127,-9.47051557491202,2.24929142641503));
#53021=CARTESIAN_POINT('Ctrl Pts',(24.5000000001022,-9.30357389606071,2.79427645741834));
#53022=CARTESIAN_POINT('Ctrl Pts',(2.1,-12.1206304302549,-6.83591261691419));
#53023=CARTESIAN_POINT('Ctrl Pts',(2.73333333333334,-12.1206304302549,-6.83591261691419));
#53024=CARTESIAN_POINT('Ctrl Pts',(3.36610615421361,-12.1206479194635,-6.83586470096514));
#53025=CARTESIAN_POINT('Ctrl Pts',(4.12374023994246,-12.1206529672983,-6.83585065866281));
#53026=CARTESIAN_POINT('Ctrl Pts',(4.36463581418031,-12.119818089853,-6.83736864158517));
#53027=CARTESIAN_POINT('Ctrl Pts',(4.85997530319406,-12.1159950337854,-6.84434016223762));
#53028=CARTESIAN_POINT('Ctrl Pts',(5.74109948643887,-12.1069511492505,-6.86086278899071));
#53029=CARTESIAN_POINT('Ctrl Pts',(6.52363773254301,-12.1067466533597,-6.8612742309798));
#53030=CARTESIAN_POINT('Ctrl Pts',(7.12000347701033,-12.1231781285262,-6.83101297830123));
#53031=CARTESIAN_POINT('Ctrl Pts',(7.24730650466272,-12.1268928519257,-6.82433786894958));
#53032=CARTESIAN_POINT('Ctrl Pts',(7.44359013132278,-12.1331371694334,-6.81335481350602));
#53033=CARTESIAN_POINT('Ctrl Pts',(7.63950249952398,-12.1399592237706,-6.80153737160822));
#53034=CARTESIAN_POINT('Ctrl Pts',(8.03411798341277,-12.1549085762698,-6.77580415828938));
#53035=CARTESIAN_POINT('Ctrl Pts',(8.63043086897818,-12.1823946115809,-6.72851622753706));
#53036=CARTESIAN_POINT('Ctrl Pts',(9.29097699605177,-12.2237061185676,-6.65361492414508));
#53037=CARTESIAN_POINT('Ctrl Pts',(9.81195534428169,-12.2644669019274,-6.57562981851048));
#53038=CARTESIAN_POINT('Ctrl Pts',(10.0691242294032,-12.2876662270862,-6.5297284806116));
#53039=CARTESIAN_POINT('Ctrl Pts',(10.7899280908924,-12.3576002597858,-6.38885954025546));
#53040=CARTESIAN_POINT('Ctrl Pts',(11.9161536741519,-12.5198279076047,-6.07413534771085));
#53041=CARTESIAN_POINT('Ctrl Pts',(12.9129363927331,-12.7028957202776,-5.68195632485753));
#53042=CARTESIAN_POINT('Ctrl Pts',(13.6692202156514,-12.8320205003908,-5.36700676384535));
#53043=CARTESIAN_POINT('Ctrl Pts',(14.2625054221329,-12.9416375398882,-5.09326044189235));
#53044=CARTESIAN_POINT('Ctrl Pts',(15.3322025816006,-13.1612208212938,-4.50953050507395));
#53045=CARTESIAN_POINT('Ctrl Pts',(16.0642045996111,-13.314626073984,-4.0376815807855));
#53046=CARTESIAN_POINT('Ctrl Pts',(16.6699064173536,-13.4217056458658,-3.63594477391126));
#53047=CARTESIAN_POINT('Ctrl Pts',(16.9656071732736,-13.4736500463097,-3.43229235011708));
#53048=CARTESIAN_POINT('Ctrl Pts',(17.5230947907728,-13.5709657994867,-3.02137001298369));
#53049=CARTESIAN_POINT('Ctrl Pts',(18.4506751005994,-13.7254773647144,-2.27570397276808));
#53050=CARTESIAN_POINT('Ctrl Pts',(19.1721322371942,-13.817061020641,-1.61983850524452));
#53051=CARTESIAN_POINT('Ctrl Pts',(19.9178174487373,-13.8707061847774,-0.934528745352126));
#53052=CARTESIAN_POINT('Ctrl Pts',(20.4828456339096,-13.8989929725084,-0.38350142317537));
#53053=CARTESIAN_POINT('Ctrl Pts',(21.519673087749,-13.8969871998656,0.719259828124072));
#53054=CARTESIAN_POINT('Ctrl Pts',(22.2434457172006,-13.8253355648101,1.55134793540283));
#53055=CARTESIAN_POINT('Ctrl Pts',(23.3781345297088,-13.6212597999766,2.84098795851428));
#53056=CARTESIAN_POINT('Ctrl Pts',(24.0312127056184,-13.4291220347533,3.62028744621722));
#53057=CARTESIAN_POINT('Ctrl Pts',(24.6419825553303,-13.1689424018865,4.38882031378994));
#53058=CARTESIAN_POINT('Ctrl Pts',(2.1,-20.916296133633,-11.071681975177));
#53059=CARTESIAN_POINT('Ctrl Pts',(2.73333333333333,-20.916296133633,-11.071681975177));
#53060=CARTESIAN_POINT('Ctrl Pts',(3.36563013999952,-20.9163457636086,-11.0715181247485));
#53061=CARTESIAN_POINT('Ctrl Pts',(4.12274830451023,-20.9163601418624,-11.0714694821853));
#53062=CARTESIAN_POINT('Ctrl Pts',(4.35698360829913,-20.9150398098762,-11.0740285474474));
#53063=CARTESIAN_POINT('Ctrl Pts',(4.84792376014415,-20.9089149916327,-11.085938742644));
#53064=CARTESIAN_POINT('Ctrl Pts',(5.73065667640276,-20.89427786353,-11.1144517034764));
#53065=CARTESIAN_POINT('Ctrl Pts',(6.536083377971,-20.8937138528347,-11.1155451125587));
#53066=CARTESIAN_POINT('Ctrl Pts',(7.15933923661711,-20.9213295292238,-11.0613487798922));
#53067=CARTESIAN_POINT('Ctrl Pts',(7.2869825297321,-20.9273577920289,-11.0497993277066));
#53068=CARTESIAN_POINT('Ctrl Pts',(7.48696545484876,-20.9376292512005,-11.0305502319027));
#53069=CARTESIAN_POINT('Ctrl Pts',(7.68596619463735,-20.9488334483803,-11.0098765165954));
#53070=CARTESIAN_POINT('Ctrl Pts',(8.0883162475225,-20.9734544781764,-10.9647379230039));
#53071=CARTESIAN_POINT('Ctrl Pts',(8.6988777287627,-21.0188908195159,-10.881420270716));
#53072=CARTESIAN_POINT('Ctrl Pts',(9.38136707068581,-21.0875686323605,-10.7485587482729));
#53073=CARTESIAN_POINT('Ctrl Pts',(9.92336660942117,-21.1557256018479,-10.6092802056132));
#53074=CARTESIAN_POINT('Ctrl Pts',(10.192104163104,-21.1946784819422,-10.5269158804284));
#53075=CARTESIAN_POINT('Ctrl Pts',(10.9468601756432,-21.312453368427,-10.2732554098091));
#53076=CARTESIAN_POINT('Ctrl Pts',(12.1070011864937,-21.5827620184303,-9.71110981143062));
#53077=CARTESIAN_POINT('Ctrl Pts',(13.1090760677711,-21.877961857721,-9.02824401297635));
#53078=CARTESIAN_POINT('Ctrl Pts',(13.8680231110403,-22.0833622460056,-8.48292378218801));
#53079=CARTESIAN_POINT('Ctrl Pts',(14.4653877431462,-22.2597779663279,-8.00456661480236));
#53080=CARTESIAN_POINT('Ctrl Pts',(15.5287361352249,-22.6051540387014,-7.00111172304811));
#53081=CARTESIAN_POINT('Ctrl Pts',(16.2553457094708,-22.8424976951966,-6.1930675108659));
#53082=CARTESIAN_POINT('Ctrl Pts',(16.859621896458,-23.0044889456917,-5.50458274371019));
#53083=CARTESIAN_POINT('Ctrl Pts',(17.1500351055466,-23.0826150095401,-5.1590775027475));
#53084=CARTESIAN_POINT('Ctrl Pts',(17.6990188169006,-23.2273294355939,-4.46234792132739));
#53085=CARTESIAN_POINT('Ctrl Pts',(18.611272879964,-23.452715685408,-3.20153979794507));
#53086=CARTESIAN_POINT('Ctrl Pts',(19.3245661130779,-23.5769499724595,-2.09052262543805));
#53087=CARTESIAN_POINT('Ctrl Pts',(20.0670920275141,-23.6354019998513,-0.924514657719357));
#53088=CARTESIAN_POINT('Ctrl Pts',(20.6170292347668,-23.6585283665091,-0.00486191135603094));
#53089=CARTESIAN_POINT('Ctrl Pts',(21.6396453273267,-23.6076069577787,1.84844937703413));
#53090=CARTESIAN_POINT('Ctrl Pts',(22.3556274201432,-23.4509610643206,3.24991333715251));
#53091=CARTESIAN_POINT('Ctrl Pts',(23.4868198684743,-23.0476613191845,5.43142402662265));
#53092=CARTESIAN_POINT('Ctrl Pts',(24.1253594022045,-22.6935861225115,6.72605099589447));
#53093=CARTESIAN_POINT('Ctrl Pts',(24.7277792021545,-22.2267622806559,8.00674483047698));
#53094=CARTESIAN_POINT('Ctrl Pts',(2.1,-29.7119618370111,-15.3074513334397));
#53095=CARTESIAN_POINT('Ctrl Pts',(2.73333333333334,-29.7119618370111,-15.3074513334397));
#53096=CARTESIAN_POINT('Ctrl Pts',(3.36509601826733,-29.7119996481889,-15.3073119398028));
#53097=CARTESIAN_POINT('Ctrl Pts',(4.12168472859039,-29.712009343078,-15.3072731750119));
#53098=CARTESIAN_POINT('Ctrl Pts',(4.34924335783325,-29.7102392280698,-15.3108028413304));
#53099=CARTESIAN_POINT('Ctrl Pts',(4.83584443000053,-29.7018839707635,-15.3275145646124));
#53100=CARTESIAN_POINT('Ctrl Pts',(5.71997740106937,-29.6816141052182,-15.3681101299536));
#53101=CARTESIAN_POINT('Ctrl Pts',(6.5487109251882,-29.6802918349395,-15.3707901137388));
#53102=CARTESIAN_POINT('Ctrl Pts',(7.19748317953822,-29.7204144003175,-15.2899276431913));
#53103=CARTESIAN_POINT('Ctrl Pts',(7.32544141258867,-29.7287738602123,-15.2734650442013));
#53104=CARTESIAN_POINT('Ctrl Pts',(7.52889917711157,-29.7432671926898,-15.2455421685912));
#53105=CARTESIAN_POINT('Ctrl Pts',(7.73075278971052,-29.7590297130559,-15.2156417671467));
#53106=CARTESIAN_POINT('Ctrl Pts',(8.14018479960674,-29.7937920094793,-15.1501008270889));
#53107=CARTESIAN_POINT('Ctrl Pts',(8.76324628290073,-29.858127960699,-15.028769624718));
#53108=CARTESIAN_POINT('Ctrl Pts',(9.46271315458471,-29.9559850568587,-14.8339981039036));
#53109=CARTESIAN_POINT('Ctrl Pts',(10.0175769787051,-30.0531863854985,-14.6296699075059));
#53110=CARTESIAN_POINT('Ctrl Pts',(10.2918333022463,-30.1086127962716,-14.5091281203088));
#53111=CARTESIAN_POINT('Ctrl Pts',(11.0595910066927,-30.2757018898991,-14.139070342574));
#53112=CARTESIAN_POINT('Ctrl Pts',(12.2112473457141,-30.648937612004,-13.3398925023309));
#53113=CARTESIAN_POINT('Ctrl Pts',(13.2033007010659,-31.0506537341638,-12.3812952012109));
#53114=CARTESIAN_POINT('Ctrl Pts',(13.9586007016383,-31.3305216353669,-11.6113351262395));
#53115=CARTESIAN_POINT('Ctrl Pts',(14.542598746085,-31.5670881163489,-10.9487986651389));
#53116=CARTESIAN_POINT('Ctrl Pts',(15.5913195536334,-32.0323898578073,-9.55125247564053));
#53117=CARTESIAN_POINT('Ctrl Pts',(16.3119173380708,-32.3531230926996,-8.41971069656156));
#53118=CARTESIAN_POINT('Ctrl Pts',(16.9149851983179,-32.5715645453592,-7.44764363908721));
#53119=CARTESIAN_POINT('Ctrl Pts',(17.2005121433669,-32.6749740884606,-6.96982244605168));
#53120=CARTESIAN_POINT('Ctrl Pts',(17.7438798901797,-32.8675630371451,-5.99886958229992));
#53121=CARTESIAN_POINT('Ctrl Pts',(18.6483251207895,-33.1666438231165,-4.23939596515499));
#53122=CARTESIAN_POINT('Ctrl Pts',(19.3595640666469,-33.3289092906231,-2.67776204570037));
#53123=CARTESIAN_POINT('Ctrl Pts',(20.101201047881,-33.3977844233599,-1.03303550949749));
#53124=CARTESIAN_POINT('Ctrl Pts',(20.6467829307123,-33.420235639171,0.247408307787539));
#53125=CARTESIAN_POINT('Ctrl Pts',(21.6665635858478,-33.3304451498286,2.84833137837582));
#53126=CARTESIAN_POINT('Ctrl Pts',(22.3811269169302,-33.0965818169693,4.81920574759241));
#53127=CARTESIAN_POINT('Ctrl Pts',(23.5117933107515,-32.5060407355254,7.89489191625015));
#53128=CARTESIAN_POINT('Ctrl Pts',(24.1480627906507,-31.997321521606,9.70668778292231));
#53129=CARTESIAN_POINT('Ctrl Pts',(24.7493903499091,-31.3302490010767,11.5032773646064));
#53130=CARTESIAN_POINT('Ctrl Pts',(2.1,-34.7380565246557,-17.7278909667327));
#53131=CARTESIAN_POINT('Ctrl Pts',(2.73333333333334,-34.7380565246557,-17.7278909667327));
#53132=CARTESIAN_POINT('Ctrl Pts',(3.36477003909008,-34.7380878504292,-17.7277685453303));
#53133=CARTESIAN_POINT('Ctrl Pts',(4.12105218050017,-34.7380950530209,-17.7277361764495));
#53134=CARTESIAN_POINT('Ctrl Pts',(4.34478769127088,-34.7360800768833,-17.7317954189765));
#53135=CARTESIAN_POINT('Ctrl Pts',(4.82894448622196,-34.7264782440274,-17.7511938998242));
#53136=CARTESIAN_POINT('Ctrl Pts',(5.71376767624365,-34.7029725862593,-17.798729519981));
#53137=CARTESIAN_POINT('Ctrl Pts',(6.55605736789038,-34.7011333795005,-17.8024966972734));
#53138=CARTESIAN_POINT('Ctrl Pts',(7.21867968559155,-34.7487778314302,-17.70561610612));
#53139=CARTESIAN_POINT('Ctrl Pts',(7.34680477302365,-34.758474208368,-17.6863351682917));
#53140=CARTESIAN_POINT('Ctrl Pts',(7.55212973160944,-34.7754330759594,-17.6533440413737));
#53141=CARTESIAN_POINT('Ctrl Pts',(7.75549216232999,-34.7938463390146,-17.6180735588395));
#53142=CARTESIAN_POINT('Ctrl Pts',(8.16863486466037,-34.8345191663954,-17.5406274875346));
#53143=CARTESIAN_POINT('Ctrl Pts',(8.79798512181356,-34.9098733771466,-17.3971072068904));
#53144=CARTESIAN_POINT('Ctrl Pts',(9.50495252296997,-35.0246122080616,-17.1664851984444));
#53145=CARTESIAN_POINT('Ctrl Pts',(10.0643544361655,-35.1382513636705,-16.9253010933509));
#53146=CARTESIAN_POINT('Ctrl Pts',(10.3400749108932,-35.2028268310511,-16.78351345817));
#53147=CARTESIAN_POINT('Ctrl Pts',(11.1102097451852,-35.3969765538676,-16.3494142249521));
#53148=CARTESIAN_POINT('Ctrl Pts',(12.2544661012045,-35.8260061974632,-15.4220345473532));
#53149=CARTESIAN_POINT('Ctrl Pts',(13.2427201344581,-36.2882744174662,-14.3078780733756));
#53150=CARTESIAN_POINT('Ctrl Pts',(13.9962152001074,-36.6106546545614,-13.410529882366));
#53151=CARTESIAN_POINT('Ctrl Pts',(14.5751544918282,-36.8812387280998,-12.6446491994453));
#53152=CARTESIAN_POINT('Ctrl Pts',(15.6190053721497,-37.4158411932568,-11.0215866115973));
#53153=CARTESIAN_POINT('Ctrl Pts',(16.3369858202403,-37.7847218374664,-9.7052068333357));
#53154=CARTESIAN_POINT('Ctrl Pts',(16.9394528589127,-38.0357988868014,-8.57126361777627));
#53155=CARTESIAN_POINT('Ctrl Pts',(17.2231900082674,-38.1539748657828,-8.01721712860961));
#53156=CARTESIAN_POINT('Ctrl Pts',(17.7643466428736,-38.3744634463336,-6.88860604294098));
#53157=CARTESIAN_POINT('Ctrl Pts',(18.665416776174,-38.7164782056892,-4.8425562907444));
#53158=CARTESIAN_POINT('Ctrl Pts',(19.3755688464135,-38.9009629285056,-3.02324311837983));
#53159=CARTESIAN_POINT('Ctrl Pts',(20.1168542434801,-38.9762754008698,-1.10510187804403));
#53160=CARTESIAN_POINT('Ctrl Pts',(20.6601247471566,-38.9987110260548,0.382680871312569));
#53161=CARTESIAN_POINT('Ctrl Pts',(21.6779306238709,-38.8871436088383,3.41175861162423));
#53162=CARTESIAN_POINT('Ctrl Pts',(22.3918707612037,-38.6096537271056,5.70820384366463));
#53163=CARTESIAN_POINT('Ctrl Pts',(23.5225369684879,-37.9128210548167,9.29489384117657));
#53164=CARTESIAN_POINT('Ctrl Pts',(24.157514841919,-37.3161464202365,11.4028407975047));
#53165=CARTESIAN_POINT('Ctrl Pts',(24.7577717974218,-36.5347967417974,13.4945033583609));
#53166=CARTESIAN_POINT('',(24.5,-9.30357389617668,2.7942764573609));
#53167=CARTESIAN_POINT('Ctrl Pts',(24.5,-9.30357389617668,2.7942764573609));
#53168=CARTESIAN_POINT('Ctrl Pts',(23.8274939346328,-9.6593359457179,2.26301432768217));
#53169=CARTESIAN_POINT('Ctrl Pts',(23.3366347313422,-9.90209213544415,1.88769087309693));
#53170=CARTESIAN_POINT('Ctrl Pts',(22.5855494187791,-10.2761542512457,1.30496983260268));
#53171=CARTESIAN_POINT('Ctrl Pts',(22.2454144272606,-10.4455512724061,1.04107994839));
#53172=CARTESIAN_POINT('Ctrl Pts',(21.838266074389,-10.649002408715,0.713024067302568));
#53173=CARTESIAN_POINT('Ctrl Pts',(21.380215694946,-10.8812747542395,0.336360818335602));
#53174=CARTESIAN_POINT('Ctrl Pts',(20.7694693292298,-11.1909775669692,-0.165867147691021));
#53175=CARTESIAN_POINT('Ctrl Pts',(20.162900303303,-11.5043313797733,-0.671800812422079));
#53176=CARTESIAN_POINT('Ctrl Pts',(19.5574857571565,-11.8416668907066,-1.16282656860098));
#53177=CARTESIAN_POINT('Ctrl Pts',(18.6418529409967,-12.3518552663123,-1.90545705014252));
#53178=CARTESIAN_POINT('Ctrl Pts',(17.7734813310041,-12.8807069946298,-2.69008889779871));
#53179=CARTESIAN_POINT('Ctrl Pts',(16.9621253090967,-13.4407209233415,-3.40811169367996));
#53180=CARTESIAN_POINT('Ctrl Pts',(16.8133360656621,-13.5434181937333,-3.53978517077668));
#53181=CARTESIAN_POINT('Ctrl Pts',(16.6656205363151,-13.6476856017606,-3.67035910850337));
#53182=CARTESIAN_POINT('Ctrl Pts',(16.5183901926363,-13.7540617624745,-3.80017688100675));
#53183=CARTESIAN_POINT('Ctrl Pts',(15.7264522887166,-14.3262489328485,-4.49845423388844));
#53184=CARTESIAN_POINT('Ctrl Pts',(14.9462259719641,-14.9411217657404,-5.26355621040781));
#53185=CARTESIAN_POINT('Ctrl Pts',(14.2963150415374,-15.5054551326937,-5.88914684389902));
#53186=CARTESIAN_POINT('Ctrl Pts',(13.9908350934413,-15.7707107540026,-6.18319543625432));
#53187=CARTESIAN_POINT('Ctrl Pts',(13.7077063567062,-16.0287137800868,-6.45459111782661));
#53188=CARTESIAN_POINT('Ctrl Pts',(13.4460198946299,-16.2769490901149,-6.70287044942663));
#53189=CARTESIAN_POINT('Ctrl Pts',(12.8373295405702,-16.8543516716327,-7.28037542640655));
#53190=CARTESIAN_POINT('Ctrl Pts',(12.3530827409722,-17.3494543756252,-7.77107105609639));
#53191=CARTESIAN_POINT('Ctrl Pts',(11.9770275688693,-17.7511354620811,-8.14810202886081));
#53192=CARTESIAN_POINT('Ctrl Pts',(11.6553972429219,-18.0946829741158,-8.4705669320408));
#53193=CARTESIAN_POINT('Ctrl Pts',(11.3684205615655,-18.4156350281444,-8.75884371968927));
#53194=CARTESIAN_POINT('Ctrl Pts',(11.071085678131,-18.7646456855957,-9.05375641021996));
#53195=CARTESIAN_POINT('Ctrl Pts',(10.8141787015647,-19.0662022058381,-9.30857053360867));
#53196=CARTESIAN_POINT('Ctrl Pts',(10.5576802661827,-19.3800705526631,-9.56028590215235));
#53197=CARTESIAN_POINT('Ctrl Pts',(10.2957959918397,-19.7169417339605,-9.81194913646659));
#53198=CARTESIAN_POINT('Ctrl Pts',(9.71459276345257,-20.4645643951982,-10.370468675743));
#53199=CARTESIAN_POINT('Ctrl Pts',(9.09527967376236,-21.3374886981073,-10.9426578680836));
#53200=CARTESIAN_POINT('Ctrl Pts',(8.43168033652658,-22.3859163093067,-11.5697730332091));
#53201=CARTESIAN_POINT('Ctrl Pts',(7.97964340480273,-23.1000942385303,-11.9969573282713));
#53202=CARTESIAN_POINT('Ctrl Pts',(7.52291961074464,-23.8750386166862,-12.4359459480503));
#53203=CARTESIAN_POINT('Ctrl Pts',(7.10363554125516,-24.632641914712,-12.8547349765663));
#53204=CARTESIAN_POINT('Ctrl Pts',(6.5632779955478,-25.6090125629922,-13.3944545320783));
#53205=CARTESIAN_POINT('Ctrl Pts',(6.08559840022222,-26.564462963399,-13.8602159500353));
#53206=CARTESIAN_POINT('Ctrl Pts',(5.6170867082795,-27.5711979548747,-14.333880928108));
#53207=CARTESIAN_POINT('Ctrl Pts',(5.04102956503258,-28.8090259390419,-14.9162742788338));
#53208=CARTESIAN_POINT('Ctrl Pts',(4.50102820503081,-30.086306522799,-15.4877262328007));
#53209=CARTESIAN_POINT('Ctrl Pts',(4.,-31.3543250987725,-16.098371795166));
#53210=CARTESIAN_POINT('Ctrl Pts',(3.72183418897184,-32.0583162354846,-16.4373960584719));
#53211=CARTESIAN_POINT('Ctrl Pts',(3.45538353518254,-32.7656113591521,-16.7780114380366));
#53212=CARTESIAN_POINT('Ctrl Pts',(3.2,-33.4762280926097,-17.1202264205697));
#53213=CARTESIAN_POINT('',(24.5,-25.5759818995428,8.65269610435146));
#53214=CARTESIAN_POINT('Ctrl Pts',(24.5,-25.5759818995428,8.65269610435144));
#53215=CARTESIAN_POINT('Ctrl Pts',(24.5,-24.4075774169203,8.24137805333807));
#53216=CARTESIAN_POINT('Ctrl Pts',(24.5,-23.2592813076738,7.83618130765631));
#53217=CARTESIAN_POINT('Ctrl Pts',(24.5,-18.5158678907521,6.15728495615527));
#53218=CARTESIAN_POINT('Ctrl Pts',(24.5,-13.4830088728325,4.36655158825629));
#53219=CARTESIAN_POINT('Ctrl Pts',(24.5,-9.30357389617668,2.7942764573609));
#53220=CARTESIAN_POINT('',(10.2670750393577,-30.770480162676,-14.8182822548653));
#53221=CARTESIAN_POINT('Ctrl Pts',(10.2670750393577,-30.770480162676,-14.8182822548653));
#53222=CARTESIAN_POINT('Ctrl Pts',(11.2293198185888,-30.1791102527654,-14.0169036234914));
#53223=CARTESIAN_POINT('Ctrl Pts',(12.092802582344,-29.8393707151449,-13.0968030075364));
#53224=CARTESIAN_POINT('Ctrl Pts',(14.3080979519049,-29.1888831332163,-10.4908414553475));
#53225=CARTESIAN_POINT('Ctrl Pts',(14.8952017874601,-29.0927432444532,-9.72024139342426));
#53226=CARTESIAN_POINT('Ctrl Pts',(17.0803363586062,-28.7592866386632,-6.39544722949815));
#53227=CARTESIAN_POINT('Ctrl Pts',(17.6922811489506,-28.6652489345692,-5.38383065662599));
#53228=CARTESIAN_POINT('Ctrl Pts',(19.0755427322033,-28.4267546017089,-2.90463394754129));
#53229=CARTESIAN_POINT('Ctrl Pts',(20.2687424742408,-28.1812035390717,-0.681869641908761));
#53230=CARTESIAN_POINT('Ctrl Pts',(22.3267279388309,-27.2670721892073,3.7530051527172));
#53231=CARTESIAN_POINT('Ctrl Pts',(23.4192562717209,-26.6256746472157,6.1252840113241));
#53232=CARTESIAN_POINT('Ctrl Pts',(24.5,-25.5759818995428,8.65269610435144));
#53233=CARTESIAN_POINT('Ctrl Pts',(6.,-34.705361282547,-17.7915119719457));
#53234=CARTESIAN_POINT('Ctrl Pts',(7.51604047332548,-32.7628371673734,-16.8524804320582));
#53235=CARTESIAN_POINT('Ctrl Pts',(9.08449301626627,-31.5752575158279,-15.7405257307418));
#53236=CARTESIAN_POINT('Ctrl Pts',(9.8624969752411,-31.0279962027639,-15.1470785535203));
#53237=CARTESIAN_POINT('Ctrl Pts',(10.0667253012216,-30.8936097541786,-14.9851379265292));
#53238=CARTESIAN_POINT('Ctrl Pts',(10.2670750393577,-30.770480162676,-14.8182822548653));
#53239=CARTESIAN_POINT('Origin',(24.5,-7.65823537717056,-3.68801178249924));
#53240=CARTESIAN_POINT('',(24.5,-8.27152931289795,5.09374822578144));
#53241=CARTESIAN_POINT('Ctrl Pts',(24.5,-8.27152931289795,5.09374822578144));
#53242=CARTESIAN_POINT('Ctrl Pts',(24.5,-8.44222149420361,4.81656817710801));
#53243=CARTESIAN_POINT('Ctrl Pts',(24.5,-8.59911506421257,4.53059124178116));
#53244=CARTESIAN_POINT('Ctrl Pts',(24.5,-8.96745037775474,3.77063565908301));
#53245=CARTESIAN_POINT('Ctrl Pts',(24.5,-9.15522875621099,3.28819321644671));
#53246=CARTESIAN_POINT('Ctrl Pts',(24.5,-9.30357389617668,2.7942764573609));
#53247=CARTESIAN_POINT('',(24.5,-23.4219747427337,13.431719888039));
#53248=CARTESIAN_POINT('Ctrl Pts',(24.5,-8.27152931289795,5.09374822578144));
#53249=CARTESIAN_POINT('Ctrl Pts',(24.5,-12.0766273202602,7.113542304172));
#53250=CARTESIAN_POINT('Ctrl Pts',(24.5,-17.1057664725757,9.89787449294439));
#53251=CARTESIAN_POINT('Ctrl Pts',(24.5,-23.4219747427337,13.4317198880391));
#53252=CARTESIAN_POINT('Origin',(24.5,0.,0.));
#53253=CARTESIAN_POINT('Ctrl Pts',(24.5,-23.4219746022546,13.4317201330038));
#53254=CARTESIAN_POINT('Ctrl Pts',(24.5,-30.4957974083931,1.09652430807625));
#53255=CARTESIAN_POINT('Ctrl Pts',(24.5,-24.3261594333653,-11.7148609561741));
#53256=CARTESIAN_POINT('Ctrl Pts',(24.5,-12.6112984771912,-36.0410203895394));
#53257=CARTESIAN_POINT('Ctrl Pts',(24.5,11.7148609561741,-24.3261594333653));
#53258=CARTESIAN_POINT('Ctrl Pts',(24.5,36.0410203895394,-12.6112984771912));
#53259=CARTESIAN_POINT('Ctrl Pts',(24.5,24.3261594333653,11.7148609561741));
#53260=CARTESIAN_POINT('Ctrl Pts',(24.5,12.6112984771912,36.0410203895394));
#53261=CARTESIAN_POINT('Ctrl Pts',(24.5,-11.7148609561741,24.3261594333653));
#53262=CARTESIAN_POINT('Ctrl Pts',(24.5,-19.2573690718243,20.6938789627184));
#53263=CARTESIAN_POINT('Ctrl Pts',(24.5,-23.4219746022546,13.4317201330038));
#53264=CARTESIAN_POINT('Ctrl Pts',(24.3078118955742,-23.4504162085652,13.4480304442642));
#53265=CARTESIAN_POINT('Ctrl Pts',(24.3078118955742,-30.5328288491125,1.09785583170779));
#53266=CARTESIAN_POINT('Ctrl Pts',(24.3078118955742,-24.355699002996,-11.7290864631587));
#53267=CARTESIAN_POINT('Ctrl Pts',(24.3078118955742,-12.6266125398373,-36.0847854661547));
#53268=CARTESIAN_POINT('Ctrl Pts',(24.3078118955742,11.7290864631587,-24.355699002996));
#53269=CARTESIAN_POINT('Ctrl Pts',(24.3078118955742,36.0847854661547,-12.6266125398373));
#53270=CARTESIAN_POINT('Ctrl Pts',(24.3078118955742,24.355699002996,11.7290864631587));
#53271=CARTESIAN_POINT('Ctrl Pts',(24.3078118955742,12.6266125398373,36.0847854661547));
#53272=CARTESIAN_POINT('Ctrl Pts',(24.3078118955742,-11.7290864631587,24.355699002996));
#53273=CARTESIAN_POINT('Ctrl Pts',(24.3078118955742,-19.2807535438433,20.7190078072539));
#53274=CARTESIAN_POINT('Ctrl Pts',(24.3078118955742,-23.4504162085652,13.4480304442642));
#53275=CARTESIAN_POINT('Ctrl Pts',(23.9225830034177,-23.5109122482986,13.4827229024644));
#53276=CARTESIAN_POINT('Ctrl Pts',(23.9225830034177,-30.6115956910654,1.10068801726159));
#53277=CARTESIAN_POINT('Ctrl Pts',(23.9225830034177,-24.4185304393985,-11.7593444881934));
#53278=CARTESIAN_POINT('Ctrl Pts',(23.9225830034177,-12.6591859512051,-36.1778749275919));
#53279=CARTESIAN_POINT('Ctrl Pts',(23.9225830034177,11.7593444881934,-24.4185304393985));
#53280=CARTESIAN_POINT('Ctrl Pts',(23.9225830034177,36.1778749275919,-12.6591859512051));
#53281=CARTESIAN_POINT('Ctrl Pts',(23.9225830034177,24.4185304393985,11.7593444881934));
#53282=CARTESIAN_POINT('Ctrl Pts',(23.9225830034177,12.6591859512051,36.1778749275919));
#53283=CARTESIAN_POINT('Ctrl Pts',(23.9225830034177,-11.7593444881934,24.4185304393985));
#53284=CARTESIAN_POINT('Ctrl Pts',(23.9225830034177,-19.330492926808,20.7724575161375));
#53285=CARTESIAN_POINT('Ctrl Pts',(23.9225830034177,-23.5109122482986,13.4827229024644));
#53286=CARTESIAN_POINT('Ctrl Pts',(23.3421815947946,-23.6124947526602,13.5409770758279));
#53287=CARTESIAN_POINT('Ctrl Pts',(23.3421815947946,-30.7438577879148,1.10544370875214));
#53288=CARTESIAN_POINT('Ctrl Pts',(23.3421815947946,-24.5240344474382,-11.8101525406477));
#53289=CARTESIAN_POINT('Ctrl Pts',(23.3421815947946,-12.7138819067904,-36.3341869880859));
#53290=CARTESIAN_POINT('Ctrl Pts',(23.3421815947946,11.8101525406477,-24.5240344474382));
#53291=CARTESIAN_POINT('Ctrl Pts',(23.3421815947946,36.3341869880859,-12.7138819067904));
#53292=CARTESIAN_POINT('Ctrl Pts',(23.3421815947946,24.5240344474382,11.8101525406477));
#53293=CARTESIAN_POINT('Ctrl Pts',(23.3421815947946,12.7138819067904,36.3341869880859));
#53294=CARTESIAN_POINT('Ctrl Pts',(23.3421815947946,-11.8101525406477,24.5240344474382));
#53295=CARTESIAN_POINT('Ctrl Pts',(23.3421815947946,-19.4140132879625,20.8622081065845));
#53296=CARTESIAN_POINT('Ctrl Pts',(23.3421815947946,-23.6124947526602,13.5409770758279));
#53297=CARTESIAN_POINT('Ctrl Pts',(22.5631762070947,-23.7697037387964,13.631131178547));
#53298=CARTESIAN_POINT('Ctrl Pts',(22.5631762070947,-30.9485464819043,1.11280361233302));
#53299=CARTESIAN_POINT('Ctrl Pts',(22.5631762070947,-24.6873123488983,-11.8887830338031));
#53300=CARTESIAN_POINT('Ctrl Pts',(22.5631762070947,-12.7985293150952,-36.5760953827013));
#53301=CARTESIAN_POINT('Ctrl Pts',(22.5631762070947,11.8887830338031,-24.6873123488983));
#53302=CARTESIAN_POINT('Ctrl Pts',(22.5631762070947,36.5760953827013,-12.7985293150952));
#53303=CARTESIAN_POINT('Ctrl Pts',(22.5631762070947,24.6873123488983,11.8887830338031));
#53304=CARTESIAN_POINT('Ctrl Pts',(22.5631762070947,12.7985293150952,36.5760953827013));
#53305=CARTESIAN_POINT('Ctrl Pts',(22.5631762070947,-11.8887830338031,24.6873123488983));
#53306=CARTESIAN_POINT('Ctrl Pts',(22.5631762070947,-19.5432693186279,21.0011060341163));
#53307=CARTESIAN_POINT('Ctrl Pts',(22.5631762070947,-23.7697037387964,13.631131178547));
#53308=CARTESIAN_POINT('Ctrl Pts',(21.5808622776984,-24.0031263055443,13.764991224189));
#53309=CARTESIAN_POINT('Ctrl Pts',(21.5808622776984,-31.2524665154187,1.12373153462988));
#53310=CARTESIAN_POINT('Ctrl Pts',(21.5808622776984,-24.929745989549,-12.0055329218856));
#53311=CARTESIAN_POINT('Ctrl Pts',(21.5808622776984,-12.9242130676634,-36.9352789114346));
#53312=CARTESIAN_POINT('Ctrl Pts',(21.5808622776984,12.0055329218856,-24.929745989549));
#53313=CARTESIAN_POINT('Ctrl Pts',(21.5808622776984,36.9352789114346,-12.9242130676634));
#53314=CARTESIAN_POINT('Ctrl Pts',(21.5808622776984,24.929745989549,12.0055329218856));
#53315=CARTESIAN_POINT('Ctrl Pts',(21.5808622776984,12.9242130676634,36.9352789114346));
#53316=CARTESIAN_POINT('Ctrl Pts',(21.5808622776984,-12.0055329218856,24.929745989549));
#53317=CARTESIAN_POINT('Ctrl Pts',(21.5808622776984,-19.73518757462,21.2073404966446));
#53318=CARTESIAN_POINT('Ctrl Pts',(21.5808622776984,-24.0031263055443,13.764991224189));
#53319=CARTESIAN_POINT('Ctrl Pts',(20.5902243197586,-24.2744594023058,13.9205916925702));
#53320=CARTESIAN_POINT('Ctrl Pts',(20.5902243197586,-31.6057466845567,1.13643427815331));
#53321=CARTESIAN_POINT('Ctrl Pts',(20.5902243197586,-25.2115536630461,-12.141244344827));
#53322=CARTESIAN_POINT('Ctrl Pts',(20.5902243197586,-13.0703093182191,-37.3527980078731));
#53323=CARTESIAN_POINT('Ctrl Pts',(20.5902243197586,12.141244344827,-25.2115536630461));
#53324=CARTESIAN_POINT('Ctrl Pts',(20.5902243197586,37.3527980078731,-13.0703093182191));
#53325=CARTESIAN_POINT('Ctrl Pts',(20.5902243197586,25.2115536630461,12.141244344827));
#53326=CARTESIAN_POINT('Ctrl Pts',(20.5902243197586,13.0703093182191,37.3527980078731));
#53327=CARTESIAN_POINT('Ctrl Pts',(20.5902243197586,-12.141244344827,25.2115536630461));
#53328=CARTESIAN_POINT('Ctrl Pts',(20.5902243197586,-19.9582755795585,21.4470698259737));
#53329=CARTESIAN_POINT('Ctrl Pts',(20.5902243197586,-24.2744594023058,13.9205916925702));
#53330=CARTESIAN_POINT('Ctrl Pts',(19.591895069338,-24.5849847342196,14.098667598778));
#53331=CARTESIAN_POINT('Ctrl Pts',(19.591895069338,-32.0100557905577,1.15097184727372));
#53332=CARTESIAN_POINT('Ctrl Pts',(19.591895069338,-25.5340665536333,-12.296558367172));
#53333=CARTESIAN_POINT('Ctrl Pts',(19.591895069338,-13.2375081864613,-37.8306249208053));
#53334=CARTESIAN_POINT('Ctrl Pts',(19.591895069338,12.296558367172,-25.5340665536333));
#53335=CARTESIAN_POINT('Ctrl Pts',(19.591895069338,37.8306249208053,-13.2375081864613));
#53336=CARTESIAN_POINT('Ctrl Pts',(19.591895069338,25.5340665536333,12.296558367172));
#53337=CARTESIAN_POINT('Ctrl Pts',(19.591895069338,13.2375081864613,37.8306249208053));
#53338=CARTESIAN_POINT('Ctrl Pts',(19.591895069338,-12.296558367172,25.5340665536333));
#53339=CARTESIAN_POINT('Ctrl Pts',(19.591895069338,-20.2135871416434,21.721426439479));
#53340=CARTESIAN_POINT('Ctrl Pts',(19.591895069338,-24.5849847342196,14.098667598778));
#53341=CARTESIAN_POINT('Ctrl Pts',(18.5871162949016,-24.9361756654508,14.3000638679505));
#53342=CARTESIAN_POINT('Ctrl Pts',(18.5871162949016,-32.4673121778761,1.16741321907992));
#53343=CARTESIAN_POINT('Ctrl Pts',(18.5871162949016,-25.8988149034099,-12.4722119146764));
#53344=CARTESIAN_POINT('Ctrl Pts',(18.5871162949016,-13.4266029887335,-38.3710268180862));
#53345=CARTESIAN_POINT('Ctrl Pts',(18.5871162949016,12.4722119146764,-25.8988149034099));
#53346=CARTESIAN_POINT('Ctrl Pts',(18.5871162949016,38.3710268180862,-13.4266029887335));
#53347=CARTESIAN_POINT('Ctrl Pts',(18.5871162949016,25.8988149034099,12.4722119146764));
#53348=CARTESIAN_POINT('Ctrl Pts',(18.5871162949016,13.4266029887335,38.3710268180862));
#53349=CARTESIAN_POINT('Ctrl Pts',(18.5871162949016,-12.4722119146764,25.8988149034099));
#53350=CARTESIAN_POINT('Ctrl Pts',(18.5871162949016,-20.502333649666,22.0317120899042));
#53351=CARTESIAN_POINT('Ctrl Pts',(18.5871162949016,-24.9361756654508,14.3000638679505));
#53352=CARTESIAN_POINT('Ctrl Pts',(17.577868433379,-25.329524499683,14.5256362864067));
#53353=CARTESIAN_POINT('Ctrl Pts',(17.577868433379,-32.9794588505319,1.1858282573341));
#53354=CARTESIAN_POINT('Ctrl Pts',(17.577868433379,-26.3073486251372,-12.6689513859872));
#53355=CARTESIAN_POINT('Ctrl Pts',(17.577868433379,-13.63839723915,-38.9763000111244));
#53356=CARTESIAN_POINT('Ctrl Pts',(17.577868433379,12.6689513859872,-26.3073486251372));
#53357=CARTESIAN_POINT('Ctrl Pts',(17.577868433379,38.9763000111244,-13.63839723915));
#53358=CARTESIAN_POINT('Ctrl Pts',(17.577868433379,26.3073486251372,12.6689513859872));
#53359=CARTESIAN_POINT('Ctrl Pts',(17.577868433379,13.63839723915,38.9763000111244));
#53360=CARTESIAN_POINT('Ctrl Pts',(17.577868433379,-12.6689513859872,26.3073486251372));
#53361=CARTESIAN_POINT('Ctrl Pts',(17.577868433379,-20.8257420643457,22.3792452635139));
#53362=CARTESIAN_POINT('Ctrl Pts',(17.577868433379,-25.329524499683,14.5256362864067));
#53363=CARTESIAN_POINT('Ctrl Pts',(16.5668667015923,-25.7662789188368,14.7761003580551));
#53364=CARTESIAN_POINT('Ctrl Pts',(16.5668667015923,-33.5481203109731,1.20627537357407));
#53365=CARTESIAN_POINT('Ctrl Pts',(16.5668667015923,-26.7609635664043,-12.8874008284133));
#53366=CARTESIAN_POINT('Ctrl Pts',(16.5668667015923,-13.873562737991,-39.6483643948176));
#53367=CARTESIAN_POINT('Ctrl Pts',(16.5668667015923,12.8874008284133,-26.7609635664043));
#53368=CARTESIAN_POINT('Ctrl Pts',(16.5668667015923,39.6483643948176,-13.873562737991));
#53369=CARTESIAN_POINT('Ctrl Pts',(16.5668667015923,26.7609635664043,12.8874008284133));
#53370=CARTESIAN_POINT('Ctrl Pts',(16.5668667015923,13.873562737991,39.6483643948176));
#53371=CARTESIAN_POINT('Ctrl Pts',(16.5668667015923,-12.8874008284133,26.7609635664043));
#53372=CARTESIAN_POINT('Ctrl Pts',(16.5668667015923,-21.1848382202515,22.7651283173505));
#53373=CARTESIAN_POINT('Ctrl Pts',(16.5668667015923,-25.7662789188368,14.7761003580551));
#53374=CARTESIAN_POINT('Ctrl Pts',(15.5576189940876,-26.2471324113782,15.0518537753682));
#53375=CARTESIAN_POINT('Ctrl Pts',(15.5576189940876,-34.1741994926254,1.22878703418975));
#53376=CARTESIAN_POINT('Ctrl Pts',(15.5576189940876,-27.2603799871926,-13.1279071008807));
#53377=CARTESIAN_POINT('Ctrl Pts',(15.5576189940876,-14.132472886312,-40.3882870880733));
#53378=CARTESIAN_POINT('Ctrl Pts',(15.5576189940876,13.1279071008807,-27.2603799871926));
#53379=CARTESIAN_POINT('Ctrl Pts',(15.5576189940876,40.3882870880733,-14.132472886312));
#53380=CARTESIAN_POINT('Ctrl Pts',(15.5576189940876,27.2603799871926,13.1279071008807));
#53381=CARTESIAN_POINT('Ctrl Pts',(15.5576189940876,14.132472886312,40.3882870880733));
#53382=CARTESIAN_POINT('Ctrl Pts',(15.5576189940876,-13.1279071008807,27.2603799871926));
#53383=CARTESIAN_POINT('Ctrl Pts',(15.5576189940876,-21.580192298317,23.1899739651847));
#53384=CARTESIAN_POINT('Ctrl Pts',(15.5576189940876,-26.2471324113782,15.0518537753682));
#53385=CARTESIAN_POINT('Ctrl Pts',(14.5544447688713,-26.7719304659624,15.3528079312506));
#53386=CARTESIAN_POINT('Ctrl Pts',(14.5544447688713,-34.8574952191684,1.25335600557047));
#53387=CARTESIAN_POINT('Ctrl Pts',(14.5544447688713,-27.805437411382,-13.3903929221629));
#53388=CARTESIAN_POINT('Ctrl Pts',(14.5544447688713,-14.4150444892191,-41.1958303335449));
#53389=CARTESIAN_POINT('Ctrl Pts',(14.5544447688713,13.3903929221629,-27.805437411382));
#53390=CARTESIAN_POINT('Ctrl Pts',(14.5544447688713,41.1958303335449,-14.4150444892191));
#53391=CARTESIAN_POINT('Ctrl Pts',(14.5544447688713,27.805437411382,13.3903929221629));
#53392=CARTESIAN_POINT('Ctrl Pts',(14.5544447688713,14.4150444892191,41.1958303335449));
#53393=CARTESIAN_POINT('Ctrl Pts',(14.5544447688713,-13.3903929221629,27.805437411382));
#53394=CARTESIAN_POINT('Ctrl Pts',(14.5544447688713,-22.0116772604913,23.6536456925202));
#53395=CARTESIAN_POINT('Ctrl Pts',(14.5544447688713,-26.7719304659624,15.3528079312506));
#53396=CARTESIAN_POINT('Ctrl Pts',(13.5625963827217,-27.3391811060136,15.6781072269685));
#53397=CARTESIAN_POINT('Ctrl Pts',(13.5625963827217,-35.596064912482,1.27991243926791));
#53398=CARTESIAN_POINT('Ctrl Pts',(13.5625963827217,-28.3945862659469,-13.6741120572209));
#53399=CARTESIAN_POINT('Ctrl Pts',(13.5625963827217,-14.720474208726,-42.0686983231678));
#53400=CARTESIAN_POINT('Ctrl Pts',(13.5625963827217,13.6741120572209,-28.3945862659469));
#53401=CARTESIAN_POINT('Ctrl Pts',(13.5625963827217,42.0686983231678,-14.720474208726));
#53402=CARTESIAN_POINT('Ctrl Pts',(13.5625963827217,28.3945862659469,13.6741120572209));
#53403=CARTESIAN_POINT('Ctrl Pts',(13.5625963827217,14.720474208726,42.0686983231678));
#53404=CARTESIAN_POINT('Ctrl Pts',(13.5625963827217,-13.6741120572209,28.3945862659469));
#53405=CARTESIAN_POINT('Ctrl Pts',(13.5625963827217,-22.4780664150012,24.1548253021));
#53406=CARTESIAN_POINT('Ctrl Pts',(13.5625963827217,-27.3391811060136,15.6781072269685));
#53407=CARTESIAN_POINT('Ctrl Pts',(12.5880795783847,-27.9460475476476,16.0261248617137));
#53408=CARTESIAN_POINT('Ctrl Pts',(12.5880795783847,-36.3862150331401,1.30832352826907));
#53409=CARTESIAN_POINT('Ctrl Pts',(12.5880795783847,-29.0248802554437,-13.9776456449495));
#53410=CARTESIAN_POINT('Ctrl Pts',(12.5880795783847,-15.0472346104942,-43.0025259003932));
#53411=CARTESIAN_POINT('Ctrl Pts',(12.5880795783847,13.9776456449495,-29.0248802554437));
#53412=CARTESIAN_POINT('Ctrl Pts',(12.5880795783847,43.0025259003932,-15.0472346104942));
#53413=CARTESIAN_POINT('Ctrl Pts',(12.5880795783847,29.0248802554437,13.9776456449495));
#53414=CARTESIAN_POINT('Ctrl Pts',(12.5880795783847,15.0472346104942,43.0025259003932));
#53415=CARTESIAN_POINT('Ctrl Pts',(12.5880795783847,-13.9776456449495,29.0248802554437));
#53416=CARTESIAN_POINT('Ctrl Pts',(12.5880795783847,-22.9770273797494,24.691006427004));
#53417=CARTESIAN_POINT('Ctrl Pts',(12.5880795783847,-27.9460475476476,16.0261248617137));
#53418=CARTESIAN_POINT('Ctrl Pts',(11.6370973936883,-28.5889671307382,16.394817768898));
#53419=CARTESIAN_POINT('Ctrl Pts',(11.6370973936883,-37.2233069388725,1.33842248290329));
#53420=CARTESIAN_POINT('Ctrl Pts',(11.6370973936883,-29.6926191863701,-14.2992117660733));
#53421=CARTESIAN_POINT('Ctrl Pts',(11.6370973936883,-15.3934074202968,-43.9918309524434));
#53422=CARTESIAN_POINT('Ctrl Pts',(11.6370973936883,14.2992117660733,-29.6926191863701));
#53423=CARTESIAN_POINT('Ctrl Pts',(11.6370973936883,43.9918309524434,-15.3934074202968));
#53424=CARTESIAN_POINT('Ctrl Pts',(11.6370973936883,29.6926191863701,14.2992117660733));
#53425=CARTESIAN_POINT('Ctrl Pts',(11.6370973936883,15.3934074202968,43.9918309524434));
#53426=CARTESIAN_POINT('Ctrl Pts',(11.6370973936883,-14.2992117660733,29.6926191863701));
#53427=CARTESIAN_POINT('Ctrl Pts',(11.6370973936883,-23.5056309627235,25.259041371161));
#53428=CARTESIAN_POINT('Ctrl Pts',(11.6370973936883,-28.5889671307382,16.394817768898));
#53429=CARTESIAN_POINT('Ctrl Pts',(10.7155646400367,-29.2640651345263,16.7819639255827));
#53430=CARTESIAN_POINT('Ctrl Pts',(10.7155646400367,-38.1022956793159,1.37002790405408));
#53431=CARTESIAN_POINT('Ctrl Pts',(10.7155646400367,-30.3937787577631,-14.6368724193901));
#53432=CARTESIAN_POINT('Ctrl Pts',(10.7155646400367,-15.756906338373,-45.0306511771533));
#53433=CARTESIAN_POINT('Ctrl Pts',(10.7155646400367,14.6368724193901,-30.3937787577631));
#53434=CARTESIAN_POINT('Ctrl Pts',(10.7155646400367,45.0306511771533,-15.756906338373));
#53435=CARTESIAN_POINT('Ctrl Pts',(10.7155646400367,30.3937787577631,14.6368724193901));
#53436=CARTESIAN_POINT('Ctrl Pts',(10.7155646400367,15.756906338373,45.0306511771533));
#53437=CARTESIAN_POINT('Ctrl Pts',(10.7155646400367,-14.6368724193901,30.3937787577631));
#53438=CARTESIAN_POINT('Ctrl Pts',(10.7155646400367,-24.0606913980357,25.8555067254108));
#53439=CARTESIAN_POINT('Ctrl Pts',(10.7155646400367,-29.2640651345263,16.7819639255827));
#53440=CARTESIAN_POINT('Ctrl Pts',(9.82859575068344,-29.9675923231116,17.1854132702049));
#53441=CARTESIAN_POINT('Ctrl Pts',(9.82859575068344,-39.0182996874633,1.40296426731023));
#53442=CARTESIAN_POINT('Ctrl Pts',(9.82859575068344,-31.1244649977519,-14.9887523668806));
#53443=CARTESIAN_POINT('Ctrl Pts',(9.82859575068344,-16.1357126308712,-46.1132173646325));
#53444=CARTESIAN_POINT('Ctrl Pts',(9.82859575068344,14.9887523668806,-31.1244649977519));
#53445=CARTESIAN_POINT('Ctrl Pts',(9.82859575068344,46.1132173646325,-16.1357126308712));
#53446=CARTESIAN_POINT('Ctrl Pts',(9.82859575068344,31.1244649977519,14.9887523668806));
#53447=CARTESIAN_POINT('Ctrl Pts',(9.82859575068344,16.1357126308712,46.1132173646325));
#53448=CARTESIAN_POINT('Ctrl Pts',(9.82859575068344,-14.9887523668806,31.1244649977519));
#53449=CARTESIAN_POINT('Ctrl Pts',(9.82859575068344,-24.6391260924933,26.4770899494897));
#53450=CARTESIAN_POINT('Ctrl Pts',(9.82859575068344,-29.9675923231116,17.1854132702049));
#53451=CARTESIAN_POINT('Ctrl Pts',(8.97989469943246,-30.6963420508599,17.6033268985962));
#53452=CARTESIAN_POINT('Ctrl Pts',(8.97989469943246,-39.9671438577877,1.43708145019297));
#53453=CARTESIAN_POINT('Ctrl Pts',(8.97989469943246,-31.8813474709538,-15.3532477553949));
#53454=CARTESIAN_POINT('Ctrl Pts',(8.97989469943246,-16.5280997155589,-47.2345952263487));
#53455=CARTESIAN_POINT('Ctrl Pts',(8.97989469943246,15.3532477553949,-31.8813474709538));
#53456=CARTESIAN_POINT('Ctrl Pts',(8.97989469943246,47.2345952263487,-16.5280997155589));
#53457=CARTESIAN_POINT('Ctrl Pts',(8.97989469943246,31.8813474709538,15.3532477553949));
#53458=CARTESIAN_POINT('Ctrl Pts',(8.97989469943246,16.5280997155589,47.2345952263487));
#53459=CARTESIAN_POINT('Ctrl Pts',(8.97989469943246,-15.3532477553949,31.8813474709538));
#53460=CARTESIAN_POINT('Ctrl Pts',(8.97989469943246,-25.2382985664866,27.1209578947093));
#53461=CARTESIAN_POINT('Ctrl Pts',(8.97989469943246,-30.6963420508599,17.6033268985962));
#53462=CARTESIAN_POINT('Ctrl Pts',(8.1713316609345,-31.4479687613503,18.0343597124917));
#53463=CARTESIAN_POINT('Ctrl Pts',(8.1713316609345,-40.9457742371258,1.47226964301821));
#53464=CARTESIAN_POINT('Ctrl Pts',(8.1713316609345,-32.6619900727951,-15.7291854188016));
#53465=CARTESIAN_POINT('Ctrl Pts',(8.1713316609345,-16.9328046539935,-48.3911754915967));
#53466=CARTESIAN_POINT('Ctrl Pts',(8.1713316609345,15.7291854188016,-32.6619900727951));
#53467=CARTESIAN_POINT('Ctrl Pts',(8.1713316609345,48.3911754915967,-16.9328046539935));
#53468=CARTESIAN_POINT('Ctrl Pts',(8.1713316609345,32.6619900727951,15.7291854188016));
#53469=CARTESIAN_POINT('Ctrl Pts',(8.1713316609345,16.9328046539935,48.3911754915967));
#53470=CARTESIAN_POINT('Ctrl Pts',(8.1713316609345,-15.7291854188016,32.6619900727951));
#53471=CARTESIAN_POINT('Ctrl Pts',(8.1713316609345,-25.8562803213964,27.7850382054503));
#53472=CARTESIAN_POINT('Ctrl Pts',(8.1713316609345,-31.4479687613503,18.0343597124917));
#53473=CARTESIAN_POINT('Ctrl Pts',(7.40358438374929,-32.2208437341878,18.4775776951444));
#53474=CARTESIAN_POINT('Ctrl Pts',(7.40358438374929,-41.9520702046485,1.50845259553232));
#53475=CARTESIAN_POINT('Ctrl Pts',(7.40358438374929,-33.4647012075554,-16.1157507275363));
#53476=CARTESIAN_POINT('Ctrl Pts',(7.40358438374929,-17.3489504800191,-49.5804519350917));
#53477=CARTESIAN_POINT('Ctrl Pts',(7.40358438374929,16.1157507275363,-33.4647012075554));
#53478=CARTESIAN_POINT('Ctrl Pts',(7.40358438374929,49.5804519350917,-17.3489504800191));
#53479=CARTESIAN_POINT('Ctrl Pts',(7.40358438374929,33.4647012075554,16.1157507275363));
#53480=CARTESIAN_POINT('Ctrl Pts',(7.40358438374929,17.3489504800191,49.5804519350917));
#53481=CARTESIAN_POINT('Ctrl Pts',(7.40358438374929,-16.1157507275363,33.4647012075554));
#53482=CARTESIAN_POINT('Ctrl Pts',(7.40358438374929,-26.4917322357228,28.4678918679965));
#53483=CARTESIAN_POINT('Ctrl Pts',(7.40358438374929,-32.2208437341878,18.4775776951444));
#53484=CARTESIAN_POINT('Ctrl Pts',(6.82198164612729,-32.8553406354367,18.8414404756127));
#53485=CARTESIAN_POINT('Ctrl Pts',(6.82198164612729,-42.778195639644,1.53815723348166));
#53486=CARTESIAN_POINT('Ctrl Pts',(6.82198164612729,-34.1236923063789,-16.4331041147498));
#53487=CARTESIAN_POINT('Ctrl Pts',(6.82198164612729,-17.6905881916291,-50.5567964211288));
#53488=CARTESIAN_POINT('Ctrl Pts',(6.82198164612729,16.4331041147498,-34.1236923063789));
#53489=CARTESIAN_POINT('Ctrl Pts',(6.82198164612729,50.5567964211288,-17.6905881916291));
#53490=CARTESIAN_POINT('Ctrl Pts',(6.82198164612729,34.1236923063789,16.4331041147498));
#53491=CARTESIAN_POINT('Ctrl Pts',(6.82198164612729,17.6905881916291,50.5567964211288));
#53492=CARTESIAN_POINT('Ctrl Pts',(6.82198164612729,-16.4331041147498,34.1236923063789));
#53493=CARTESIAN_POINT('Ctrl Pts',(6.82198164612729,-27.013410753857,29.0284851697842));
#53494=CARTESIAN_POINT('Ctrl Pts',(6.82198164612729,-32.8553406354367,18.8414404756127));
#53495=CARTESIAN_POINT('Ctrl Pts',(6.40395249919757,-33.3400992359811,19.1194333419337));
#53496=CARTESIAN_POINT('Ctrl Pts',(6.40395249919757,-43.4093593363527,1.56085171582452));
#53497=CARTESIAN_POINT('Ctrl Pts',(6.40395249919757,-34.627164588447,-16.6755635870669));
#53498=CARTESIAN_POINT('Ctrl Pts',(6.40395249919757,-17.9516010013801,-51.3027281755139));
#53499=CARTESIAN_POINT('Ctrl Pts',(6.40395249919757,16.6755635870669,-34.627164588447));
#53500=CARTESIAN_POINT('Ctrl Pts',(6.40395249919757,51.3027281755139,-17.9516010013801));
#53501=CARTESIAN_POINT('Ctrl Pts',(6.40395249919757,34.627164588447,16.6755635870669));
#53502=CARTESIAN_POINT('Ctrl Pts',(6.40395249919757,17.9516010013801,51.3027281755139));
#53503=CARTESIAN_POINT('Ctrl Pts',(6.40395249919757,-16.6755635870669,34.627164588447));
#53504=CARTESIAN_POINT('Ctrl Pts',(6.40395249919757,-27.4119755819704,29.4567810746408));
#53505=CARTESIAN_POINT('Ctrl Pts',(6.40395249919757,-33.3400992359811,19.1194333419337));
#53506=CARTESIAN_POINT('Ctrl Pts',(6.13331019225912,-33.6672049264476,19.3070175299823));
#53507=CARTESIAN_POINT('Ctrl Pts',(6.13331019225912,-43.835256342775,1.57616551182155));
#53508=CARTESIAN_POINT('Ctrl Pts',(6.13331019225912,-34.9668979078181,-16.8391705308393));
#53509=CARTESIAN_POINT('Ctrl Pts',(6.13331019225912,-18.1277273769788,-51.8060684386574));
#53510=CARTESIAN_POINT('Ctrl Pts',(6.13331019225912,16.8391705308393,-34.9668979078181));
#53511=CARTESIAN_POINT('Ctrl Pts',(6.13331019225912,51.8060684386574,-18.1277273769788));
#53512=CARTESIAN_POINT('Ctrl Pts',(6.13331019225912,34.9668979078181,16.8391705308393));
#53513=CARTESIAN_POINT('Ctrl Pts',(6.13331019225912,18.1277273769788,51.8060684386574));
#53514=CARTESIAN_POINT('Ctrl Pts',(6.13331019225912,-16.8391705308393,34.9668979078181));
#53515=CARTESIAN_POINT('Ctrl Pts',(6.13331019225912,-27.6809193885357,29.745786834466));
#53516=CARTESIAN_POINT('Ctrl Pts',(6.13331019225912,-33.6672049264476,19.3070175299823));
#53517=CARTESIAN_POINT('Ctrl Pts',(6.,-33.8317410921456,19.4013735254499));
#53518=CARTESIAN_POINT('Ctrl Pts',(6.,-44.0494851454566,1.58386844499903));
#53519=CARTESIAN_POINT('Ctrl Pts',(6.,-35.1377858481943,-16.9214658255848));
#53520=CARTESIAN_POINT('Ctrl Pts',(6.,-18.2163200226096,-52.0592516737791));
#53521=CARTESIAN_POINT('Ctrl Pts',(6.,16.9214658255848,-35.1377858481943));
#53522=CARTESIAN_POINT('Ctrl Pts',(6.,52.0592516737791,-18.2163200226096));
#53523=CARTESIAN_POINT('Ctrl Pts',(6.,35.1377858481943,16.9214658255848));
#53524=CARTESIAN_POINT('Ctrl Pts',(6.,18.2163200226096,52.0592516737791));
#53525=CARTESIAN_POINT('Ctrl Pts',(6.,-16.9214658255848,35.1377858481943));
#53526=CARTESIAN_POINT('Ctrl Pts',(6.,-27.8161997704128,29.8911585017043));
#53527=CARTESIAN_POINT('Ctrl Pts',(6.,-33.8317410921456,19.4013735254499));
#53528=CARTESIAN_POINT('Ctrl Pts',(24.5,-23.4219747427337,13.431719888039));
#53529=CARTESIAN_POINT('Ctrl Pts',(23.5178991898112,-25.0276360494611,10.9685861831122));
#53530=CARTESIAN_POINT('Ctrl Pts',(22.3947886245986,-26.2729301477538,8.34676959442289));
#53531=CARTESIAN_POINT('Ctrl Pts',(21.1743874927566,-27.2201735658818,5.66613862859487));
#53532=CARTESIAN_POINT('Ctrl Pts',(20.5031871793434,-27.7411416824604,4.19183620665813));
#53533=CARTESIAN_POINT('Ctrl Pts',(19.8411792966408,-28.1598441640515,2.68270023879079));
#53534=CARTESIAN_POINT('Ctrl Pts',(19.1295827650261,-28.508103594306,1.18344085144545));
#53535=CARTESIAN_POINT('Ctrl Pts',(18.8261415870913,-28.6566094498694,0.544122060088292));
#53536=CARTESIAN_POINT('Ctrl Pts',(18.5104994276271,-28.7937513256439,-0.0985692732500806));
#53537=CARTESIAN_POINT('Ctrl Pts',(18.2016639423759,-28.9165522468366,-0.697094034628921));
#53538=CARTESIAN_POINT('Ctrl Pts',(17.6747132403633,-29.1260813803741,-1.718327209709));
#53539=CARTESIAN_POINT('Ctrl Pts',(17.2016343370993,-29.2779074067587,-2.63744809926651));
#53540=CARTESIAN_POINT('Ctrl Pts',(16.872935292646,-29.3776496099841,-3.25480188360693));
#53541=CARTESIAN_POINT('Ctrl Pts',(16.6342454025477,-29.4500789520458,-3.703102873289));
#53542=CARTESIAN_POINT('Ctrl Pts',(16.5014949770664,-29.4875609766571,-3.94561707113168));
#53543=CARTESIAN_POINT('Ctrl Pts',(16.3424569562979,-29.5324155816376,-4.23265760880312));
#53544=CARTESIAN_POINT('Ctrl Pts',(15.993118510103,-29.6309419461689,-4.86316278574444));
#53545=CARTESIAN_POINT('Ctrl Pts',(15.6312480487537,-29.7273563920893,-5.48745018218933));
#53546=CARTESIAN_POINT('Ctrl Pts',(15.2503296894305,-29.8330034119802,-6.09818239131044));
#53547=CARTESIAN_POINT('Ctrl Pts',(14.7484414179076,-29.9722012188248,-6.90286750374191));
#53548=CARTESIAN_POINT('Ctrl Pts',(14.2669345517206,-30.0952138942946,-7.68104629603547));
#53549=CARTESIAN_POINT('Ctrl Pts',(13.7912435751455,-30.2282988102454,-8.40145711329548));
#53550=CARTESIAN_POINT('Ctrl Pts',(13.5533980868579,-30.2948412682208,-8.76166252192548));
#53551=CARTESIAN_POINT('Ctrl Pts',(13.3161115657262,-30.3641806660347,-9.10948527341258));
#53552=CARTESIAN_POINT('Ctrl Pts',(13.0766514227367,-30.440228178246,-9.44459923238964));
#53553=CARTESIAN_POINT('Ctrl Pts',(12.9188702359555,-30.4903361694075,-9.66540707746248));
#53554=CARTESIAN_POINT('Ctrl Pts',(12.7601526360409,-30.5433595566134,-9.88070391694664));
#53555=CARTESIAN_POINT('Ctrl Pts',(12.5997389313808,-30.6005375280091,-10.0903988646281));
#53556=CARTESIAN_POINT('Ctrl Pts',(12.5166971934814,-30.6301369822723,-10.1989521389328));
#53557=CARTESIAN_POINT('Ctrl Pts',(12.4397215765388,-30.6583559714772,-10.29784186772));
#53558=CARTESIAN_POINT('Ctrl Pts',(12.3478597934844,-30.6933593253107,-10.4131461873135));
#53559=CARTESIAN_POINT('Ctrl Pts',(11.9116121727781,-30.8595887334372,-10.9607213965826));
#53560=CARTESIAN_POINT('Ctrl Pts',(10.7144663992386,-31.2847896561702,-12.5314661716072));
#53561=CARTESIAN_POINT('Ctrl Pts',(9.56604185022482,-32.0598213250961,-13.5737242681804));
#53562=CARTESIAN_POINT('Ctrl Pts',(9.07284645450724,-32.3926616940849,-14.0213260673763));
#53563=CARTESIAN_POINT('Ctrl Pts',(8.57333454992668,-32.7892957869518,-14.4000170895921));
#53564=CARTESIAN_POINT('Ctrl Pts',(8.00348148262884,-33.3155434735552,-14.8086408410792));
#53565=CARTESIAN_POINT('Ctrl Pts',(7.63919428965855,-33.6519552673337,-15.0698597551337));
#53566=CARTESIAN_POINT('Ctrl Pts',(7.24388644384666,-34.0525400988056,-15.3432535750814));
#53567=CARTESIAN_POINT('Ctrl Pts',(6.94254646282606,-34.3778179503946,-15.5540684672922));
#53568=CARTESIAN_POINT('Ctrl Pts',(6.91433564865313,-34.4082697775789,-15.5738045133651));
#53569=CARTESIAN_POINT('Ctrl Pts',(6.88669635040576,-34.4382827302419,-15.5931590893644));
#53570=CARTESIAN_POINT('Ctrl Pts',(6.85962514029878,-34.4678401502989,-15.6121377164754));
#53571=CARTESIAN_POINT('Ctrl Pts',(6.44000062073739,-34.9260028309428,-15.9063209928014));
#53572=CARTESIAN_POINT('Ctrl Pts',(6.15412442492902,-35.2918397798349,-16.0757548327879));
#53573=CARTESIAN_POINT('Ctrl Pts',(6.,-35.4893251315053,-16.1712028529206));
#53574=CARTESIAN_POINT('Ctrl Pts',(2.09999999999999,-9.13041565192885,-3.39805179937466));
#53575=CARTESIAN_POINT('Ctrl Pts',(2.73333333333332,-9.13041565192885,-3.39805179937466));
#53576=CARTESIAN_POINT('Ctrl Pts',(3.36701317451252,-9.13040108347824,-3.39810652799444));
#53577=CARTESIAN_POINT('Ctrl Pts',(4.12582101723434,-9.13039676871029,-3.39812307912054));
#53578=CARTESIAN_POINT('Ctrl Pts',(4.3827813081152,-9.12995863034688,-3.39933937508568));
#53579=CARTESIAN_POINT('Ctrl Pts',(4.88874880886513,-9.12802340460705,-3.40473249825757));
#53580=CARTESIAN_POINT('Ctrl Pts',(5.76579688899393,-9.12357463561424,-3.4171742341258));
#53581=CARTESIAN_POINT('Ctrl Pts',(6.49301772180469,-9.12367746676099,-3.41699407326797));
#53582=CARTESIAN_POINT('Ctrl Pts',(7.02339624162716,-9.13084124181946,-3.39664052379125));
#53583=CARTESIAN_POINT('Ctrl Pts',(7.1498562830745,-9.13266683983108,-3.3916514191029));
#53584=CARTESIAN_POINT('Ctrl Pts',(7.33704059907056,-9.13564437529334,-3.38374208606773));
#53585=CARTESIAN_POINT('Ctrl Pts',(7.52531480017061,-9.13893394226214,-3.37518464965992));
#53586=CARTESIAN_POINT('Ctrl Pts',(7.90079264373577,-9.14610157643292,-3.35670170902175));
#53587=CARTESIAN_POINT('Ctrl Pts',(8.46123456943149,-9.15912772542386,-3.32321177104627));
#53588=CARTESIAN_POINT('Ctrl Pts',(9.06500753118942,-9.177875904121,-3.27146172501592));
#53589=CARTESIAN_POINT('Ctrl Pts',(9.52838216794511,-9.19546305542652,-3.21908622722073));
#53590=CARTESIAN_POINT('Ctrl Pts',(9.75197533530386,-9.20509907063539,-3.18893300462712));
#53591=CARTESIAN_POINT('Ctrl Pts',(10.3692809660311,-9.23340523376178,-3.09795413997167));
#53592=CARTESIAN_POINT('Ctrl Pts',(11.3477650727983,-9.30172686747984,-2.89373436722122));
#53593=CARTESIAN_POINT('Ctrl Pts',(12.2736167934301,-9.38175751450599,-2.62467429855293));
#53594=CARTESIAN_POINT('Ctrl Pts',(13.0004869538322,-9.43659420895444,-2.40131121191103));
#53595=CARTESIAN_POINT('Ctrl Pts',(13.5002202963651,-9.47692561134844,-2.23041445466345));
#53596=CARTESIAN_POINT('Ctrl Pts',(14.4706182485369,-9.56220626799283,-1.84447625067277));
#53597=CARTESIAN_POINT('Ctrl Pts',(15.1515663737436,-9.61926188953974,-1.52559606535566));
#53598=CARTESIAN_POINT('Ctrl Pts',(15.884389511088,-9.66262454675229,-1.17518401443769));
#53599=CARTESIAN_POINT('Ctrl Pts',(16.3868780638063,-9.68960774126478,-0.916464713226361));
#53600=CARTESIAN_POINT('Ctrl Pts',(17.3638496496076,-9.73087588269211,-0.357244332963071));
#53601=CARTESIAN_POINT('Ctrl Pts',(18.0499776434112,-9.73673515107644,0.0836392175228933));
#53602=CARTESIAN_POINT('Ctrl Pts',(18.7841567244697,-9.71419302093459,0.55803484097089));
#53603=CARTESIAN_POINT('Ctrl Pts',(19.2877100748509,-9.68849014881372,0.901898771721124));
#53604=CARTESIAN_POINT('Ctrl Pts',(20.2708126431919,-9.60110184256547,1.62625821337173));
#53605=CARTESIAN_POINT('Ctrl Pts',(20.968566991788,-9.48879837203063,2.17915797653068));
#53606=CARTESIAN_POINT('Ctrl Pts',(22.6570657765617,-9.12376585269189,3.49147880528747));
#53607=CARTESIAN_POINT('Ctrl Pts',(23.7241254823866,-8.71518052183065,4.38549881588758));
#53608=CARTESIAN_POINT('Ctrl Pts',(24.6950729185821,-8.16338858110383,5.27047024423429));
#53609=CARTESIAN_POINT('Ctrl Pts',(2.09999999999999,-12.9002177548493,-5.21349281006839));
#53610=CARTESIAN_POINT('Ctrl Pts',(2.73333333333332,-12.9002177548493,-5.21349281006839));
#53611=CARTESIAN_POINT('Ctrl Pts',(3.36720848131827,-12.9001975910235,-5.21355448519127));
#53612=CARTESIAN_POINT('Ctrl Pts',(4.12623507204341,-12.9001917132969,-5.21357280295523));
#53613=CARTESIAN_POINT('Ctrl Pts',(4.38604826009982,-12.8995138670331,-5.21530251739604));
#53614=CARTESIAN_POINT('Ctrl Pts',(4.89390545898918,-12.8965300720384,-5.2229435076951));
#53615=CARTESIAN_POINT('Ctrl Pts',(5.77024592040542,-12.8896918237525,-5.24051394682823));
#53616=CARTESIAN_POINT('Ctrl Pts',(6.48768609145402,-12.8898924702624,-5.24012227121644));
#53617=CARTESIAN_POINT('Ctrl Pts',(7.00642437533162,-12.900756463832,-5.21179807239735));
#53618=CARTESIAN_POINT('Ctrl Pts',(7.13273638677672,-12.9035579301272,-5.20475518479158));
#53619=CARTESIAN_POINT('Ctrl Pts',(7.3183164241747,-12.9080992926691,-5.19364592987697));
#53620=CARTESIAN_POINT('Ctrl Pts',(7.50524686034319,-12.9131151672861,-5.18161674063603));
#53621=CARTESIAN_POINT('Ctrl Pts',(7.87735507332389,-12.9240283057097,-5.15566801581097));
#53622=CARTESIAN_POINT('Ctrl Pts',(8.4315346972579,-12.9438386062717,-5.10870296150625));
#53623=CARTESIAN_POINT('Ctrl Pts',(9.02545493458829,-12.9723788727574,-5.03636407240455));
#53624=CARTESIAN_POINT('Ctrl Pts',(9.47896581078012,-12.99918743678,-4.96340069318231));
#53625=CARTESIAN_POINT('Ctrl Pts',(9.69688367867189,-13.0138864528649,-4.92150249520299));
#53626=CARTESIAN_POINT('Ctrl Pts',(10.2969185301416,-13.0570771398965,-4.79527718202436));
#53627=CARTESIAN_POINT('Ctrl Pts',(11.2522144952412,-13.1613303391514,-4.51147447372354));
#53628=CARTESIAN_POINT('Ctrl Pts',(12.16830830149,-13.2859456545432,-4.13360457116113));
#53629=CARTESIAN_POINT('Ctrl Pts',(12.8911660496029,-13.3731353575996,-3.81822327297548));
#53630=CARTESIAN_POINT('Ctrl Pts',(13.3786040775802,-13.4368505094726,-3.58035741471442));
#53631=CARTESIAN_POINT('Ctrl Pts',(14.3384175365999,-13.574070267889,-3.03828527802715));
#53632=CARTESIAN_POINT('Ctrl Pts',(15.0146631063079,-13.6690362785393,-2.58739886270306));
#53633=CARTESIAN_POINT('Ctrl Pts',(15.7460539088381,-13.7458705357116,-2.0894399940261));
#53634=CARTESIAN_POINT('Ctrl Pts',(16.2427389372309,-13.7954928643336,-1.7249477173051));
#53635=CARTESIAN_POINT('Ctrl Pts',(17.2171500502893,-13.8792388914454,-0.931039998810538));
#53636=CARTESIAN_POINT('Ctrl Pts',(17.901657841902,-13.9071495118269,-0.302213557964748));
#53637=CARTESIAN_POINT('Ctrl Pts',(18.6350521995774,-13.89566421944,0.376020800248144));
#53638=CARTESIAN_POINT('Ctrl Pts',(19.138387973248,-13.8747909549584,0.867348303200731));
#53639=CARTESIAN_POINT('Ctrl Pts',(20.1238445925502,-13.782576518031,1.90675272254023));
#53640=CARTESIAN_POINT('Ctrl Pts',(20.822005894914,-13.6464379916399,2.70212764346435));
#53641=CARTESIAN_POINT('Ctrl Pts',(22.5097447039609,-13.1821252157743,4.59209198679041));
#53642=CARTESIAN_POINT('Ctrl Pts',(23.5814142719248,-12.6388162011058,5.8901716529331));
#53643=CARTESIAN_POINT('Ctrl Pts',(24.5630597774301,-11.882904360092,7.18919796098686));
#53644=CARTESIAN_POINT('Ctrl Pts',(2.09999999999999,-21.6964226616636,-9.44952183502042));
#53645=CARTESIAN_POINT('Ctrl Pts',(2.73333333333332,-21.6964226616636,-9.44952183502042));
#53646=CARTESIAN_POINT('Ctrl Pts',(3.36768851389112,-21.6963695414677,-9.44970316559896));
#53647=CARTESIAN_POINT('Ctrl Pts',(4.12723220823948,-21.6963540844379,-9.44975722375134));
#53648=CARTESIAN_POINT('Ctrl Pts',(4.39370635937899,-21.6950981950085,-9.45272881112924));
#53649=CARTESIAN_POINT('Ctrl Pts',(4.90596400000984,-21.6896305544311,-9.46570382276018));
#53650=CARTESIAN_POINT('Ctrl Pts',(5.78069669373953,-21.6772192778768,-9.49525285207215));
#53651=CARTESIAN_POINT('Ctrl Pts',(6.47525361359603,-21.677778366334,-9.49418418263408));
#53652=CARTESIAN_POINT('Ctrl Pts',(6.96710249362278,-21.6966497719658,-9.44860121784704));
#53653=CARTESIAN_POINT('Ctrl Pts',(7.09307430585892,-21.7017191773118,-9.43678759087601));
#53654=CARTESIAN_POINT('Ctrl Pts',(7.27495509380485,-21.7098167389422,-9.4184111745766));
#53655=CARTESIAN_POINT('Ctrl Pts',(7.45879739148957,-21.7187736697537,-9.39847144082777));
#53656=CARTESIAN_POINT('Ctrl Pts',(7.823170843205,-21.7381987850423,-9.35559078117172));
#53657=CARTESIAN_POINT('Ctrl Pts',(8.36310684327955,-21.7733135823236,-9.27838002203018));
#53658=CARTESIAN_POINT('Ctrl Pts',(8.93508744882405,-21.823600521285,-9.16047238005773));
#53659=CARTESIAN_POINT('Ctrl Pts',(9.36757815131443,-21.87052047451,-9.04266937137984));
#53660=CARTESIAN_POINT('Ctrl Pts',(9.57392762477484,-21.8961119122116,-8.97550203198768));
#53661=CARTESIAN_POINT('Ctrl Pts',(10.140021954483,-21.9710011903251,-8.77426004522114));
#53662=CARTESIAN_POINT('Ctrl Pts',(11.0614193925012,-22.1545360362948,-8.31703872507497));
#53663=CARTESIAN_POINT('Ctrl Pts',(11.9722628052669,-22.3833575412528,-7.68838929295787));
#53664=CARTESIAN_POINT('Ctrl Pts',(12.6924971605734,-22.5463694958218,-7.16015059826062));
#53665=CARTESIAN_POINT('Ctrl Pts',(13.1758960402558,-22.6651639298491,-6.76712693131451));
#53666=CARTESIAN_POINT('Ctrl Pts',(14.142076411012,-22.9274558453913,-5.85324663451816));
#53667=CARTESIAN_POINT('Ctrl Pts',(14.8238713096107,-23.1131579009961,-5.08951620479052));
#53668=CARTESIAN_POINT('Ctrl Pts',(15.5572563628566,-23.269163089777,-4.24668378099617));
#53669=CARTESIAN_POINT('Ctrl Pts',(16.0655853887807,-23.3748818615298,-3.62213679367982));
#53670=CARTESIAN_POINT('Ctrl Pts',(17.0554277769773,-23.5604115991072,-2.2604717975477));
#53671=CARTESIAN_POINT('Ctrl Pts',(17.749227444809,-23.639780747396,-1.18295910400568));
#53672=CARTESIAN_POINT('Ctrl Pts',(18.4856283652679,-23.6530822724334,-0.0267264997289242));
#53673=CARTESIAN_POINT('Ctrl Pts',(19.0039954021354,-23.642532945262,0.828874446381748));
#53674=CARTESIAN_POINT('Ctrl Pts',(20.0037042032201,-23.5329875501118,2.62392419000413));
#53675=CARTESIAN_POINT('Ctrl Pts',(20.7092095322358,-23.3355002606907,3.994145223667));
#53676=CARTESIAN_POINT('Ctrl Pts',(22.4031068849489,-22.6280521158487,7.2370377336757));
#53677=CARTESIAN_POINT('Ctrl Pts',(23.504475912352,-21.746935009538,9.5200949784719));
#53678=CARTESIAN_POINT('Ctrl Pts',(24.5018373925611,-20.4887878955378,11.7966817146722));
#53679=CARTESIAN_POINT('Ctrl Pts',(2.09999999999999,-30.492627568478,-13.6855508599725));
#53680=CARTESIAN_POINT('Ctrl Pts',(2.73333333333332,-30.492627568478,-13.6855508599725));
#53681=CARTESIAN_POINT('Ctrl Pts',(3.36822682214226,-30.4925870569924,-13.6857046438341));
#53682=CARTESIAN_POINT('Ctrl Pts',(4.12830119635636,-30.4925765273047,-13.6857478663648));
#53683=CARTESIAN_POINT('Ctrl Pts',(4.40145272754258,-30.4907070441319,-13.6900312837157));
#53684=CARTESIAN_POINT('Ctrl Pts',(4.91805056385413,-30.4826845293831,-13.7084761779709));
#53685=CARTESIAN_POINT('Ctrl Pts',(5.791384213593,-30.4647401208151,-13.7499098195501));
#53686=CARTESIAN_POINT('Ctrl Pts',(6.46263952973601,-30.4660585960359,-13.7472501476117));
#53687=CARTESIAN_POINT('Ctrl Pts',(6.92897284878534,-30.4916153574711,-13.6871363494999));
#53688=CARTESIAN_POINT('Ctrl Pts',(7.05462978588519,-30.4989350691117,-13.6705906736548));
#53689=CARTESIAN_POINT('Ctrl Pts',(7.2330357976122,-30.5103941645259,-13.64535449053));
#53690=CARTESIAN_POINT('Ctrl Pts',(7.41402545512323,-30.5231160748026,-13.6178741235955));
#53691=CARTESIAN_POINT('Ctrl Pts',(7.77131680307424,-30.550583615613,-13.5590581898128));
#53692=CARTESIAN_POINT('Ctrl Pts',(8.29875758008135,-30.6000551322046,-13.4535786484538));
#53693=CARTESIAN_POINT('Ctrl Pts',(8.85376435941124,-30.6702769361216,-13.2940463367281));
#53694=CARTESIAN_POINT('Ctrl Pts',(9.27339243591186,-30.7356605585286,-13.1351572273555));
#53695=CARTESIAN_POINT('Ctrl Pts',(9.4742240152269,-30.7714246498893,-13.0444339073219));
#53696=CARTESIAN_POINT('Ctrl Pts',(10.0273297328825,-30.8765426957254,-12.7717645325826));
#53697=CARTESIAN_POINT('Ctrl Pts',(10.9572339063684,-31.1445192227213,-12.1307089623794));
#53698=CARTESIAN_POINT('Ctrl Pts',(11.8781426048001,-31.4831753576899,-11.2362716678478));
#53699=CARTESIAN_POINT('Ctrl Pts',(12.6020626440135,-31.7238287379969,-10.4893969835164));
#53700=CARTESIAN_POINT('Ctrl Pts',(13.0988736704966,-31.9043633305436,-9.92073242692073));
#53701=CARTESIAN_POINT('Ctrl Pts',(14.0796979680275,-32.2976015767017,-8.60937463783709));
#53702=CARTESIAN_POINT('Ctrl Pts',(14.767676431986,-32.5746344119006,-7.51992611358519));
#53703=CARTESIAN_POINT('Ctrl Pts',(15.5027273811337,-32.8079808305111,-6.32795870904283));
#53704=CARTESIAN_POINT('Ctrl Pts',(16.0202991032636,-32.9710575408164,-5.42474240090243));
#53705=CARTESIAN_POINT('Ctrl Pts',(17.0170548288356,-33.2543208336152,-3.48039388031436));
#53706=CARTESIAN_POINT('Ctrl Pts',(17.7141669052032,-33.3803196556765,-1.94722345366041));
#53707=CARTESIAN_POINT('Ctrl Pts',(18.451391136466,-33.4127835371598,-0.311140673056842));
#53708=CARTESIAN_POINT('Ctrl Pts',(18.9741597084201,-33.4081197665559,0.916672237872836));
#53709=CARTESIAN_POINT('Ctrl Pts',(19.9767059515643,-33.2711886970384,3.47029956120117));
#53710=CARTESIAN_POINT('Ctrl Pts',(20.683600748323,-33.0046898829411,5.4153715482179));
#53711=CARTESIAN_POINT('Ctrl Pts',(22.3785099788158,-32.036142933647,10.0079986575605));
#53712=CARTESIAN_POINT('Ctrl Pts',(23.4839952293235,-30.8044868476372,13.2681438080948));
#53713=CARTESIAN_POINT('Ctrl Pts',(24.4831092917558,-29.0356277561782,16.5096970084821));
#53714=CARTESIAN_POINT('Ctrl Pts',(2.09999999999999,-35.5190303723719,-16.1061388742308));
#53715=CARTESIAN_POINT('Ctrl Pts',(2.73333333333332,-35.5190303723719,-16.1061388742308));
#53716=CARTESIAN_POINT('Ctrl Pts',(3.3685529499539,-35.5189963826913,-16.1062755303871));
#53717=CARTESIAN_POINT('Ctrl Pts',(4.12893389176798,-35.5189883555912,-16.1063123113306));
#53718=CARTESIAN_POINT('Ctrl Pts',(4.40590876805926,-35.5167560554967,-16.1113705287801));
#53719=CARTESIAN_POINT('Ctrl Pts',(4.92495106442005,-35.5072455660771,-16.1329983700014));
#53720=CARTESIAN_POINT('Ctrl Pts',(5.79759451343229,-35.4861563499845,-16.181187912636));
#53721=CARTESIAN_POINT('Ctrl Pts',(6.4552933171533,-35.4879918202634,-16.1774408228987));
#53722=CARTESIAN_POINT('Ctrl Pts',(6.90777589770066,-35.5169934210011,-16.1098049933539));
#53723=CARTESIAN_POINT('Ctrl Pts',(7.03326597379373,-35.5255942090726,-16.090566148091));
#53724=CARTESIAN_POINT('Ctrl Pts',(7.20980469627123,-35.5389211123446,-16.0615220192229));
#53725=CARTESIAN_POINT('Ctrl Pts',(7.38928547178791,-35.5537484109996,-16.0298305624976));
#53726=CARTESIAN_POINT('Ctrl Pts',(7.74286592221491,-35.5856960588913,-15.9621555487075));
#53727=CARTESIAN_POINT('Ctrl Pts',(8.26401794171908,-35.6431524329166,-15.840991390971));
#53728=CARTESIAN_POINT('Ctrl Pts',(8.81152408908925,-35.7245572865462,-15.6581486065571));
#53729=CARTESIAN_POINT('Ctrl Pts',(9.22661397401185,-35.8006503185216,-15.4754672744663));
#53730=CARTESIAN_POINT('Ctrl Pts',(9.42598140904611,-35.8424916660102,-15.3707139312043));
#53731=CARTESIAN_POINT('Ctrl Pts',(9.976710666656,-35.9660011697121,-15.0547620286962));
#53732=CARTESIAN_POINT('Ctrl Pts',(10.9140166500484,-36.2852504824252,-14.301418631492));
#53733=CARTESIAN_POINT('Ctrl Pts',(11.8387266298368,-36.6869798302323,-13.2531154851079));
#53734=CARTESIAN_POINT('Ctrl Pts',(12.5644537233057,-36.9720369099943,-12.380341222988));
#53735=CARTESIAN_POINT('Ctrl Pts',(13.0663236803827,-37.1882014264798,-11.7094275168349));
#53736=CARTESIAN_POINT('Ctrl Pts',(14.0520240221945,-37.65549414411,-10.1712590536084));
#53737=CARTESIAN_POINT('Ctrl Pts',(14.7426139091248,-37.9842005172013,-8.89575090186054));
#53738=CARTESIAN_POINT('Ctrl Pts',(15.4784727169398,-38.2612735354973,-7.50405020937324));
#53739=CARTESIAN_POINT('Ctrl Pts',(15.9995906107788,-38.456495327364,-6.44277625931302));
#53740=CARTESIAN_POINT('Ctrl Pts',(16.9994487463634,-38.7947103989691,-4.16721681261721));
#53741=CARTESIAN_POINT('Ctrl Pts',(17.6981454111525,-38.9468546317636,-2.37398192696008));
#53742=CARTESIAN_POINT('Ctrl Pts',(18.4357121346094,-38.9897987920051,-0.463585233612633));
#53743=CARTESIAN_POINT('Ctrl Pts',(18.9608308592025,-38.9881432373632,0.975716140749977));
#53744=CARTESIAN_POINT('Ctrl Pts',(19.9653528594919,-38.8351271359227,3.96186424955774));
#53745=CARTESIAN_POINT('Ctrl Pts',(20.6729531153352,-38.5287766299084,6.23514955400077));
#53746=CARTESIAN_POINT('Ctrl Pts',(22.3680492077458,-37.4100161862565,11.5988469917284));
#53747=CARTESIAN_POINT('Ctrl Pts',(23.4757593035169,-35.9774143267865,15.4158344467734));
#53748=CARTESIAN_POINT('Ctrl Pts',(24.4767076204831,-33.9162528966534,19.2087170933586));
#53749=CARTESIAN_POINT('',(3.2,-34.2572188230213,-15.4984824583453));
#53750=CARTESIAN_POINT('Ctrl Pts',(3.2,-34.2572188230213,-15.4984824583453));
#53751=CARTESIAN_POINT('Ctrl Pts',(3.45174020130992,-33.5567398379256,-15.1611495581151));
#53752=CARTESIAN_POINT('Ctrl Pts',(3.71840125360142,-32.8479951510644,-14.8198361057081));
#53753=CARTESIAN_POINT('Ctrl Pts',(4.,-32.1353158291841,-14.4766278329416));
#53754=CARTESIAN_POINT('Ctrl Pts',(4.62816481260912,-30.5455357665781,-13.7110301053043));
#53755=CARTESIAN_POINT('Ctrl Pts',(5.32582967254414,-28.9317001372407,-13.0007563214461));
#53756=CARTESIAN_POINT('Ctrl Pts',(6.03866108353657,-27.4700228811071,-12.2911204000068));
#53757=CARTESIAN_POINT('Ctrl Pts',(6.32798218217299,-26.8767632925494,-12.0030962736052));
#53758=CARTESIAN_POINT('Ctrl Pts',(6.61604116814955,-26.3158796257153,-11.717411134043));
#53759=CARTESIAN_POINT('Ctrl Pts',(6.89476148100327,-25.8006837185162,-11.4328824518093));
#53760=CARTESIAN_POINT('Ctrl Pts',(7.65522892841368,-24.3950103664284,-10.6565673046356));
#53761=CARTESIAN_POINT('Ctrl Pts',(8.35226709293656,-23.2781841584713,-9.99003821184204));
#53762=CARTESIAN_POINT('Ctrl Pts',(8.7892632371809,-22.6126816498706,-9.5632075888662));
#53763=CARTESIAN_POINT('Ctrl Pts',(8.99031957804211,-22.3064924512345,-9.36682827441841));
#53764=CARTESIAN_POINT('Ctrl Pts',(9.18275522061529,-22.0230827498019,-9.17790378245122));
#53765=CARTESIAN_POINT('Ctrl Pts',(9.37496045909766,-21.7488041106976,-8.9863600510071));
#53766=CARTESIAN_POINT('Ctrl Pts',(9.48075233189684,-21.5978381374038,-8.88093227894211));
#53767=CARTESIAN_POINT('Ctrl Pts',(9.58626090848609,-21.4500100268611,-8.77491379472231));
#53768=CARTESIAN_POINT('Ctrl Pts',(9.69257910363365,-21.3038773401306,-8.66672356115102));
#53769=CARTESIAN_POINT('Ctrl Pts',(10.0319880469606,-20.8373650867963,-8.32133834459649));
#53770=CARTESIAN_POINT('Ctrl Pts',(10.3788056742595,-20.3884564675231,-7.95278423285573));
#53771=CARTESIAN_POINT('Ctrl Pts',(10.7756849085126,-19.9045583626959,-7.52432563668368));
#53772=CARTESIAN_POINT('Ctrl Pts',(10.8890930405622,-19.7662846123093,-7.40189371064982));
#53773=CARTESIAN_POINT('Ctrl Pts',(11.0576203524086,-19.5630034060169,-7.21920703316946));
#53774=CARTESIAN_POINT('Ctrl Pts',(11.2725125496543,-19.3123908782387,-6.98620793040072));
#53775=CARTESIAN_POINT('Ctrl Pts',(11.5968279595885,-18.9341663278698,-6.63456556973203));
#53776=CARTESIAN_POINT('Ctrl Pts',(12.0255678845029,-18.4509663195227,-6.16660018051478));
#53777=CARTESIAN_POINT('Ctrl Pts',(12.532035905153,-17.9090112566991,-5.64334903954311));
#53778=CARTESIAN_POINT('Ctrl Pts',(13.0988763177203,-17.3024536481663,-5.05772491219147));
#53779=CARTESIAN_POINT('Ctrl Pts',(13.7495416918469,-16.6567125930623,-4.35710056287699));
#53780=CARTESIAN_POINT('Ctrl Pts',(14.4398764942141,-16.0137917956181,-3.63694865307657));
#53781=CARTESIAN_POINT('Ctrl Pts',(14.7901814038696,-15.6875467459813,-3.27151328919831));
#53782=CARTESIAN_POINT('Ctrl Pts',(15.1459546152778,-15.3661826765097,-2.90956453468361));
#53783=CARTESIAN_POINT('Ctrl Pts',(15.4570717747561,-15.0907170797824,-2.60751868956995));
#53784=CARTESIAN_POINT('Ctrl Pts',(15.7998231405479,-14.7872423062749,-2.27476100395055));
#53785=CARTESIAN_POINT('Ctrl Pts',(16.0676294492373,-14.5587589003322,-2.012820704421));
#53786=CARTESIAN_POINT('Ctrl Pts',(16.3615307970805,-14.3129125519894,-1.7268209695992));
#53787=CARTESIAN_POINT('Ctrl Pts',(17.029661602165,-13.754025973718,-1.07665303235506));
#53788=CARTESIAN_POINT('Ctrl Pts',(17.70846918735,-13.2157293141182,-0.418819875773385));
#53789=CARTESIAN_POINT('Ctrl Pts',(18.4207032016838,-12.6778667357551,0.201349018822154));
#53790=CARTESIAN_POINT('Ctrl Pts',(18.8298642042311,-12.368877853777,0.5576208642475));
#53791=CARTESIAN_POINT('Ctrl Pts',(19.2113759272833,-12.0893434047209,0.892739516924111));
#53792=CARTESIAN_POINT('Ctrl Pts',(19.5701113607632,-11.8294329222545,1.20481008177065));
#53793=CARTESIAN_POINT('Ctrl Pts',(20.1215476021955,-11.4299071264062,1.68451463080629));
#53794=CARTESIAN_POINT('Ctrl Pts',(20.6514912601791,-11.0507292363155,2.14929111120006));
#53795=CARTESIAN_POINT('Ctrl Pts',(21.3979544325339,-10.5292525052453,2.73212531702577));
#53796=CARTESIAN_POINT('Ctrl Pts',(21.8107631282044,-10.2408657004461,3.05444400227331));
#53797=CARTESIAN_POINT('Ctrl Pts',(22.3076315955317,-9.89607813725398,3.43397758799233));
#53798=CARTESIAN_POINT('Ctrl Pts',(22.8472772295076,-9.51040350637145,3.84215125052754));
#53799=CARTESIAN_POINT('Ctrl Pts',(23.3953136568588,-9.11873213256344,4.25667148690292));
#53800=CARTESIAN_POINT('Ctrl Pts',(23.9608264583105,-8.70201347485439,4.68200859429454));
#53801=CARTESIAN_POINT('Ctrl Pts',(24.5,-8.27152931289794,5.09374822578144));
#53802=CARTESIAN_POINT('Ctrl Pts',(2.7976100639101,-35.1047407419896,-15.9066763790287));
#53803=CARTESIAN_POINT('Ctrl Pts',(2.93206313032129,-34.8224775747036,-15.7707621775971));
#53804=CARTESIAN_POINT('Ctrl Pts',(3.06672198084968,-34.5398707717893,-15.6346853141056));
#53805=CARTESIAN_POINT('Ctrl Pts',(3.20143373635558,-34.2571954190233,-15.4985756754768));
#53806=CARTESIAN_POINT('Origin',(2.9,0.,0.));
#53807=CARTESIAN_POINT('Origin',(3.2,0.,0.));
#53808=CARTESIAN_POINT('Ctrl Pts',(2.1,-9.132050144933,3.39883892972008));
#53809=CARTESIAN_POINT('Ctrl Pts',(2.73333333333333,-9.132050144933,3.39883892972008));
#53810=CARTESIAN_POINT('Ctrl Pts',(3.3663079725943,-9.13201814031333,3.39888229101301));
#53811=CARTESIAN_POINT('Ctrl Pts',(4.12416251276081,-9.13200839072933,3.3988953533008));
#53812=CARTESIAN_POINT('Ctrl Pts',(4.36791120644981,-9.13244533410776,3.39775559897473));
#53813=CARTESIAN_POINT('Ctrl Pts',(4.86514190730704,-9.13445129820771,3.39254860847465));
#53814=CARTESIAN_POINT('Ctrl Pts',(5.74556055405348,-9.13920122500316,3.38025835485548));
#53815=CARTESIAN_POINT('Ctrl Pts',(6.51833360630206,-9.13927981015121,3.3800633150153));
#53816=CARTESIAN_POINT('Ctrl Pts',(7.10306547172688,-9.13061179056261,3.40220636614938));
#53817=CARTESIAN_POINT('Ctrl Pts',(7.2302207071034,-9.12871923506172,3.40720377175751));
#53818=CARTESIAN_POINT('Ctrl Pts',(7.42490086908427,-9.12567677829264,3.41546028383053));
#53819=CARTESIAN_POINT('Ctrl Pts',(7.61947075258487,-9.12244641117515,3.42440794243591));
#53820=CARTESIAN_POINT('Ctrl Pts',(8.01071766333096,-9.11546267897863,3.44392145121506));
#53821=CARTESIAN_POINT('Ctrl Pts',(8.60078557051619,-9.10263571479926,3.47975799428797));
#53822=CARTESIAN_POINT('Ctrl Pts',(9.2514949577206,-9.08139957335397,3.53513809773506));
#53823=CARTESIAN_POINT('Ctrl Pts',(9.76261946444148,-9.0583588320315,3.59140175594612));
#53824=CARTESIAN_POINT('Ctrl Pts',(10.0141181534512,-9.0444728354789,3.62401874784084));
#53825=CARTESIAN_POINT('Ctrl Pts',(10.7177011859537,-9.00131652348988,3.72332977624404));
#53826=CARTESIAN_POINT('Ctrl Pts',(11.8208115644903,-8.90749893786242,3.94890859650272));
#53827=CARTESIAN_POINT('Ctrl Pts',(12.8079858159913,-8.78130149362605,4.22216464532031));
#53828=CARTESIAN_POINT('Ctrl Pts',(13.5603938947108,-8.6716091455336,4.43282977440356));
#53829=CARTESIAN_POINT('Ctrl Pts',(14.1415289562624,-8.57605910539162,4.61236119395963));
#53830=CARTESIAN_POINT('Ctrl Pts',(15.2007183254417,-8.36507036120484,4.99040411635023));
#53831=CARTESIAN_POINT('Ctrl Pts',(15.9285075560867,-8.18274706597629,5.28485668422829));
#53832=CARTESIAN_POINT('Ctrl Pts',(16.6747842807949,-7.97783754058137,5.57956090150159));
#53833=CARTESIAN_POINT('Ctrl Pts',(17.2498051121831,-7.80376743378315,5.81968941516198));
#53834=CARTESIAN_POINT('Ctrl Pts',(18.2984823004268,-7.4319812814029,6.29489826615604));
#53835=CARTESIAN_POINT('Ctrl Pts',(19.0236998873884,-7.12174287391437,6.64228560049974));
#53836=CARTESIAN_POINT('Ctrl Pts',(19.7682368455845,-6.78029956366935,6.98103393296198));
#53837=CARTESIAN_POINT('Ctrl Pts',(20.3331957372982,-6.49893080008033,7.24492384682381));
#53838=CARTESIAN_POINT('Ctrl Pts',(21.3723377324311,-5.90855985872452,7.74330400682432));
#53839=CARTESIAN_POINT('Ctrl Pts',(22.0962735028998,-5.43125088344887,8.08178692215916));
#53840=CARTESIAN_POINT('Ctrl Pts',(23.2302665631601,-4.65052680131279,8.5566407190325));
#53841=CARTESIAN_POINT('Ctrl Pts',(23.8854423668127,-4.14620302888525,8.80675749744808));
#53842=CARTESIAN_POINT('Ctrl Pts',(24.5000000001022,-3.61603013990409,9.0160298461823));
#53843=CARTESIAN_POINT('Ctrl Pts',(2.1,-12.9016211606665,5.21416865468984));
#53844=CARTESIAN_POINT('Ctrl Pts',(2.73333333333333,-12.9016211606665,5.21416865468984));
#53845=CARTESIAN_POINT('Ctrl Pts',(3.3661091233326,-12.9015874618483,5.21422021700749));
#53846=CARTESIAN_POINT('Ctrl Pts',(4.12374360042828,-12.9015773813688,5.21423545286286));
#53847=CARTESIAN_POINT('Ctrl Pts',(4.36463922026465,-12.9022430853862,5.212636908042));
#53848=CARTESIAN_POINT('Ctrl Pts',(4.85997974089114,-12.9053085358418,5.20530291707169));
#53849=CARTESIAN_POINT('Ctrl Pts',(5.74110524153444,-12.9125858457571,5.18793249877815));
#53850=CARTESIAN_POINT('Ctrl Pts',(6.5236553961773,-12.912769153219,5.18752851193186));
#53851=CARTESIAN_POINT('Ctrl Pts',(7.12002561380569,-12.8993507043393,5.21924743609842));
#53852=CARTESIAN_POINT('Ctrl Pts',(7.24732883907975,-12.8964478351332,5.22631376259351));
#53853=CARTESIAN_POINT('Ctrl Pts',(7.44361306854449,-12.8917537205922,5.23804414925047));
#53854=CARTESIAN_POINT('Ctrl Pts',(7.63952655731801,-12.8867672451576,5.25074673477078));
#53855=CARTESIAN_POINT('Ctrl Pts',(8.03414277825582,-12.8759684345895,5.27847963617582));
#53856=CARTESIAN_POINT('Ctrl Pts',(8.6304721476858,-12.8561250346134,5.32946386238128));
#53857=CARTESIAN_POINT('Ctrl Pts',(9.29103328875621,-12.8233137230442,5.4084727122217));
#53858=CARTESIAN_POINT('Ctrl Pts',(9.8120207794755,-12.7877516418428,5.48896946217565));
#53859=CARTESIAN_POINT('Ctrl Pts',(10.0691942302806,-12.7663266344001,5.53572936280494));
#53860=CARTESIAN_POINT('Ctrl Pts',(10.790046981849,-12.6997688928597,5.67826660603544));
#53861=CARTESIAN_POINT('Ctrl Pts',(11.9163416059387,-12.5548183870822,6.00137237696006));
#53862=CARTESIAN_POINT('Ctrl Pts',(12.9132756635671,-12.3622653266479,6.38911209475131));
#53863=CARTESIAN_POINT('Ctrl Pts',(13.6696998405866,-12.1964669129034,6.68651744379352));
#53864=CARTESIAN_POINT('Ctrl Pts',(14.2631317779486,-12.0507099019981,6.94299161237581));
#53865=CARTESIAN_POINT('Ctrl Pts',(15.3329015938421,-11.7312148722742,7.47865016429502));
#53866=CARTESIAN_POINT('Ctrl Pts',(16.0654051873355,-11.4576547378963,7.89313324640987));
#53867=CARTESIAN_POINT('Ctrl Pts',(16.813125378213,-11.152369030053,8.30562093805636));
#53868=CARTESIAN_POINT('Ctrl Pts',(17.3939613704063,-10.8918326264795,8.64433036386289));
#53869=CARTESIAN_POINT('Ctrl Pts',(18.4451989758741,-10.3392458422533,9.30923518676035));
#53870=CARTESIAN_POINT('Ctrl Pts',(19.1720929876942,-9.88132720383576,9.79256593426711));
#53871=CARTESIAN_POINT('Ctrl Pts',(19.9174587712572,-9.3790868197873,10.2616497070843));
#53872=CARTESIAN_POINT('Ctrl Pts',(20.4827049382928,-8.96580926313345,10.6274510023226));
#53873=CARTESIAN_POINT('Ctrl Pts',(21.5194880485299,-8.10240134706929,11.3134235687948));
#53874=CARTESIAN_POINT('Ctrl Pts',(22.2433743515511,-7.40711512464527,11.7762751484356));
#53875=CARTESIAN_POINT('Ctrl Pts',(23.3781098890497,-6.27155818967328,12.4208354707857));
#53876=CARTESIAN_POINT('Ctrl Pts',(24.0312127056184,-5.54246593554869,12.7565226911889));
#53877=CARTESIAN_POINT('Ctrl Pts',(24.6419825553303,-4.77938339662506,13.0322784684415));
#53878=CARTESIAN_POINT('Ctrl Pts',(2.1,-21.6972868640446,9.4499380129526));
#53879=CARTESIAN_POINT('Ctrl Pts',(2.73333333333333,-21.6972868640446,9.4499380129526));
#53880=CARTESIAN_POINT('Ctrl Pts',(3.36562354525866,-21.6971828798135,9.45008587645688));
#53881=CARTESIAN_POINT('Ctrl Pts',(4.12273867778471,-21.697151611036,9.45012970586554));
#53882=CARTESIAN_POINT('Ctrl Pts',(4.35697313403335,-21.6983286095062,9.44750243336562));
#53883=CARTESIAN_POINT('Ctrl Pts',(4.84791259063805,-21.7038201038517,9.43528956102119));
#53884=CARTESIAN_POINT('Ctrl Pts',(5.7306447376668,-21.7169845344723,9.40607010718203));
#53885=CARTESIAN_POINT('Ctrl Pts',(6.53607333749491,-21.7174761488546,9.40495984396926));
#53886=CARTESIAN_POINT('Ctrl Pts',(7.15932985413337,-21.6923174381321,9.46034624187088));
#53887=CARTESIAN_POINT('Ctrl Pts',(7.28697322394794,-21.6870460982782,9.4722604919422));
#53888=CARTESIAN_POINT('Ctrl Pts',(7.48695635027016,-21.6784001614658,9.49229325078789));
#53889=CARTESIAN_POINT('Ctrl Pts',(7.68595777901539,-21.6692216654712,9.51394386312415));
#53890=CARTESIAN_POINT('Ctrl Pts',(8.0883081610984,-21.6492812399527,9.56133749836178));
#53891=CARTESIAN_POINT('Ctrl Pts',(8.69888136072734,-21.6124584984937,9.6488222621323));
#53892=CARTESIAN_POINT('Ctrl Pts',(9.381381730169,-21.5513928087426,9.78536670703229));
#53893=CARTESIAN_POINT('Ctrl Pts',(9.92338843691519,-21.4849895522994,9.92550005748472));
#53894=CARTESIAN_POINT('Ctrl Pts',(10.1921295368678,-21.4448781952111,10.0073116343241));
#53895=CARTESIAN_POINT('Ctrl Pts',(10.9469244149175,-21.3199576370334,10.257585612213));
#53896=CARTESIAN_POINT('Ctrl Pts',(12.1071221516794,-21.0489433681523,10.8194689670457));
#53897=CARTESIAN_POINT('Ctrl Pts',(13.1093104456794,-20.6990109732753,11.4761470369039));
#53898=CARTESIAN_POINT('Ctrl Pts',(13.8683648550469,-20.4006353577185,11.9768494012792));
#53899=CARTESIAN_POINT('Ctrl Pts',(14.4658363655178,-20.136535574814,12.413145511352));
#53900=CARTESIAN_POINT('Ctrl Pts',(15.5292386507845,-19.5672964049095,13.3088706944097));
#53901=CARTESIAN_POINT('Ctrl Pts',(16.2561779329736,-19.0831769560747,13.9986415819097));
#53902=CARTESIAN_POINT('Ctrl Pts',(17.0018880874651,-18.5434600004101,14.6847508610486));
#53903=CARTESIAN_POINT('Ctrl Pts',(17.5710595442823,-18.0894667653548,15.2426602928667));
#53904=CARTESIAN_POINT('Ctrl Pts',(18.6068613700326,-17.129093535584,16.3355437642704));
#53905=CARTESIAN_POINT('Ctrl Pts',(19.3243916655247,-16.3344548929372,17.1296950555117));
#53906=CARTESIAN_POINT('Ctrl Pts',(20.0666972723063,-15.4594613044778,17.9021666930174));
#53907=CARTESIAN_POINT('Ctrl Pts',(20.6168159622415,-14.7547166790696,18.4938305405518));
#53908=CARTESIAN_POINT('Ctrl Pts',(21.6393971978862,-13.274017342785,19.6095065175213));
#53909=CARTESIAN_POINT('Ctrl Pts',(22.3554713915253,-12.0805610478001,20.3609361957837));
#53910=CARTESIAN_POINT('Ctrl Pts',(23.4866975992548,-10.1234946186001,21.4058157420793));
#53911=CARTESIAN_POINT('Ctrl Pts',(24.125246467622,-8.89054296253175,21.9361966402162));
#53912=CARTESIAN_POINT('Ctrl Pts',(24.727666267572,-7.59819629859098,22.3697186090524));
#53913=CARTESIAN_POINT('Ctrl Pts',(2.1,-30.4929525674227,13.6857073712154));
#53914=CARTESIAN_POINT('Ctrl Pts',(2.73333333333333,-30.4929525674227,13.6857073712154));
#53915=CARTESIAN_POINT('Ctrl Pts',(3.36508111731483,-30.4928630358999,13.6858268427981));
#53916=CARTESIAN_POINT('Ctrl Pts',(4.12166372313058,-30.4928374222987,13.6858596139329));
#53917=CARTESIAN_POINT('Ctrl Pts',(4.34922070449677,-30.49449304522,13.6822752188327));
#53918=CARTESIAN_POINT('Ctrl Pts',(4.83581952795261,-30.5023484303467,13.6653239915311));
#53919=CARTESIAN_POINT('Ctrl Pts',(5.71994990272322,-30.5214481532399,13.6241663122579));
#53920=CARTESIAN_POINT('Ctrl Pts',(6.54867625091358,-30.5227115994799,13.6214678470964));
#53921=CARTESIAN_POINT('Ctrl Pts',(7.19744568466461,-30.4845039603552,13.7032562477442));
#53922=CARTESIAN_POINT('Ctrl Pts',(7.32540386607941,-30.4768448962739,13.7200563246537));
#53923=CARTESIAN_POINT('Ctrl Pts',(7.52886144254688,-30.4640499949291,13.7487976356855));
#53924=CARTESIAN_POINT('Ctrl Pts',(7.73071526159972,-30.4505000752736,13.7797645234549));
#53925=CARTESIAN_POINT('Ctrl Pts',(8.14014718867705,-30.4209316168907,13.8478073053149));
#53926=CARTESIAN_POINT('Ctrl Pts',(8.76321456595858,-30.3661751673437,13.9737656730329));
#53927=CARTESIAN_POINT('Ctrl Pts',(9.46268739969009,-30.274901687886,14.1717203974558));
#53928=CARTESIAN_POINT('Ctrl Pts',(10.017555629263,-30.1757507026565,14.3751176598203));
#53929=CARTESIAN_POINT('Ctrl Pts',(10.2918140826348,-30.1160627467491,14.4936111394812));
#53930=CARTESIAN_POINT('Ctrl Pts',(11.0595965108885,-29.9308924752226,14.8550046648317));
#53931=CARTESIAN_POINT('Ctrl Pts',(12.2112890847585,-29.538742900038,15.6451338086644));
#53932=CARTESIAN_POINT('Ctrl Pts',(13.2034136834303,-29.0396659631087,16.5569799806426));
#53933=CARTESIAN_POINT('Ctrl Pts',(13.9587824395507,-28.6121062675108,17.2559421918816));
#53934=CARTESIAN_POINT('Ctrl Pts',(14.5428434697006,-28.2415332240579,17.8540725971182));
#53935=CARTESIAN_POINT('Ctrl Pts',(15.5916053350762,-27.4389567528664,19.089267636165));
#53936=CARTESIAN_POINT('Ctrl Pts',(16.312366647535,-26.7539934204414,20.045818201422));
#53937=CARTESIAN_POINT('Ctrl Pts',(17.0564138076615,-25.9843342941303,21.0043101087993));
#53938=CARTESIAN_POINT('Ctrl Pts',(17.6163463570722,-25.3506638339921,21.7688212811574));
#53939=CARTESIAN_POINT('Ctrl Pts',(18.6452383036686,-23.9966999747395,23.2835440124754));
#53940=CARTESIAN_POINT('Ctrl Pts',(19.3594664110678,-22.873824767894,24.3879531932759));
#53941=CARTESIAN_POINT('Ctrl Pts',(20.100955640781,-21.6310467382024,25.4670642243813));
#53942=CARTESIAN_POINT('Ctrl Pts',(20.6466714554163,-20.6438263892792,26.2831266089234));
#53943=CARTESIAN_POINT('Ctrl Pts',(21.666430039865,-18.5543852156517,27.8345444051144));
#53944=CARTESIAN_POINT('Ctrl Pts',(22.3810701794161,-16.8676153595205,28.8806138340969));
#53945=CARTESIAN_POINT('Ctrl Pts',(23.5117719637955,-14.094719744574,30.3366076891904));
#53946=CARTESIAN_POINT('Ctrl Pts',(24.1480627906507,-12.3610095563398,31.0685341627222));
#53947=CARTESIAN_POINT('Ctrl Pts',(24.7493903499091,-10.540466346655,31.6671511473888));
#53948=CARTESIAN_POINT('Ctrl Pts',(2.1,-35.5190472550673,16.1061470045084));
#53949=CARTESIAN_POINT('Ctrl Pts',(2.73333333333333,-35.5190472550673,16.1061470045084));
#53950=CARTESIAN_POINT('Ctrl Pts',(3.36475413268099,-35.5189670351233,16.1062505100172));
#53951=CARTESIAN_POINT('Ctrl Pts',(4.12102956711596,-35.5189449021359,16.1062772345771));
#53952=CARTESIAN_POINT('Ctrl Pts',(4.34476326499953,-35.5208619030567,16.1021711888042));
#53953=CARTESIAN_POINT('Ctrl Pts',(4.82891764559021,-35.5300406854563,16.0825700940178));
#53954=CARTESIAN_POINT('Ctrl Pts',(5.71373811875233,-35.5525489027151,16.0345554335906));
#53955=CARTESIAN_POINT('Ctrl Pts',(6.55602060536393,-35.5543403393864,16.0307742128651));
#53956=CARTESIAN_POINT('Ctrl Pts',(7.21864005381085,-35.5082991666069,16.1284303018243));
#53957=CARTESIAN_POINT('Ctrl Pts',(7.34676507585227,-35.4992701924678,16.1480328226317));
#53958=CARTESIAN_POINT('Ctrl Pts',(7.55208983697808,-35.4840500176732,16.1818617453272));
#53959=CARTESIAN_POINT('Ctrl Pts',(7.75545246761066,-35.4679543088847,16.2182492540178));
#53960=CARTESIAN_POINT('Ctrl Pts',(8.16859508244807,-35.432763206004,16.2983357838761));
#53961=CARTESIAN_POINT('Ctrl Pts',(8.79795126468624,-35.3675282937919,16.4467433812652));
#53962=CARTESIAN_POINT('Ctrl Pts',(9.50492466084984,-35.2587512344281,16.6802493752873));
#53963=CARTESIAN_POINT('Ctrl Pts',(10.0643308640972,-35.1410338487819,16.9194777147605));
#53964=CARTESIAN_POINT('Ctrl Pts',(10.3400534304426,-35.0704395069489,17.0583708781951));
#53965=CARTESIAN_POINT('Ctrl Pts',(11.1102119878275,-34.8520710674395,17.4808514386373));
#53966=CARTESIAN_POINT('Ctrl Pts',(12.2545037825343,-34.3944746405569,18.3945372313141));
#53967=CARTESIAN_POINT('Ctrl Pts',(13.2428241044381,-33.8115307458597,19.45071368533));
#53968=CARTESIAN_POINT('Ctrl Pts',(13.996383095991,-33.3108813879676,20.2623381758305));
#53969=CARTESIAN_POINT('Ctrl Pts',(14.5753829446244,-32.8807198531287,20.9514986906474));
#53970=CARTESIAN_POINT('Ctrl Pts',(15.6192678372118,-31.9450395751563,22.3814785397995));
#53971=CARTESIAN_POINT('Ctrl Pts',(16.3374176744543,-31.1455802637508,23.4909182338773));
#53972=CARTESIAN_POINT('Ctrl Pts',(17.0806574874892,-30.2449968793303,24.6052817498839));
#53973=CARTESIAN_POINT('Ctrl Pts',(17.6370457520303,-29.5081260556649,25.4890808130937));
#53974=CARTESIAN_POINT('Ctrl Pts',(18.6628364663185,-27.9284442945199,27.2466455033113));
#53975=CARTESIAN_POINT('Ctrl Pts',(19.3754944079007,-26.618087896118,28.5289319062647));
#53976=CARTESIAN_POINT('Ctrl Pts',(20.1166524072473,-25.1655401045655,29.7835633599642));
#53977=CARTESIAN_POINT('Ctrl Pts',(20.6600335100608,-24.0162045057133,30.728885186263));
#53978=CARTESIAN_POINT('Ctrl Pts',(21.6778210050225,-21.5784381766374,32.5302297375723));
#53979=CARTESIAN_POINT('Ctrl Pts',(22.3918241741696,-19.6099219678105,33.7451822199181));
#53980=CARTESIAN_POINT('Ctrl Pts',(23.5225185291349,-16.371232079717,35.4366819891224));
#53981=CARTESIAN_POINT('Ctrl Pts',(24.157514841919,-14.3511368126248,36.2844930251905));
#53982=CARTESIAN_POINT('Ctrl Pts',(24.7577717974218,-12.2286456156553,36.977739523394));
#53983=CARTESIAN_POINT('',(24.5,-3.6160301400213,9.01602984623715));
#53984=CARTESIAN_POINT('Ctrl Pts',(24.5,-3.6160301400213,9.01602984623715));
#53985=CARTESIAN_POINT('Ctrl Pts',(23.8274939346415,-4.25320160821626,8.96293929686807));
#53986=CARTESIAN_POINT('Ctrl Pts',(23.3366347313213,-4.69799730977943,8.91872338222509));
#53987=CARTESIAN_POINT('Ctrl Pts',(22.5855494187791,-5.38681087917914,8.84785629468263));
#53988=CARTESIAN_POINT('Ctrl Pts',(22.2454144271855,-5.69874561378915,8.81576356723475));
#53989=CARTESIAN_POINT('Ctrl Pts',(21.8382660741845,-6.08207973842203,8.77028857443063));
#53990=CARTESIAN_POINT('Ctrl Pts',(21.3802156946739,-6.52138636350872,8.71704071219447));
#53991=CARTESIAN_POINT('Ctrl Pts',(20.76946932905,-7.10714054398311,8.64604210638015));
#53992=CARTESIAN_POINT('Ctrl Pts',(20.1629003032131,-7.69806831767953,8.57558750201974));
#53993=CARTESIAN_POINT('Ctrl Pts',(19.5574857571565,-8.2922929633463,8.53317747320063));
#53994=CARTESIAN_POINT('Ctrl Pts',(18.6418529406584,-9.19100210320499,8.46903627542409));
#53995=CARTESIAN_POINT('Ctrl Pts',(17.7734813303986,-10.1341856434662,8.39329925092376));
#53996=CARTESIAN_POINT('Ctrl Pts',(16.962125308111,-11.0447214443253,8.38345588031826));
#53997=CARTESIAN_POINT('Ctrl Pts',(16.8133360650119,-11.211698614523,8.38165076934145));
#53998=CARTESIAN_POINT('Ctrl Pts',(16.6656205359918,-11.3787950950318,8.38175879297581));
#53999=CARTESIAN_POINT('Ctrl Pts',(16.5183901926363,-11.5466151675562,8.38398696714523));
#54000=CARTESIAN_POINT('Ctrl Pts',(15.726452288761,-12.4493032509656,8.39597210241662));
#54001=CARTESIAN_POINT('Ctrl Pts',(14.9462259720485,-13.4308510041996,8.39966576114259));
#54002=CARTESIAN_POINT('Ctrl Pts',(14.2963150416359,-14.2718135557227,8.45082997390809));
#54003=CARTESIAN_POINT('Ctrl Pts',(13.9908350935056,-14.6670941774161,8.47487887096513));
#54004=CARTESIAN_POINT('Ctrl Pts',(13.7077063567372,-15.0401421211308,8.50738131960351));
#54005=CARTESIAN_POINT('Ctrl Pts',(13.4460198946299,-15.3890269033268,8.54665986878341));
#54006=CARTESIAN_POINT('Ctrl Pts',(12.837329540793,-16.2005430964578,8.63802292136927));
#54007=CARTESIAN_POINT('Ctrl Pts',(12.3530827413148,-16.8928758746813,8.71916608145024));
#54008=CARTESIAN_POINT('Ctrl Pts',(11.9770275692621,-17.438094619976,8.79813803422803));
#54009=CARTESIAN_POINT('Ctrl Pts',(11.6553972431166,-17.9044062037594,8.86568071630212));
#54010=CARTESIAN_POINT('Ctrl Pts',(11.3684205616876,-18.3299004046869,8.93687349930713));
#54011=CARTESIAN_POINT('Ctrl Pts',(11.0710856781329,-18.7780770165651,9.0258659640707));
#54012=CARTESIAN_POINT('Ctrl Pts',(10.8141787015661,-19.165316135464,9.10275833803743));
#54013=CARTESIAN_POINT('Ctrl Pts',(10.5576802661834,-19.557808848585,9.19120852767749));
#54014=CARTESIAN_POINT('Ctrl Pts',(10.2957959918397,-19.9646028342318,9.29767556265455));
#54015=CARTESIAN_POINT('Ctrl Pts',(9.71459276345261,-20.8674060985318,9.53395925933903));
#54016=CARTESIAN_POINT('Ctrl Pts',(9.09527967376161,-21.8590210236913,9.85968483500704));
#54017=CARTESIAN_POINT('Ctrl Pts',(8.43168033652491,-23.0030033264912,10.2883786384855));
#54018=CARTESIAN_POINT('Ctrl Pts',(7.97964340480209,-23.7822721127686,10.5804003761503));
#54019=CARTESIAN_POINT('Ctrl Pts',(7.52291961074489,-24.6086571529433,10.9125713605893));
#54020=CARTESIAN_POINT('Ctrl Pts',(7.10363554125516,-25.4084375301234,11.2437787817976));
#54021=CARTESIAN_POINT('Ctrl Pts',(6.56327799553922,-26.4391644123796,11.670626454462));
#54022=CARTESIAN_POINT('Ctrl Pts',(6.08559840020574,-27.3990249331094,12.1272301632502));
#54023=CARTESIAN_POINT('Ctrl Pts',(5.61708670825588,-28.397040125486,12.6190019907712));
#54024=CARTESIAN_POINT('Ctrl Pts',(5.04102956501762,-29.6241467068311,13.2236585638182));
#54025=CARTESIAN_POINT('Ctrl Pts',(4.50102820502357,-30.867297253229,13.8659822705852));
#54026=CARTESIAN_POINT('Ctrl Pts',(4.,-32.1353158291841,14.4766278329416));
#54027=CARTESIAN_POINT('Ctrl Pts',(3.72183418897115,-32.8393069658979,14.8156520962484));
#54028=CARTESIAN_POINT('Ctrl Pts',(3.45538353518228,-33.5466020895644,15.1562674758126));
#54029=CARTESIAN_POINT('Ctrl Pts',(3.2,-34.2572188230213,15.4984824583453));
#54030=CARTESIAN_POINT('',(24.5,-9.18141366427805,25.390975623741));
#54031=CARTESIAN_POINT('Ctrl Pts',(24.5,-9.18141366427807,25.390975623741));
#54032=CARTESIAN_POINT('Ctrl Pts',(24.5,-8.77450678650653,24.2210276048427));
#54033=CARTESIAN_POINT('Ctrl Pts',(24.5,-8.37535144524489,23.0706175167593));
#54034=CARTESIAN_POINT('Ctrl Pts',(24.5,-6.73049557719857,18.3152928195099));
#54035=CARTESIAN_POINT('Ctrl Pts',(24.5,-4.99261102906233,13.2639411997441));
#54036=CARTESIAN_POINT('Ctrl Pts',(24.5,-3.6160301400213,9.01602984623715));
#54037=CARTESIAN_POINT('',(10.2670750393577,-30.770480162676,14.8182822548653));
#54038=CARTESIAN_POINT('Ctrl Pts',(10.2670750393577,-30.770480162676,14.8182822548653));
#54039=CARTESIAN_POINT('Ctrl Pts',(11.2293198185888,-29.7752240113353,14.8555820456021));
#54040=CARTESIAN_POINT('Ctrl Pts',(12.092802582344,-28.8440362457489,15.1636363299831));
#54041=CARTESIAN_POINT('Ctrl Pts',(14.3080979519049,-26.4010410885782,16.2798551113026));
#54042=CARTESIAN_POINT('Ctrl Pts',(14.8952017874601,-25.7386194595791,16.6851511994675));
#54043=CARTESIAN_POINT('Ctrl Pts',(17.0803363586062,-22.9312839164232,18.4974195815112));
#54044=CARTESIAN_POINT('Ctrl Pts',(17.6922811489506,-22.0817386820725,19.0546305604886));
#54045=CARTESIAN_POINT('Ctrl Pts',(19.0755427322033,-19.9947258593395,20.4139220475843));
#54046=CARTESIAN_POINT('Ctrl Pts',(20.2687424742408,-18.1038001636999,21.6078133727585));
#54047=CARTESIAN_POINT('Ctrl Pts',(22.3267279388309,-14.0665238542576,23.6582159112932));
#54048=CARTESIAN_POINT('Ctrl Pts',(23.4192562717209,-11.8118967310364,24.635842795693));
#54049=CARTESIAN_POINT('Ctrl Pts',(24.5,-9.18141366427807,25.390975623741));
#54050=CARTESIAN_POINT('Ctrl Pts',(6.,-35.548403009865,16.0409177869666));
#54051=CARTESIAN_POINT('Ctrl Pts',(7.51604047332548,-33.6030946132751,15.107667867014));
#54052=CARTESIAN_POINT('Ctrl Pts',(9.08449301626627,-31.993289619074,14.872473123897));
#54053=CARTESIAN_POINT('Ctrl Pts',(9.8624969752411,-31.1881020850933,14.8146152631462));
#54054=CARTESIAN_POINT('Ctrl Pts',(10.0667253012217,-30.97770322442,14.8105160362608));
#54055=CARTESIAN_POINT('Ctrl Pts',(10.2670750393577,-30.770480162676,14.8182822548653));
#54056=CARTESIAN_POINT('Origin',(24.5,-7.65823537717056,3.68801178249925));
#54057=CARTESIAN_POINT('',(24.5,-1.17476144568584,9.64284209699151));
#54058=CARTESIAN_POINT('Ctrl Pts',(24.5,-1.17476144568584,9.64284209699151));
#54059=CARTESIAN_POINT('Ctrl Pts',(24.5,-1.44558163417187,9.6098488038372));
#54060=CARTESIAN_POINT('Ctrl Pts',(24.5,-1.71513676748961,9.56543133792098));
#54061=CARTESIAN_POINT('Ctrl Pts',(24.5,-2.54106347065763,9.39323084353225));
#54062=CARTESIAN_POINT('Ctrl Pts',(24.5,-3.0875901120013,9.22796959145788));
#54063=CARTESIAN_POINT('Ctrl Pts',(24.5,-3.6160301400213,9.01602984623715));
#54064=CARTESIAN_POINT('',(24.5,-4.10202091932642,26.6865776070557));
#54065=CARTESIAN_POINT('Ctrl Pts',(24.5,-1.17476144568584,9.64284209699151));
#54066=CARTESIAN_POINT('Ctrl Pts',(24.5,-1.96806264976098,13.8771085227549));
#54067=CARTESIAN_POINT('Ctrl Pts',(24.5,-2.92680106052676,19.5450505664343));
#54068=CARTESIAN_POINT('Ctrl Pts',(24.5,-4.10202091932642,26.6865776070557));
#54069=CARTESIAN_POINT('Origin',(24.5,0.,0.));
#54070=CARTESIAN_POINT('Ctrl Pts',(24.5,-4.10202064021797,26.6865776499578));
#54071=CARTESIAN_POINT('Ctrl Pts',(24.5,-18.1565214583376,24.5262462204244));
#54072=CARTESIAN_POINT('Ctrl Pts',(24.5,-24.3261594333653,11.7148609561741));
#54073=CARTESIAN_POINT('Ctrl Pts',(24.5,-36.0410203895394,-12.6112984771912));
#54074=CARTESIAN_POINT('Ctrl Pts',(24.5,-11.7148609561741,-24.3261594333653));
#54075=CARTESIAN_POINT('Ctrl Pts',(24.5,12.6112984771912,-36.0410203895394));
#54076=CARTESIAN_POINT('Ctrl Pts',(24.5,24.3261594333653,-11.7148609561741));
#54077=CARTESIAN_POINT('Ctrl Pts',(24.5,36.0410203895394,12.6112984771912));
#54078=CARTESIAN_POINT('Ctrl Pts',(24.5,11.7148609561741,24.3261594333653));
#54079=CARTESIAN_POINT('Ctrl Pts',(24.5,4.17235284052387,27.9584399040123));
#54080=CARTESIAN_POINT('Ctrl Pts',(24.5,-4.10202064021797,26.6865776499578));
#54081=CARTESIAN_POINT('Ctrl Pts',(24.3078118955742,-4.10700177686883,26.7189835059193));
#54082=CARTESIAN_POINT('Ctrl Pts',(24.3078118955742,-18.1785691568795,24.5560287580252));
#54083=CARTESIAN_POINT('Ctrl Pts',(24.3078118955742,-24.355699002996,11.7290864631587));
#54084=CARTESIAN_POINT('Ctrl Pts',(24.3078118955742,-36.0847854661547,-12.6266125398373));
#54085=CARTESIAN_POINT('Ctrl Pts',(24.3078118955742,-11.7290864631587,-24.355699002996));
#54086=CARTESIAN_POINT('Ctrl Pts',(24.3078118955742,12.6266125398373,-36.0847854661547));
#54087=CARTESIAN_POINT('Ctrl Pts',(24.3078118955742,24.355699002996,-11.7290864631587));
#54088=CARTESIAN_POINT('Ctrl Pts',(24.3078118955742,36.0847854661547,12.6266125398373));
#54089=CARTESIAN_POINT('Ctrl Pts',(24.3078118955742,11.7290864631587,24.355699002996));
#54090=CARTESIAN_POINT('Ctrl Pts',(24.3078118955742,4.17741938247407,27.9923901987381));
#54091=CARTESIAN_POINT('Ctrl Pts',(24.3078118955742,-4.10700177686883,26.7189835059193));
#54092=CARTESIAN_POINT('Ctrl Pts',(23.9225830034177,-4.11759678467036,26.7879116082368));
#54093=CARTESIAN_POINT('Ctrl Pts',(23.9225830034177,-18.2254651877316,24.6193769936484));
#54094=CARTESIAN_POINT('Ctrl Pts',(23.9225830034177,-24.4185304393985,11.7593444881934));
#54095=CARTESIAN_POINT('Ctrl Pts',(23.9225830034177,-36.1778749275919,-12.6591859512051));
#54096=CARTESIAN_POINT('Ctrl Pts',(23.9225830034177,-11.7593444881934,-24.4185304393985));
#54097=CARTESIAN_POINT('Ctrl Pts',(23.9225830034177,12.6591859512051,-36.1778749275919));
#54098=CARTESIAN_POINT('Ctrl Pts',(23.9225830034177,24.4185304393985,-11.7593444881934));
#54099=CARTESIAN_POINT('Ctrl Pts',(23.9225830034177,36.1778749275919,12.6591859512051));
#54100=CARTESIAN_POINT('Ctrl Pts',(23.9225830034177,11.7593444881934,24.4185304393985));
#54101=CARTESIAN_POINT('Ctrl Pts',(23.9225830034177,4.18819604957873,28.0646033626596));
#54102=CARTESIAN_POINT('Ctrl Pts',(23.9225830034177,-4.11759678467036,26.7879116082368));
#54103=CARTESIAN_POINT('Ctrl Pts',(23.3421815947946,-4.13538749346637,26.9036528912225));
#54104=CARTESIAN_POINT('Ctrl Pts',(23.3421815947946,-18.3042111069615,24.7257487900476));
#54105=CARTESIAN_POINT('Ctrl Pts',(23.3421815947946,-24.5240344474382,11.8101525406477));
#54106=CARTESIAN_POINT('Ctrl Pts',(23.3421815947946,-36.3341869880859,-12.7138819067904));
#54107=CARTESIAN_POINT('Ctrl Pts',(23.3421815947946,-11.8101525406477,-24.5240344474382));
#54108=CARTESIAN_POINT('Ctrl Pts',(23.3421815947946,12.7138819067904,-36.3341869880859));
#54109=CARTESIAN_POINT('Ctrl Pts',(23.3421815947946,24.5240344474382,-11.8101525406477));
#54110=CARTESIAN_POINT('Ctrl Pts',(23.3421815947946,36.3341869880859,12.7138819067904));
#54111=CARTESIAN_POINT('Ctrl Pts',(23.3421815947946,11.8101525406477,24.5240344474382));
#54112=CARTESIAN_POINT('Ctrl Pts',(23.3421815947946,4.20629179333296,28.1858607882918));
#54113=CARTESIAN_POINT('Ctrl Pts',(23.3421815947946,-4.13538749346637,26.9036528912225));
#54114=CARTESIAN_POINT('Ctrl Pts',(22.5631762070947,-4.16292037730343,27.0827739895517));
#54115=CARTESIAN_POINT('Ctrl Pts',(22.5631762070947,-18.4260782158922,24.8903696799392));
#54116=CARTESIAN_POINT('Ctrl Pts',(22.5631762070947,-24.6873123488983,11.8887830338031));
#54117=CARTESIAN_POINT('Ctrl Pts',(22.5631762070947,-36.5760953827013,-12.7985293150952));
#54118=CARTESIAN_POINT('Ctrl Pts',(22.5631762070947,-11.8887830338031,-24.6873123488983));
#54119=CARTESIAN_POINT('Ctrl Pts',(22.5631762070947,12.7985293150952,-36.5760953827013));
#54120=CARTESIAN_POINT('Ctrl Pts',(22.5631762070947,24.6873123488983,-11.8887830338031));
#54121=CARTESIAN_POINT('Ctrl Pts',(22.5631762070947,36.5760953827013,12.7985293150952));
#54122=CARTESIAN_POINT('Ctrl Pts',(22.5631762070947,11.8887830338031,24.6873123488983));
#54123=CARTESIAN_POINT('Ctrl Pts',(22.5631762070947,4.23429674897826,28.3735186636802));
#54124=CARTESIAN_POINT('Ctrl Pts',(22.5631762070947,-4.16292037730343,27.0827739895517));
#54125=CARTESIAN_POINT('Ctrl Pts',(21.5808622776984,-4.20380096926686,27.3487314742879));
#54126=CARTESIAN_POINT('Ctrl Pts',(21.5808622776984,-18.6070254636793,25.1347973784011));
#54127=CARTESIAN_POINT('Ctrl Pts',(21.5808622776984,-24.929745989549,12.0055329218856));
#54128=CARTESIAN_POINT('Ctrl Pts',(21.5808622776984,-36.9352789114346,-12.9242130676634));
#54129=CARTESIAN_POINT('Ctrl Pts',(21.5808622776984,-12.0055329218856,-24.929745989549));
#54130=CARTESIAN_POINT('Ctrl Pts',(21.5808622776984,12.9242130676634,-36.9352789114346));
#54131=CARTESIAN_POINT('Ctrl Pts',(21.5808622776984,24.929745989549,-12.0055329218856));
#54132=CARTESIAN_POINT('Ctrl Pts',(21.5808622776984,36.9352789114346,12.9242130676634));
#54133=CARTESIAN_POINT('Ctrl Pts',(21.5808622776984,12.0055329218856,24.929745989549));
#54134=CARTESIAN_POINT('Ctrl Pts',(21.5808622776984,4.27587826915116,28.6521514824534));
#54135=CARTESIAN_POINT('Ctrl Pts',(21.5808622776984,-4.20380096926686,27.3487314742879));
#54136=CARTESIAN_POINT('Ctrl Pts',(20.5902243197586,-4.25132104313727,27.6578835367717));
#54137=CARTESIAN_POINT('Ctrl Pts',(20.5902243197586,-18.8173606415355,25.4189229678073));
#54138=CARTESIAN_POINT('Ctrl Pts',(20.5902243197586,-25.2115536630461,12.141244344827));
#54139=CARTESIAN_POINT('Ctrl Pts',(20.5902243197586,-37.3527980078731,-13.0703093182191));
#54140=CARTESIAN_POINT('Ctrl Pts',(20.5902243197586,-12.141244344827,-25.2115536630461));
#54141=CARTESIAN_POINT('Ctrl Pts',(20.5902243197586,13.0703093182191,-37.3527980078731));
#54142=CARTESIAN_POINT('Ctrl Pts',(20.5902243197586,25.2115536630461,-12.141244344827));
#54143=CARTESIAN_POINT('Ctrl Pts',(20.5902243197586,37.3527980078731,13.0703093182191));
#54144=CARTESIAN_POINT('Ctrl Pts',(20.5902243197586,12.141244344827,25.2115536630461));
#54145=CARTESIAN_POINT('Ctrl Pts',(20.5902243197586,4.32421311009545,28.9760375001185));
#54146=CARTESIAN_POINT('Ctrl Pts',(20.5902243197586,-4.25132104313727,27.6578835367717));
#54147=CARTESIAN_POINT('Ctrl Pts',(19.591895069338,-4.30570507106198,28.011690528843));
#54148=CARTESIAN_POINT('Ctrl Pts',(19.591895069338,-19.0580773167089,25.7440885816178));
#54149=CARTESIAN_POINT('Ctrl Pts',(19.591895069338,-25.5340665536333,12.296558367172));
#54150=CARTESIAN_POINT('Ctrl Pts',(19.591895069338,-37.8306249208053,-13.2375081864613));
#54151=CARTESIAN_POINT('Ctrl Pts',(19.591895069338,-12.296558367172,-25.5340665536333));
#54152=CARTESIAN_POINT('Ctrl Pts',(19.591895069338,13.2375081864613,-37.8306249208053));
#54153=CARTESIAN_POINT('Ctrl Pts',(19.591895069338,25.5340665536333,-12.296558367172));
#54154=CARTESIAN_POINT('Ctrl Pts',(19.591895069338,37.8306249208053,13.2375081864613));
#54155=CARTESIAN_POINT('Ctrl Pts',(19.591895069338,12.296558367172,25.5340665536333));
#54156=CARTESIAN_POINT('Ctrl Pts',(19.591895069338,4.37952959270064,29.3467066677876));
#54157=CARTESIAN_POINT('Ctrl Pts',(19.591895069338,-4.30570507106198,28.011690528843));
#54158=CARTESIAN_POINT('Ctrl Pts',(18.5871162949016,-4.36721109149925,28.4118311751982));
#54159=CARTESIAN_POINT('Ctrl Pts',(18.5871162949016,-19.3303176289436,26.1118370484326));
#54160=CARTESIAN_POINT('Ctrl Pts',(18.5871162949016,-25.8988149034099,12.4722119146764));
#54161=CARTESIAN_POINT('Ctrl Pts',(18.5871162949016,-38.3710268180862,-13.4266029887335));
#54162=CARTESIAN_POINT('Ctrl Pts',(18.5871162949016,-12.4722119146764,-25.8988149034099));
#54163=CARTESIAN_POINT('Ctrl Pts',(18.5871162949016,13.4266029887335,-38.3710268180862));
#54164=CARTESIAN_POINT('Ctrl Pts',(18.5871162949016,25.8988149034099,-12.4722119146764));
#54165=CARTESIAN_POINT('Ctrl Pts',(18.5871162949016,38.3710268180862,13.4266029887335));
#54166=CARTESIAN_POINT('Ctrl Pts',(18.5871162949016,12.4722119146764,25.8988149034099));
#54167=CARTESIAN_POINT('Ctrl Pts',(18.5871162949016,4.44209017968666,29.7659177169156));
#54168=CARTESIAN_POINT('Ctrl Pts',(18.5871162949016,-4.36721109149925,28.4118311751982));
#54169=CARTESIAN_POINT('Ctrl Pts',(17.577868433379,-4.43610045989054,28.8600057798811));
#54170=CARTESIAN_POINT('Ctrl Pts',(17.577868433379,-19.6352383997424,26.5237310293085));
#54171=CARTESIAN_POINT('Ctrl Pts',(17.577868433379,-26.3073486251372,12.6689513859872));
#54172=CARTESIAN_POINT('Ctrl Pts',(17.577868433379,-38.9763000111244,-13.63839723915));
#54173=CARTESIAN_POINT('Ctrl Pts',(17.577868433379,-12.6689513859872,-26.3073486251372));
#54174=CARTESIAN_POINT('Ctrl Pts',(17.577868433379,13.63839723915,-38.9763000111244));
#54175=CARTESIAN_POINT('Ctrl Pts',(17.577868433379,26.3073486251372,-12.6689513859872));
#54176=CARTESIAN_POINT('Ctrl Pts',(17.577868433379,38.9763000111244,13.63839723915));
#54177=CARTESIAN_POINT('Ctrl Pts',(17.577868433379,12.6689513859872,26.3073486251372));
#54178=CARTESIAN_POINT('Ctrl Pts',(17.577868433379,4.51216070762872,30.2354519867605));
#54179=CARTESIAN_POINT('Ctrl Pts',(17.577868433379,-4.43610045989054,28.8600057798811));
#54180=CARTESIAN_POINT('Ctrl Pts',(16.5668667015923,-4.51259168970781,29.3576359292874));
#54181=CARTESIAN_POINT('Ctrl Pts',(16.5668667015923,-19.9738068218355,26.9810770304007));
#54182=CARTESIAN_POINT('Ctrl Pts',(16.5668667015923,-26.7609635664043,12.8874008284133));
#54183=CARTESIAN_POINT('Ctrl Pts',(16.5668667015923,-39.6483643948176,-13.873562737991));
#54184=CARTESIAN_POINT('Ctrl Pts',(16.5668667015923,-12.8874008284133,-26.7609635664043));
#54185=CARTESIAN_POINT('Ctrl Pts',(16.5668667015923,13.873562737991,-39.6483643948176));
#54186=CARTESIAN_POINT('Ctrl Pts',(16.5668667015923,26.7609635664043,-12.8874008284133));
#54187=CARTESIAN_POINT('Ctrl Pts',(16.5668667015923,39.6483643948176,13.873562737991));
#54188=CARTESIAN_POINT('Ctrl Pts',(16.5668667015923,12.8874008284133,26.7609635664043));
#54189=CARTESIAN_POINT('Ctrl Pts',(16.5668667015923,4.58996343657508,30.7567988154581));
#54190=CARTESIAN_POINT('Ctrl Pts',(16.5668667015923,-4.51259168970781,29.3576359292874));
#54191=CARTESIAN_POINT('Ctrl Pts',(15.5576189940876,-4.59680623544197,29.9055117717334));
#54192=CARTESIAN_POINT('Ctrl Pts',(15.5576189940876,-20.3465604817598,27.4846012359511));
#54193=CARTESIAN_POINT('Ctrl Pts',(15.5576189940876,-27.2603799871926,13.1279071008807));
#54194=CARTESIAN_POINT('Ctrl Pts',(15.5576189940876,-40.3882870880733,-14.1324728863119));
#54195=CARTESIAN_POINT('Ctrl Pts',(15.5576189940876,-13.1279071008807,-27.2603799871926));
#54196=CARTESIAN_POINT('Ctrl Pts',(15.5576189940876,14.1324728863119,-40.3882870880733));
#54197=CARTESIAN_POINT('Ctrl Pts',(15.5576189940876,27.2603799871926,-13.1279071008807));
#54198=CARTESIAN_POINT('Ctrl Pts',(15.5576189940876,40.3882870880733,14.1324728863119));
#54199=CARTESIAN_POINT('Ctrl Pts',(15.5576189940876,13.1279071008807,27.2603799871926));
#54200=CARTESIAN_POINT('Ctrl Pts',(15.5576189940876,4.67562190344439,31.3307860092005));
#54201=CARTESIAN_POINT('Ctrl Pts',(15.5576189940876,-4.59680623544197,29.9055117717334));
#54202=CARTESIAN_POINT('Ctrl Pts',(14.5544447688713,-4.68871703666209,30.503457259765));
#54203=CARTESIAN_POINT('Ctrl Pts',(14.5544447688713,-20.7533796035957,28.0341418498963));
#54204=CARTESIAN_POINT('Ctrl Pts',(14.5544447688713,-27.805437411382,13.3903929221629));
#54205=CARTESIAN_POINT('Ctrl Pts',(14.5544447688713,-41.1958303335449,-14.4150444892191));
#54206=CARTESIAN_POINT('Ctrl Pts',(14.5544447688713,-13.3903929221629,-27.805437411382));
#54207=CARTESIAN_POINT('Ctrl Pts',(14.5544447688713,14.4150444892191,-41.1958303335449));
#54208=CARTESIAN_POINT('Ctrl Pts',(14.5544447688713,27.805437411382,-13.3903929221629));
#54209=CARTESIAN_POINT('Ctrl Pts',(14.5544447688713,41.1958303335449,14.4150444892191));
#54210=CARTESIAN_POINT('Ctrl Pts',(14.5544447688713,13.3903929221629,27.805437411382));
#54211=CARTESIAN_POINT('Ctrl Pts',(14.5544447688713,4.76910858383447,31.9572291302439));
#54212=CARTESIAN_POINT('Ctrl Pts',(14.5544447688713,-4.68871703666209,30.503457259765));
#54213=CARTESIAN_POINT('Ctrl Pts',(13.5625963827217,-4.78806279521497,31.1497724620392));
#54214=CARTESIAN_POINT('Ctrl Pts',(13.5625963827217,-21.1931076194119,28.6281365537097));
#54215=CARTESIAN_POINT('Ctrl Pts',(13.5625963827217,-28.3945862659469,13.6741120572209));
#54216=CARTESIAN_POINT('Ctrl Pts',(13.5625963827217,-42.0686983231678,-14.720474208726));
#54217=CARTESIAN_POINT('Ctrl Pts',(13.5625963827217,-13.6741120572209,-28.3945862659469));
#54218=CARTESIAN_POINT('Ctrl Pts',(13.5625963827217,14.720474208726,-42.0686983231678));
#54219=CARTESIAN_POINT('Ctrl Pts',(13.5625963827217,28.3945862659469,-13.6741120572209));
#54220=CARTESIAN_POINT('Ctrl Pts',(13.5625963827217,42.0686983231678,14.720474208726));
#54221=CARTESIAN_POINT('Ctrl Pts',(13.5625963827217,13.6741120572209,28.3945862659469));
#54222=CARTESIAN_POINT('Ctrl Pts',(13.5625963827217,4.8701576994406,32.6343472297938));
#54223=CARTESIAN_POINT('Ctrl Pts',(13.5625963827217,-4.78806279521497,31.1497724620392));
#54224=CARTESIAN_POINT('Ctrl Pts',(12.5880795783847,-4.89434668936618,31.8412251978926));
#54225=CARTESIAN_POINT('Ctrl Pts',(12.5880795783847,-21.6635454777474,29.263614818168));
#54226=CARTESIAN_POINT('Ctrl Pts',(12.5880795783847,-29.0248802554437,13.9776456449495));
#54227=CARTESIAN_POINT('Ctrl Pts',(12.5880795783847,-43.0025259003932,-15.0472346104942));
#54228=CARTESIAN_POINT('Ctrl Pts',(12.5880795783847,-13.9776456449495,-29.0248802554437));
#54229=CARTESIAN_POINT('Ctrl Pts',(12.5880795783847,15.0472346104942,-43.0025259003932));
#54230=CARTESIAN_POINT('Ctrl Pts',(12.5880795783847,29.0248802554437,-13.9776456449495));
#54231=CARTESIAN_POINT('Ctrl Pts',(12.5880795783847,43.0025259003932,15.0472346104942));
#54232=CARTESIAN_POINT('Ctrl Pts',(12.5880795783847,13.9776456449495,29.0248802554437));
#54233=CARTESIAN_POINT('Ctrl Pts',(12.5880795783847,4.97826391014952,33.3587540838835));
#54234=CARTESIAN_POINT('Ctrl Pts',(12.5880795783847,-4.89434668936618,31.8412251978926));
#54235=CARTESIAN_POINT('Ctrl Pts',(11.6370973936883,-5.00694477063914,32.5737562362951));
#54236=CARTESIAN_POINT('Ctrl Pts',(11.6370973936883,-22.1619314338677,29.9368460150499));
#54237=CARTESIAN_POINT('Ctrl Pts',(11.6370973936883,-29.6926191863701,14.2992117660733));
#54238=CARTESIAN_POINT('Ctrl Pts',(11.6370973936883,-43.9918309524434,-15.3934074202968));
#54239=CARTESIAN_POINT('Ctrl Pts',(11.6370973936883,-14.2992117660733,-29.6926191863701));
#54240=CARTESIAN_POINT('Ctrl Pts',(11.6370973936883,15.3934074202968,-43.9918309524434));
#54241=CARTESIAN_POINT('Ctrl Pts',(11.6370973936883,29.6926191863701,-14.2992117660733));
#54242=CARTESIAN_POINT('Ctrl Pts',(11.6370973936883,43.9918309524434,15.3934074202968));
#54243=CARTESIAN_POINT('Ctrl Pts',(11.6370973936883,14.2992117660733,29.6926191863701));
#54244=CARTESIAN_POINT('Ctrl Pts',(11.6370973936883,5.09279256942311,34.1261970015792));
#54245=CARTESIAN_POINT('Ctrl Pts',(11.6370973936883,-5.00694477063914,32.5737562362951));
#54246=CARTESIAN_POINT('Ctrl Pts',(10.7155646400367,-5.12517843764354,33.3429507899297));
#54247=CARTESIAN_POINT('Ctrl Pts',(10.7155646400367,-22.6852618362104,30.6437727428344));
#54248=CARTESIAN_POINT('Ctrl Pts',(10.7155646400367,-30.3937787577631,14.6368724193901));
#54249=CARTESIAN_POINT('Ctrl Pts',(10.7155646400367,-45.0306511771533,-15.756906338373));
#54250=CARTESIAN_POINT('Ctrl Pts',(10.7155646400367,-14.6368724193901,-30.3937787577631));
#54251=CARTESIAN_POINT('Ctrl Pts',(10.7155646400367,15.756906338373,-45.0306511771533));
#54252=CARTESIAN_POINT('Ctrl Pts',(10.7155646400367,30.3937787577631,-14.6368724193901));
#54253=CARTESIAN_POINT('Ctrl Pts',(10.7155646400367,45.0306511771533,15.756906338373));
#54254=CARTESIAN_POINT('Ctrl Pts',(10.7155646400367,14.6368724193901,30.3937787577631));
#54255=CARTESIAN_POINT('Ctrl Pts',(10.7155646400367,5.21305344074461,34.9320507901155));
#54256=CARTESIAN_POINT('Ctrl Pts',(10.7155646400367,-5.12517843764354,33.3429507899297));
#54257=CARTESIAN_POINT('Ctrl Pts',(9.82859575068344,-5.24839106585011,34.1445370466763));
#54258=CARTESIAN_POINT('Ctrl Pts',(9.82859575068344,-23.2306303080404,31.3804690010715));
#54259=CARTESIAN_POINT('Ctrl Pts',(9.82859575068344,-31.1244649977519,14.9887523668806));
#54260=CARTESIAN_POINT('Ctrl Pts',(9.82859575068344,-46.1132173646325,-16.1357126308712));
#54261=CARTESIAN_POINT('Ctrl Pts',(9.82859575068344,-14.9887523668806,-31.1244649977519));
#54262=CARTESIAN_POINT('Ctrl Pts',(9.82859575068344,16.1357126308712,-46.1132173646325));
#54263=CARTESIAN_POINT('Ctrl Pts',(9.82859575068344,31.1244649977519,-14.9887523668806));
#54264=CARTESIAN_POINT('Ctrl Pts',(9.82859575068344,46.1132173646325,16.1357126308712));
#54265=CARTESIAN_POINT('Ctrl Pts',(9.82859575068344,14.9887523668806,31.1244649977519));
#54266=CARTESIAN_POINT('Ctrl Pts',(9.82859575068344,5.33837864126793,35.771840046014));
#54267=CARTESIAN_POINT('Ctrl Pts',(9.82859575068344,-5.24839106585011,34.1445370466763));
#54268=CARTESIAN_POINT('Ctrl Pts',(8.97989469943246,-5.37602105757972,34.9748614120298));
#54269=CARTESIAN_POINT('Ctrl Pts',(8.97989469943246,-23.7955510841199,32.1435769609828));
#54270=CARTESIAN_POINT('Ctrl Pts',(8.97989469943246,-31.8813474709538,15.3532477553949));
#54271=CARTESIAN_POINT('Ctrl Pts',(8.97989469943246,-47.2345952263487,-16.5280997155588));
#54272=CARTESIAN_POINT('Ctrl Pts',(8.97989469943246,-15.3532477553949,-31.8813474709538));
#54273=CARTESIAN_POINT('Ctrl Pts',(8.97989469943246,16.5280997155588,-47.2345952263487));
#54274=CARTESIAN_POINT('Ctrl Pts',(8.97989469943246,31.8813474709538,-15.3532477553949));
#54275=CARTESIAN_POINT('Ctrl Pts',(8.97989469943246,47.2345952263487,16.5280997155588));
#54276=CARTESIAN_POINT('Ctrl Pts',(8.97989469943246,15.3532477553949,31.8813474709538));
#54277=CARTESIAN_POINT('Ctrl Pts',(8.97989469943246,5.46819694430327,36.6417370471983));
#54278=CARTESIAN_POINT('Ctrl Pts',(8.97989469943246,-5.37602105757972,34.9748614120298));
#54279=CARTESIAN_POINT('Ctrl Pts',(8.1713316609345,-5.50765762249487,35.8312514010853));
#54280=CARTESIAN_POINT('Ctrl Pts',(8.1713316609345,-24.3782059084644,32.9306404806214));
#54281=CARTESIAN_POINT('Ctrl Pts',(8.1713316609345,-32.6619900727951,15.7291854188016));
#54282=CARTESIAN_POINT('Ctrl Pts',(8.1713316609345,-48.3911754915967,-16.9328046539935));
#54283=CARTESIAN_POINT('Ctrl Pts',(8.1713316609345,-15.7291854188016,-32.6619900727951));
#54284=CARTESIAN_POINT('Ctrl Pts',(8.1713316609345,16.9328046539935,-48.3911754915967));
#54285=CARTESIAN_POINT('Ctrl Pts',(8.1713316609345,32.6619900727951,-15.7291854188016));
#54286=CARTESIAN_POINT('Ctrl Pts',(8.1713316609345,48.3911754915967,16.9328046539935));
#54287=CARTESIAN_POINT('Ctrl Pts',(8.1713316609345,15.7291854188016,32.6619900727951));
#54288=CARTESIAN_POINT('Ctrl Pts',(8.1713316609345,5.60209051620674,37.5389419401399));
#54289=CARTESIAN_POINT('Ctrl Pts',(8.1713316609345,-5.50765762249487,35.8312514010853));
#54290=CARTESIAN_POINT('Ctrl Pts',(7.40358438374929,-5.64301551373697,36.7118512790457));
#54291=CARTESIAN_POINT('Ctrl Pts',(7.40358438374929,-24.9773322104622,33.739954050605));
#54292=CARTESIAN_POINT('Ctrl Pts',(7.40358438374929,-33.4647012075554,16.1157507275363));
#54293=CARTESIAN_POINT('Ctrl Pts',(7.40358438374929,-49.5804519350917,-17.348950480019));
#54294=CARTESIAN_POINT('Ctrl Pts',(7.40358438374929,-16.1157507275363,-33.4647012075554));
#54295=CARTESIAN_POINT('Ctrl Pts',(7.40358438374929,17.348950480019,-49.5804519350917));
#54296=CARTESIAN_POINT('Ctrl Pts',(7.40358438374929,33.4647012075554,-16.1157507275363));
#54297=CARTESIAN_POINT('Ctrl Pts',(7.40358438374929,49.5804519350917,17.348950480019));
#54298=CARTESIAN_POINT('Ctrl Pts',(7.40358438374929,16.1157507275363,33.4647012075554));
#54299=CARTESIAN_POINT('Ctrl Pts',(7.40358438374929,5.73976921934981,38.4615105471143));
#54300=CARTESIAN_POINT('Ctrl Pts',(7.40358438374929,-5.64301551373697,36.7118512790457));
#54301=CARTESIAN_POINT('Ctrl Pts',(6.82198164612729,-5.75413848390819,37.4347856648684));
#54302=CARTESIAN_POINT('Ctrl Pts',(6.82198164612729,-25.4691889731139,34.4043654629813));
#54303=CARTESIAN_POINT('Ctrl Pts',(6.82198164612729,-34.1236923063789,16.4331041147498));
#54304=CARTESIAN_POINT('Ctrl Pts',(6.82198164612729,-50.5567964211288,-17.6905881916291));
#54305=CARTESIAN_POINT('Ctrl Pts',(6.82198164612729,-16.4331041147498,-34.1236923063789));
#54306=CARTESIAN_POINT('Ctrl Pts',(6.82198164612729,17.6905881916291,-50.5567964211288));
#54307=CARTESIAN_POINT('Ctrl Pts',(6.82198164612729,34.1236923063789,-16.4331041147498));
#54308=CARTESIAN_POINT('Ctrl Pts',(6.82198164612729,50.5567964211288,17.6905881916291));
#54309=CARTESIAN_POINT('Ctrl Pts',(6.82198164612729,16.4331041147498,34.1236923063789));
#54310=CARTESIAN_POINT('Ctrl Pts',(6.82198164612729,5.85279747564271,39.2188994429737));
#54311=CARTESIAN_POINT('Ctrl Pts',(6.82198164612729,-5.75413848390819,37.4347856648684));
#54312=CARTESIAN_POINT('Ctrl Pts',(6.40395249919757,-5.83903695291963,37.9871109173118));
#54313=CARTESIAN_POINT('Ctrl Pts',(6.40395249919757,-25.8449698405413,34.9119788899584));
#54314=CARTESIAN_POINT('Ctrl Pts',(6.40395249919757,-34.627164588447,16.6755635870669));
#54315=CARTESIAN_POINT('Ctrl Pts',(6.40395249919757,-51.3027281755139,-17.9516010013801));
#54316=CARTESIAN_POINT('Ctrl Pts',(6.40395249919757,-16.6755635870669,-34.627164588447));
#54317=CARTESIAN_POINT('Ctrl Pts',(6.40395249919757,17.9516010013801,-51.3027281755139));
#54318=CARTESIAN_POINT('Ctrl Pts',(6.40395249919757,34.627164588447,-16.6755635870669));
#54319=CARTESIAN_POINT('Ctrl Pts',(6.40395249919757,51.3027281755139,17.9516010013801));
#54320=CARTESIAN_POINT('Ctrl Pts',(6.40395249919757,16.6755635870669,34.627164588447));
#54321=CARTESIAN_POINT('Ctrl Pts',(6.40395249919757,5.93915159216349,39.7975481022532));
#54322=CARTESIAN_POINT('Ctrl Pts',(6.40395249919757,-5.83903695291963,37.9871109173118));
#54323=CARTESIAN_POINT('Ctrl Pts',(6.13331019225912,-5.89632479122585,38.3598092724512));
#54324=CARTESIAN_POINT('Ctrl Pts',(6.13331019225912,-26.0985394728612,35.2545065735001));
#54325=CARTESIAN_POINT('Ctrl Pts',(6.13331019225912,-34.9668979078181,16.8391705308393));
#54326=CARTESIAN_POINT('Ctrl Pts',(6.13331019225912,-51.8060684386574,-18.1277273769788));
#54327=CARTESIAN_POINT('Ctrl Pts',(6.13331019225912,-16.8391705308393,-34.9668979078181));
#54328=CARTESIAN_POINT('Ctrl Pts',(6.13331019225912,18.1277273769788,-51.8060684386574));
#54329=CARTESIAN_POINT('Ctrl Pts',(6.13331019225912,34.9668979078181,-16.8391705308393));
#54330=CARTESIAN_POINT('Ctrl Pts',(6.13331019225912,51.8060684386574,18.1277273769788));
#54331=CARTESIAN_POINT('Ctrl Pts',(6.13331019225912,16.8391705308393,34.9668979078181));
#54332=CARTESIAN_POINT('Ctrl Pts',(6.13331019225912,5.99742167314282,40.1880089811702));
#54333=CARTESIAN_POINT('Ctrl Pts',(6.13331019225912,-5.89632479122585,38.3598092724512));
#54334=CARTESIAN_POINT('Ctrl Pts',(6.,-5.92514092475929,38.5472788277168));
#54335=CARTESIAN_POINT('Ctrl Pts',(6.,-26.2260865509321,35.4268000961685));
#54336=CARTESIAN_POINT('Ctrl Pts',(6.,-35.1377858481943,16.9214658255848));
#54337=CARTESIAN_POINT('Ctrl Pts',(6.,-52.0592516737791,-18.2163200226096));
#54338=CARTESIAN_POINT('Ctrl Pts',(6.,-16.9214658255848,-35.1377858481943));
#54339=CARTESIAN_POINT('Ctrl Pts',(6.,18.2163200226096,-52.0592516737791));
#54340=CARTESIAN_POINT('Ctrl Pts',(6.,35.1377858481943,-16.9214658255848));
#54341=CARTESIAN_POINT('Ctrl Pts',(6.,52.0592516737791,18.2163200226096));
#54342=CARTESIAN_POINT('Ctrl Pts',(6.,16.9214658255848,35.1377858481943));
#54343=CARTESIAN_POINT('Ctrl Pts',(6.,6.0267318807567,40.3844131946844));
#54344=CARTESIAN_POINT('Ctrl Pts',(6.,-5.92514092475929,38.5472788277168));
#54345=CARTESIAN_POINT('Ctrl Pts',(24.5,-4.10202091932642,26.6865776070557));
#54346=CARTESIAN_POINT('Ctrl Pts',(23.5178991898112,-7.02888984535001,26.4061954211995));
#54347=CARTESIAN_POINT('Ctrl Pts',(22.3947886245986,-9.85513676624463,25.7451296467846));
#54348=CARTESIAN_POINT('Ctrl Pts',(21.1743874927566,-12.5415350592883,24.8143683028972));
#54349=CARTESIAN_POINT('Ctrl Pts',(20.503187179342,-14.0190094152206,24.3024650528661));
#54350=CARTESIAN_POINT('Ctrl Pts',(19.841179296638,-15.459956153512,23.6888889491766));
#54351=CARTESIAN_POINT('Ctrl Pts',(19.1295827650217,-16.8492605460919,23.0263961974636));
#54352=CARTESIAN_POINT('Ctrl Pts',(18.8261415870883,-17.4416919909654,22.7438940041273));
#54353=CARTESIAN_POINT('Ctrl Pts',(18.5104994276256,-18.0296748698289,22.4504043480946));
#54354=CARTESIAN_POINT('Ctrl Pts',(18.2016639423759,-18.5741854933314,22.1732398894808));
#54355=CARTESIAN_POINT('Ctrl Pts',(17.6747132403639,-19.5032570185016,21.700327892593));
#54356=CARTESIAN_POINT('Ctrl Pts',(17.2016343371005,-20.3165166452584,21.2459677585646));
#54357=CARTESIAN_POINT('Ctrl Pts',(16.8729352926472,-20.8613715162025,20.9390355645018));
#54358=CARTESIAN_POINT('Ctrl Pts',(16.6342454025482,-21.2570262996894,20.7161520091495));
#54359=CARTESIAN_POINT('Ctrl Pts',(16.5014949770667,-21.4700011946069,20.5942515068562));
#54360=CARTESIAN_POINT('Ctrl Pts',(16.3424569562979,-21.7223849124751,20.4503534012052));
#54361=CARTESIAN_POINT('Ctrl Pts',(15.993118510103,-22.2767638931664,20.1342708670068));
#54362=CARTESIAN_POINT('Ctrl Pts',(15.6312480487537,-22.8249648575983,19.8204138910798));
#54363=CARTESIAN_POINT('Ctrl Pts',(15.2503296894305,-23.3683243655452,19.5222267532057));
#54364=CARTESIAN_POINT('Ctrl Pts',(14.7484414179076,-24.0842409329261,19.1293430195787));
#54365=CARTESIAN_POINT('Ctrl Pts',(14.2669345517206,-24.7693427603849,18.7403316609859));
#54366=CARTESIAN_POINT('Ctrl Pts',(13.7912435751455,-25.4155597055059,18.3952128404075));
#54367=CARTESIAN_POINT('Ctrl Pts',(13.5533980868579,-25.7386681780664,18.2226534301183));
#54368=CARTESIAN_POINT('Ctrl Pts',(13.3161115657262,-26.0538393629016,18.0600012158979));
#54369=CARTESIAN_POINT('Ctrl Pts',(13.0766514227367,-26.3632568545648,17.9105174192254));
#54370=CARTESIAN_POINT('Ctrl Pts',(12.9188702359555,-26.5671332008995,17.8120219846653));
#54371=CARTESIAN_POINT('Ctrl Pts',(12.7601526360409,-26.768518589267,17.7192419542993));
#54372=CARTESIAN_POINT('Ctrl Pts',(12.5997389313808,-26.9681145831351,17.6332028310594));
#54373=CARTESIAN_POINT('Ctrl Pts',(12.5166971934814,-27.0714399083852,17.5886627567788));
#54374=CARTESIAN_POINT('Ctrl Pts',(12.4397215765388,-27.1663492636317,17.5490685135353));
#54375=CARTESIAN_POINT('Ctrl Pts',(12.3478597934844,-27.2783220449005,17.5045441701774));
#54376=CARTESIAN_POINT('Ctrl Pts',(11.9116121727781,-27.810075923262,17.2930999960328));
#54377=CARTESIAN_POINT('Ctrl Pts',(10.7144663992386,-29.3032420783634,16.6461921152493));
#54378=CARTESIAN_POINT('Ctrl Pts',(9.56604185022482,-30.6013366128143,16.6022989798071));
#54379=CARTESIAN_POINT('Ctrl Pts',(9.07284645450887,-31.1588083667446,16.5834489018267));
#54380=CARTESIAN_POINT('Ctrl Pts',(8.57333454993011,-31.7021782420111,16.6574399322426));
#54381=CARTESIAN_POINT('Ctrl Pts',(8.00348148263448,-32.3497632212541,16.8141041993546));
#54382=CARTESIAN_POINT('Ctrl Pts',(7.63919428966211,-32.7637417147262,16.9142542018388));
#54383=CARTESIAN_POINT('Ctrl Pts',(7.24388644384739,-33.2272501674787,17.0569857758551));
#54384=CARTESIAN_POINT('Ctrl Pts',(6.94254646282505,-33.5948793104207,17.1798573054043));
#54385=CARTESIAN_POINT('Ctrl Pts',(6.91433564865247,-33.6292959762769,17.19136027914));
#54386=CARTESIAN_POINT('Ctrl Pts',(6.88669635040544,-33.6631407630316,17.2027579696588));
#54387=CARTESIAN_POINT('Ctrl Pts',(6.85962514029879,-33.6964076011753,17.2140339107427));
#54388=CARTESIAN_POINT('Ctrl Pts',(6.44000062073739,-34.2120691071963,17.3888196458955));
#54389=CARTESIAN_POINT('Ctrl Pts',(6.15412442492901,-34.5726334242706,17.569202218668));
#54390=CARTESIAN_POINT('Ctrl Pts',(6.,-34.7703877941326,17.6640916167698));
#54391=CARTESIAN_POINT('Ctrl Pts',(2.09999999999999,-8.34942492151724,5.01979576159902));
#54392=CARTESIAN_POINT('Ctrl Pts',(2.73333333333333,-8.34942492151724,5.01979576159902));
#54393=CARTESIAN_POINT('Ctrl Pts',(3.3670066960941,-8.34945762015934,5.01975070676219));
#54394=CARTESIAN_POINT('Ctrl Pts',(4.12581290128969,-8.3494675953969,5.01973710194472));
#54395=CARTESIAN_POINT('Ctrl Pts',(4.38277322768255,-8.35014527570449,5.01863624946971));
#54396=CARTESIAN_POINT('Ctrl Pts',(4.88873771935076,-8.35315509347545,5.01376061458228));
#54397=CARTESIAN_POINT('Ctrl Pts',(5.76578794114311,-8.36010835560182,5.00252538661004));
#54398=CARTESIAN_POINT('Ctrl Pts',(6.49297690404802,-8.36003126626443,5.00271709005476));
#54399=CARTESIAN_POINT('Ctrl Pts',(7.02338209451756,-8.34858381308083,5.02100940896465));
#54400=CARTESIAN_POINT('Ctrl Pts',(7.14976392682211,-8.3458231106267,5.02554405062937));
#54401=CARTESIAN_POINT('Ctrl Pts',(7.39959333012189,-8.3400478083999,5.03523386697765));
#54402=CARTESIAN_POINT('Ctrl Pts',(7.71338818747182,-8.33207879519409,5.04890883922946));
#54403=CARTESIAN_POINT('Ctrl Pts',(8.08764188214564,-8.32084794494089,5.0682031434201));
#54404=CARTESIAN_POINT('Ctrl Pts',(8.58206241785991,-8.30304111738429,5.09831422701953));
#54405=CARTESIAN_POINT('Ctrl Pts',(9.18588787679093,-8.27425997957743,5.14525139206092));
#54406=CARTESIAN_POINT('Ctrl Pts',(9.64255639534934,-8.24198331627265,5.19457168720712));
#54407=CARTESIAN_POINT('Ctrl Pts',(10.3692081392539,-8.17902467196105,5.28739536504009));
#54408=CARTESIAN_POINT('Ctrl Pts',(11.102425634648,-8.09134598482829,5.42279242355537));
#54409=CARTESIAN_POINT('Ctrl Pts',(12.0425787397489,-7.9415154745789,5.64100401523642));
#54410=CARTESIAN_POINT('Ctrl Pts',(12.4996155489097,-7.8577884580503,5.755174313772));
#54411=CARTESIAN_POINT('Ctrl Pts',(13.0011661172537,-7.76088369919287,5.88085533234623));
#54412=CARTESIAN_POINT('Ctrl Pts',(13.5006127767821,-7.65247605468804,6.01885415512814));
#54413=CARTESIAN_POINT('Ctrl Pts',(14.4710726589074,-7.40389754548305,6.32617356312799));
#54414=CARTESIAN_POINT('Ctrl Pts',(15.1518142252861,-7.19020489438465,6.56953458941686));
#54415=CARTESIAN_POINT('Ctrl Pts',(15.8845569213207,-6.9432966915507,6.82188773029062));
#54416=CARTESIAN_POINT('Ctrl Pts',(16.3869773989622,-6.75786173757531,7.00426968060754));
#54417=CARTESIAN_POINT('Ctrl Pts',(17.3639381354626,-6.3463779015774,7.38519896132104));
#54418=CARTESIAN_POINT('Ctrl Pts',(18.0500099547399,-6.00535000373466,7.66464608496521));
#54419=CARTESIAN_POINT('Ctrl Pts',(18.7841565036792,-5.62040929877534,7.94279021781233));
#54420=CARTESIAN_POINT('Ctrl Pts',(19.2876849505228,-5.33554933752951,8.13708078860648));
#54421=CARTESIAN_POINT('Ctrl Pts',(20.2707836182184,-4.71473834446341,8.52038703318919));
#54422=CARTESIAN_POINT('Ctrl Pts',(20.9685349513319,-4.21244438509208,8.77731094000538));
#54423=CARTESIAN_POINT('Ctrl Pts',(22.65695724953,-2.95889425175503,9.31010852249438));
#54424=CARTESIAN_POINT('Ctrl Pts',(23.7241254823866,-2.00510513613211,9.54811629512881));
#54425=CARTESIAN_POINT('Ctrl Pts',(24.6950729185821,-0.969169964574942,
9.66847864460699));
#54426=CARTESIAN_POINT('Ctrl Pts',(2.09999999999999,-10.8626263234642,6.23008976872817));
#54427=CARTESIAN_POINT('Ctrl Pts',(2.73333333333333,-10.8626263234642,6.23008976872817));
#54428=CARTESIAN_POINT('Ctrl Pts',(3.36712916604075,-10.8626687927181,6.23002867096587));
#54429=CARTESIAN_POINT('Ctrl Pts',(4.1260789328716,-10.8626816890499,6.23001031043174));
#54430=CARTESIAN_POINT('Ctrl Pts',(4.38494073854913,-10.8635280023923,6.22857030785887));
#54431=CARTESIAN_POINT('Ctrl Pts',(4.89216306342126,-10.867275319152,6.22221170294779));
#54432=CARTESIAN_POINT('Ctrl Pts',(5.76874066410185,-10.8759106709847,6.20759670771725));
#54433=CARTESIAN_POINT('Ctrl Pts',(6.48939227720775,-10.8757765578405,6.20791193263853));
#54434=CARTESIAN_POINT('Ctrl Pts',(7.01204180322129,-10.8617170555104,6.23144086586232));
#54435=CARTESIAN_POINT('Ctrl Pts',(7.13830270328599,-10.858292565369,6.23733581247022));
#54436=CARTESIAN_POINT('Ctrl Pts',(7.38677643126479,-10.8511579895149,6.24989080196436));
#54437=CARTESIAN_POINT('Ctrl Pts',(7.69896900751756,-10.8413202385665,6.26761040631564));
#54438=CARTESIAN_POINT('Ctrl Pts',(8.07060760210473,-10.8274748483276,6.29258196555194));
#54439=CARTESIAN_POINT('Ctrl Pts',(8.56092958329594,-10.8055382261151,6.33151268282151));
#54440=CARTESIAN_POINT('Ctrl Pts',(9.1581881055872,-10.7701032006638,6.39210343890159));
#54441=CARTESIAN_POINT('Ctrl Pts',(9.60781844770696,-10.7304229027369,6.45557012594851));
#54442=CARTESIAN_POINT('Ctrl Pts',(10.3209483006796,-10.6531647380277,6.57470987900924));
#54443=CARTESIAN_POINT('Ctrl Pts',(11.042581596335,-10.5456407687268,6.74887792887924));
#54444=CARTESIAN_POINT('Ctrl Pts',(11.9743268683783,-10.3604778566151,7.03151955961449));
#54445=CARTESIAN_POINT('Ctrl Pts',(12.4289046542735,-10.2564876869773,7.17994113381094));
#54446=CARTESIAN_POINT('Ctrl Pts',(12.9286907133014,-10.135786957015,7.34363551094295));
#54447=CARTESIAN_POINT('Ctrl Pts',(13.4199991602706,-10.0021283089252,7.52177847665784));
#54448=CARTESIAN_POINT('Ctrl Pts',(14.3833044564643,-9.69353871566837,7.92135052907318));
#54449=CARTESIAN_POINT('Ctrl Pts',(15.0608942658284,-9.42683427492701,8.23929021623871));
#54450=CARTESIAN_POINT('Ctrl Pts',(15.7927655637968,-9.11698148114171,8.57033742089244));
#54451=CARTESIAN_POINT('Ctrl Pts',(16.2911221408769,-8.88573333710061,8.80857545235014));
#54452=CARTESIAN_POINT('Ctrl Pts',(17.2659436260203,-8.36948997402069,9.30918082924326));
#54453=CARTESIAN_POINT('Ctrl Pts',(17.951042142688,-7.93971093348247,9.67818466313474));
#54454=CARTESIAN_POINT('Ctrl Pts',(18.6848541385476,-7.45311339013388,10.0467837622568));
#54455=CARTESIAN_POINT('Ctrl Pts',(19.1879800656874,-7.09344722076858,10.3048160303236));
#54456=CARTESIAN_POINT('Ctrl Pts',(20.1723051379962,-6.30654681482803,10.8163737020384));
#54457=CARTESIAN_POINT('Ctrl Pts',(20.8704406678443,-5.66794248076931,11.1616568826984));
#54458=CARTESIAN_POINT('Ctrl Pts',(22.5587575563567,-4.07186834192525,11.8828606633097));
#54459=CARTESIAN_POINT('Ctrl Pts',(23.6292145427077,-2.85110598151754,12.2186869038546));
#54460=CARTESIAN_POINT('Ctrl Pts',(24.6070641578141,-1.51514224511533,12.4047064442659));
#54461=CARTESIAN_POINT('Ctrl Pts',(2.09999999999999,-15.8890291273581,8.65067778298648));
#54462=CARTESIAN_POINT('Ctrl Pts',(2.73333333333333,-15.8890291273581,8.65067778298648));
#54463=CARTESIAN_POINT('Ctrl Pts',(3.3673825055222,-15.889104504075,8.65057089971265));
#54464=CARTESIAN_POINT('Ctrl Pts',(4.12662168526103,-15.889127309897,8.65053895855418));
#54465=CARTESIAN_POINT('Ctrl Pts',(4.38928798294562,-15.890318506566,8.64840599244989));
#54466=CARTESIAN_POINT('Ctrl Pts',(4.89902245014287,-15.8955560337698,8.63905247688287));
#54467=CARTESIAN_POINT('Ctrl Pts',(5.77467110216829,-15.907556286625,8.61768036781575));
#54468=CARTESIAN_POINT('Ctrl Pts',(6.48222349628015,-15.9072667853389,8.61834812915088));
#54469=CARTESIAN_POINT('Ctrl Pts',(6.98946452110265,-15.8882256758818,8.65185633792884));
#54470=CARTESIAN_POINT('Ctrl Pts',(7.11548589692682,-15.8834783966492,8.66046288514499));
#54471=CARTESIAN_POINT('Ctrl Pts',(7.36126941213412,-15.8736712461814,8.67865495699402));
#54472=CARTESIAN_POINT('Ctrl Pts',(7.67029367856112,-15.8601635892604,8.70433206734693));
#54473=CARTESIAN_POINT('Ctrl Pts',(8.0367725352429,-15.8412062817442,8.74042252484053));
#54474=CARTESIAN_POINT('Ctrl Pts',(8.51906506082345,-15.8112406517118,8.79654161635137));
#54475=CARTESIAN_POINT('Ctrl Pts',(9.10358944465605,-15.7629482177986,8.88355963695649));
#54476=CARTESIAN_POINT('Ctrl Pts',(9.5400123194474,-15.7091485978985,8.97402106211602));
#54477=CARTESIAN_POINT('Ctrl Pts',(10.2287355379469,-15.6048805966226,9.14286649421513));
#54478=CARTESIAN_POINT('Ctrl Pts',(10.9322921746061,-15.4596505450725,9.39125917852511));
#54479=CARTESIAN_POINT('Ctrl Pts',(11.8534554375931,-15.2053258424165,9.80087093771465));
#54480=CARTESIAN_POINT('Ctrl Pts',(12.3052690270545,-15.0613611618861,10.0173156165896));
#54481=CARTESIAN_POINT('Ctrl Pts',(12.8031307179637,-14.8935321735672,10.2567539515269));
#54482=CARTESIAN_POINT('Ctrl Pts',(13.2871710515135,-14.7104718569604,10.5140864129075));
#54483=CARTESIAN_POINT('Ctrl Pts',(14.2485990096974,-14.2816356908812,11.0997389287419));
#54484=CARTESIAN_POINT('Ctrl Pts',(14.9265639642419,-13.9085020645968,11.5682553472289));
#54485=CARTESIAN_POINT('Ctrl Pts',(15.65866299345,-13.4730533863241,12.0571400248602));
#54486=CARTESIAN_POINT('Ctrl Pts',(16.1598143108985,-13.1477831760047,12.4105209936867));
#54487=CARTESIAN_POINT('Ctrl Pts',(17.1407487388018,-12.417186963142,13.156067730112));
#54488=CARTESIAN_POINT('Ctrl Pts',(17.8295851905423,-11.8071773596292,13.7066920314026));
#54489=CARTESIAN_POINT('Ctrl Pts',(18.5645530783256,-11.1166259020156,14.2565922786745));
#54490=CARTESIAN_POINT('Ctrl Pts',(19.0747524351397,-10.6010291281585,14.6469875368371));
#54491=CARTESIAN_POINT('Ctrl Pts',(20.0668395729403,-9.47382018883457,15.4190563401778));
#54492=CARTESIAN_POINT('Ctrl Pts',(20.7687912462459,-8.55849044800405,15.9418324548243));
#54493=CARTESIAN_POINT('Ctrl Pts',(22.4600869487331,-6.27367162967554,17.0380712303253));
#54494=CARTESIAN_POINT('Ctrl Pts',(23.5475381170851,-4.49961958864046,17.5738159147105));
#54495=CARTESIAN_POINT('Ctrl Pts',(24.5367404413918,-2.55107090700389,17.8863800997173));
#54496=CARTESIAN_POINT('Ctrl Pts',(2.09999999999999,-24.6852340341725,12.8867068079385));
#54497=CARTESIAN_POINT('Ctrl Pts',(2.73333333333333,-24.6852340341725,12.8867068079385));
#54498=CARTESIAN_POINT('Ctrl Pts',(3.36791107159354,-24.6853317546275,12.8865652847935));
#54499=CARTESIAN_POINT('Ctrl Pts',(4.12768121430416,-24.6853606115858,12.8865243203323));
#54500=CARTESIAN_POINT('Ctrl Pts',(4.39701762154762,-24.6871752442854,12.8831353414075));
#54501=CARTESIAN_POINT('Ctrl Pts',(4.91113197063761,-24.6950582823475,12.8684563166808));
#54502=CARTESIAN_POINT('Ctrl Pts',(5.7852670703077,-24.7129251351602,12.8352991234043));
#54503=CARTESIAN_POINT('Ctrl Pts',(6.46978616647,-24.7121107535044,12.8370651611017));
#54504=CARTESIAN_POINT('Ctrl Pts',(6.95073559623754,-24.6851250729823,12.8864227095011));
#54505=CARTESIAN_POINT('Ctrl Pts',(7.07635357803357,-24.6780765591886,12.8997472234176));
#54506=CARTESIAN_POINT('Ctrl Pts',(7.31756522858531,-24.6637419516586,12.9274971155078));
#54507=CARTESIAN_POINT('Ctrl Pts',(7.62128632811344,-24.6440033147104,12.9667017603524));
#54508=CARTESIAN_POINT('Ctrl Pts',(7.97917793444992,-24.6164746134198,13.0214934233426));
#54509=CARTESIAN_POINT('Ctrl Pts',(8.44847277450474,-24.573120133392,13.1063538137385));
#54510=CARTESIAN_POINT('Ctrl Pts',(9.01312641813064,-24.5036098535915,13.2370812402565));
#54511=CARTESIAN_POINT('Ctrl Pts',(9.43134912688994,-24.4266874344919,13.3717464360822));
#54512=CARTESIAN_POINT('Ctrl Pts',(10.0907921620889,-24.2778927786545,13.6225041072927));
#54513=CARTESIAN_POINT('Ctrl Pts',(10.7834912876056,-24.0671198126597,14.000653890148));
#54514=CARTESIAN_POINT('Ctrl Pts',(11.7034370264027,-23.6895856203247,14.6371266646603));
#54515=CARTESIAN_POINT('Ctrl Pts',(12.1558473466704,-23.4745906089699,14.9746304906823));
#54516=CARTESIAN_POINT('Ctrl Pts',(12.6542419042604,-23.2234646468753,15.348225695834));
#54517=CARTESIAN_POINT('Ctrl Pts',(13.1437462399789,-22.9481397930833,15.7534255158228));
#54518=CARTESIAN_POINT('Ctrl Pts',(14.1171132883844,-22.2987829221682,16.6787955360184));
#54519=CARTESIAN_POINT('Ctrl Pts',(14.8016574873343,-21.7325476271127,17.4179925894728));
#54520=CARTESIAN_POINT('Ctrl Pts',(15.5357648414539,-21.0744403383711,18.1847988319859));
#54521=CARTESIAN_POINT('Ctrl Pts',(16.0483420510548,-20.573614508204,18.7509903067964));
#54522=CARTESIAN_POINT('Ctrl Pts',(17.0412063199226,-19.4551142828868,19.9339578481721));
#54523=CARTESIAN_POINT('Ctrl Pts',(17.7361485053828,-18.5215259268316,20.8054593492918));
#54524=CARTESIAN_POINT('Ctrl Pts',(18.4726929142883,-17.4699774150895,21.6714660034558));
#54525=CARTESIAN_POINT('Ctrl Pts',(18.9926305583918,-16.670868714932,22.2983785648451));
#54526=CARTESIAN_POINT('Ctrl Pts',(19.9931796161569,-14.9373133436789,23.5255394018631));
#54527=CARTESIAN_POINT('Ctrl Pts',(20.6988341590712,-13.5316346811608,24.355867966199));
#54528=CARTESIAN_POINT('Ctrl Pts',(22.3924759398877,-10.0329126621697,26.0975343019239));
#54529=CARTESIAN_POINT('Ctrl Pts',(23.4934655270119,-7.27758194603014,26.9751716398332));
#54530=CARTESIAN_POINT('Ctrl Pts',(24.4911063137788,-4.25357930705334,27.4974711076497));
#54531=CARTESIAN_POINT('Ctrl Pts',(2.09999999999999,-30.9682375390399,15.9124418257614));
#54532=CARTESIAN_POINT('Ctrl Pts',(2.73333333333333,-30.9682375390399,15.9124418257614));
#54533=CARTESIAN_POINT('Ctrl Pts',(3.36829025256733,-30.9683301024836,15.9123139194918));
#54534=CARTESIAN_POINT('Ctrl Pts',(4.1284374497986,-30.9683565622462,15.9122787049611));
#54535=CARTESIAN_POINT('Ctrl Pts',(4.40254535554455,-30.970634683707,15.9079545360157));
#54536=CARTESIAN_POINT('Ctrl Pts',(4.91974554141507,-30.9804441635442,15.8893934640385));
#54537=CARTESIAN_POINT('Ctrl Pts',(5.79291553961598,-31.0024795572307,15.8478635012422));
#54538=CARTESIAN_POINT('Ctrl Pts',(6.46068624857462,-31.0010953179064,15.8508078920142));
#54539=CARTESIAN_POINT('Ctrl Pts',(6.92365522593866,-30.9690910431221,15.9101265761794));
#54540=CARTESIAN_POINT('Ctrl Pts',(7.04900195729302,-30.9604102911096,15.9267985760767));
#54541=CARTESIAN_POINT('Ctrl Pts',(7.28711491876453,-30.9429667627173,15.9611199296699));
#54542=CARTESIAN_POINT('Ctrl Pts',(7.58730945500939,-30.9189356421462,16.009664909088));
#54543=CARTESIAN_POINT('Ctrl Pts',(7.93961085376542,-30.8855807484087,16.0772177527489));
#54544=CARTESIAN_POINT('Ctrl Pts',(8.40082290028868,-30.8331543630746,16.1816268564623));
#54545=CARTESIAN_POINT('Ctrl Pts',(8.95405999645022,-30.7493484525957,16.3418922694593));
#54546=CARTESIAN_POINT('Ctrl Pts',(9.36434284862748,-30.6565656105899,16.5069296423345));
#54547=CARTESIAN_POINT('Ctrl Pts',(10.0148884847374,-30.4761334632112,16.8160554392504));
#54548=CARTESIAN_POINT('Ctrl Pts',(10.7127408890464,-30.2155593319315,17.2928070606343));
#54549=CARTESIAN_POINT('Ctrl Pts',(11.6387343709689,-29.7461959624163,18.0977624082062));
#54550=CARTESIAN_POINT('Ctrl Pts',(12.0933688355602,-29.4791056966195,18.5237540722142));
#54551=CARTESIAN_POINT('Ctrl Pts',(12.5933202684205,-29.1674178905854,18.9946082520247));
#54552=CARTESIAN_POINT('Ctrl Pts',(13.0908862957948,-28.8211456765741,19.5128785502266));
#54553=CARTESIAN_POINT('Ctrl Pts',(14.0727349416798,-28.0083559361138,20.6876432051089));
#54554=CARTESIAN_POINT('Ctrl Pts',(14.7612267225558,-27.301134448208,21.6223765758924));
#54555=CARTESIAN_POINT('Ctrl Pts',(15.4964710430934,-26.4824736348807,22.5876620437275));
#54556=CARTESIAN_POINT('Ctrl Pts',(16.01484268476,-25.8522730655872,23.3090056830889));
#54557=CARTESIAN_POINT('Ctrl Pts',(17.0124740776252,-24.452781473862,24.804932045947));
#54558=CARTESIAN_POINT('Ctrl Pts',(17.709978366144,-23.2858793778611,25.9050193793247));
#54559=CARTESIAN_POINT('Ctrl Pts',(18.4472345601431,-21.9749509058657,26.9953458912914));
#54560=CARTESIAN_POINT('Ctrl Pts',(18.9707204797144,-20.9713314847816,27.7907154941331));
#54561=CARTESIAN_POINT('Ctrl Pts',(19.9739933044595,-18.8024955852929,29.3401330613107));
#54562=CARTESIAN_POINT('Ctrl Pts',(20.6810262896676,-17.0452285236267,30.3879138141395));
#54563=CARTESIAN_POINT('Ctrl Pts',(22.3757441673503,-12.6765752760488,32.5850201604799));
#54564=CARTESIAN_POINT('Ctrl Pts',(23.4815899075194,-9.21962042180251,33.7021663443025));
#54565=CARTESIAN_POINT('Ctrl Pts',(24.4815088739376,-5.42882719120685,34.3692550812891));
#54566=CARTESIAN_POINT('Ctrl Pts',(2.09999999999999,-34.7380396419603,17.7278828364551));
#54567=CARTESIAN_POINT('Ctrl Pts',(2.73333333333333,-34.7380396419603,17.7278828364551));
#54568=CARTESIAN_POINT('Ctrl Pts',(3.36851999241306,-34.7381248546768,17.7277694819828));
#54569=CARTESIAN_POINT('Ctrl Pts',(4.12889275411719,-34.7381485955713,17.7277395939778));
#54570=CARTESIAN_POINT('Ctrl Pts',(4.40586721403073,-34.740711327236,17.7228406337032));
#54571=CARTESIAN_POINT('Ctrl Pts',(4.92489733234861,-34.7516913871972,17.7019190689149));
#54572=CARTESIAN_POINT('Ctrl Pts',(5.79754727458879,-34.7762173055544,17.655387207618));
#54573=CARTESIAN_POINT('Ctrl Pts',(6.45512262940898,-34.7744373975726,17.6591456413559));
#54574=CARTESIAN_POINT('Ctrl Pts',(6.90770633030733,-34.7396306906666,17.7240081296612));
#54575=CARTESIAN_POINT('Ctrl Pts',(7.03289870960102,-34.7299741346044,17.7426817178056));
#54576=CARTESIAN_POINT('Ctrl Pts',(7.2692358301988,-34.710703785389,17.7808672202825));
#54577=CARTESIAN_POINT('Ctrl Pts',(7.56744238493173,-34.6841437259206,17.8349214307925));
#54578=CARTESIAN_POINT('Ctrl Pts',(7.91665003948323,-34.6473728595804,17.9099709368762));
#54579=CARTESIAN_POINT('Ctrl Pts',(8.37355692634873,-34.5896133218137,18.0258905306332));
#54580=CARTESIAN_POINT('Ctrl Pts',(8.92113358743038,-34.497360835933,18.203630160046));
#54581=CARTESIAN_POINT('Ctrl Pts',(9.32837987631535,-34.3949235995297,18.387182191653));
#54582=CARTESIAN_POINT('Ctrl Pts',(9.97672036625888,-34.1947703440345,18.7327763273445));
#54583=CARTESIAN_POINT('Ctrl Pts',(10.6788811821633,-33.9029132211185,19.2712416755063));
#54584=CARTESIAN_POINT('Ctrl Pts',(11.6082688528039,-33.3775438321155,20.1785876628404));
#54585=CARTESIAN_POINT('Ctrl Pts',(12.064154115784,-33.0788815748098,20.6580339412667));
#54586=CARTESIAN_POINT('Ctrl Pts',(12.5649503363404,-32.7306110340746,21.1874574525754));
#54587=CARTESIAN_POINT('Ctrl Pts',(13.0665664254018,-32.3410506220515,21.7744538722713));
#54588=CARTESIAN_POINT('Ctrl Pts',(14.0523375976892,-31.4297559210954,23.0989321907902));
#54589=CARTESIAN_POINT('Ctrl Pts',(14.7427637262042,-30.6376034884511,24.1509958186388));
#54590=CARTESIAN_POINT('Ctrl Pts',(15.4785695663788,-29.7223267263288,25.2352714327783));
#54591=CARTESIAN_POINT('Ctrl Pts',(15.9996419749169,-29.0143486465837,26.0495423163302));
#54592=CARTESIAN_POINT('Ctrl Pts',(16.9994926423133,-27.4461241825516,27.7327496384012));
#54593=CARTESIAN_POINT('Ctrl Pts',(17.6981566854513,-26.1390088681491,28.9697268515409));
#54594=CARTESIAN_POINT('Ctrl Pts',(18.4357083126267,-24.6721941391514,30.1943963087492));
#54595=CARTESIAN_POINT('Ctrl Pts',(18.9608160431014,-23.5458848553488,31.0904778020446));
#54596=CARTESIAN_POINT('Ctrl Pts',(19.9653367025609,-21.1158182718772,32.8326764201553));
#54597=CARTESIAN_POINT('Ctrl Pts',(20.6729356218039,-19.1474864936212,34.0105320904367));
#54598=CARTESIAN_POINT('Ctrl Pts',(22.3680176960418,-14.2564897842765,36.4800421305849));
#54599=CARTESIAN_POINT('Ctrl Pts',(23.4757593035169,-10.3789662309951,37.7398907431838));
#54600=CARTESIAN_POINT('Ctrl Pts',(24.4767076204831,-6.12845803691562,38.4932334964498));
#54601=CARTESIAN_POINT('',(3.2,-33.4762280926097,17.1202264205697));
#54602=CARTESIAN_POINT('Ctrl Pts',(3.2,-33.4762280926097,17.1202264205697));
#54603=CARTESIAN_POINT('Ctrl Pts',(3.4517402013188,-32.7757491074893,16.7828935203276));
#54604=CARTESIAN_POINT('Ctrl Pts',(3.71840125361074,-32.0670044206292,16.4415800679211));
#54605=CARTESIAN_POINT('Ctrl Pts',(4.,-31.3543250987725,16.098371795166));
#54606=CARTESIAN_POINT('Ctrl Pts',(4.6281648118965,-29.76454503797,15.3327740683972));
#54607=CARTESIAN_POINT('Ctrl Pts',(5.32582967091579,-28.2030205776301,14.5138750276624));
#54608=CARTESIAN_POINT('Ctrl Pts',(6.03866108102417,-26.7368640118942,13.813540492213));
#54609=CARTESIAN_POINT('Ctrl Pts',(6.32798218053302,-26.1417863769365,13.529291573118));
#54610=CARTESIAN_POINT('Ctrl Pts',(6.61604116736837,-25.5687234927156,13.2688968345931));
#54611=CARTESIAN_POINT('Ctrl Pts',(6.89476148100328,-25.0250506156583,13.0435011857835));
#54612=CARTESIAN_POINT('Ctrl Pts',(7.65522892881283,-23.5416799927312,12.4285260820233));
#54613=CARTESIAN_POINT('Ctrl Pts',(8.35226709346248,-22.324236812765,11.9709302842019));
#54614=CARTESIAN_POINT('Ctrl Pts',(8.78926323736241,-21.5755931674142,11.7167440120742));
#54615=CARTESIAN_POINT('Ctrl Pts',(8.9903195773824,-21.231151795529,11.5997961573375));
#54616=CARTESIAN_POINT('Ctrl Pts',(9.18275521977661,-20.9067416215901,11.4960100244497));
#54617=CARTESIAN_POINT('Ctrl Pts',(9.37496045779525,-20.5859767684872,11.4009959127837));
#54618=CARTESIAN_POINT('Ctrl Pts',(9.48075233102288,-20.4094242716606,11.3486991025623));
#54619=CARTESIAN_POINT('Ctrl Pts',(9.58626090804149,-20.2343663629071,11.2992238752517));
#54620=CARTESIAN_POINT('Ctrl Pts',(9.69257910363365,-20.0586675915761,11.2524282472449));
#54621=CARTESIAN_POINT('Ctrl Pts',(10.0319880468435,-19.4977689234922,11.1030384409171));
#54622=CARTESIAN_POINT('Ctrl Pts',(10.3788056741065,-18.9297317699116,10.9818572797184));
#54623=CARTESIAN_POINT('Ctrl Pts',(10.775684908382,-18.293043816953,10.8706700722781));
#54624=CARTESIAN_POINT('Ctrl Pts',(10.8890930404452,-18.1111104094671,10.8388983583255));
#54625=CARTESIAN_POINT('Ctrl Pts',(11.0576203523027,-17.8415364545336,10.7938699917916));
#54626=CARTESIAN_POINT('Ctrl Pts',(11.2725125495735,-17.5031160652737,10.743205792085));
#54627=CARTESIAN_POINT('Ctrl Pts',(11.5968279595283,-16.9923718471319,10.666743356936));
#54628=CARTESIAN_POINT('Ctrl Pts',(12.0255678844699,-16.3252314956296,10.5807340258753));
#54629=CARTESIAN_POINT('Ctrl Pts',(12.532035905153,-15.5782338255957,10.4832582458773));
#54630=CARTESIAN_POINT('Ctrl Pts',(13.0988763177502,-14.7421919627351,10.3741630827162));
#54631=CARTESIAN_POINT('Ctrl Pts',(13.7495416919435,-13.7918088264638,10.3061345330427));
#54632=CARTESIAN_POINT('Ctrl Pts',(14.4398764943048,-12.8279168306252,10.2524861844184));
#54633=CARTESIAN_POINT('Ctrl Pts',(14.7901814039645,-12.3387974969788,10.2252627562297));
#54634=CARTESIAN_POINT('Ctrl Pts',(15.1459546153433,-11.8554473457044,10.1996815666194));
#54635=CARTESIAN_POINT('Ctrl Pts',(15.4570717747561,-11.4475484046093,10.172636394889));
#54636=CARTESIAN_POINT('Ctrl Pts',(15.7998231403801,-10.9981745437756,10.1428412863143));
#54637=CARTESIAN_POINT('Ctrl Pts',(16.0676294489035,-10.6509242977906,10.1275228717851));
#54638=CARTESIAN_POINT('Ctrl Pts',(16.3615307965769,-10.2740380103256,10.1136303748));
#54639=CARTESIAN_POINT('Ctrl Pts',(17.0296616018229,-9.41725616592929,10.0820483311278));
#54640=CARTESIAN_POINT('Ctrl Pts',(17.708469187171,-8.56731901604727,10.0713433202013));
#54641=CARTESIAN_POINT('Ctrl Pts',(18.4207032016838,-7.74709961718816,10.0374944043974));
#54642=CARTESIAN_POINT('Ctrl Pts',(18.829864204215,-7.27590365533518,10.0180490310472));
#54643=CARTESIAN_POINT('Ctrl Pts',(19.2113759272667,-6.83961046405605,10.0084432606969));
#54644=CARTESIAN_POINT('Ctrl Pts',(19.5701113607413,-6.43357233649932,9.99980987752349));
#54645=CARTESIAN_POINT('Ctrl Pts',(20.1215476021908,-5.80942395846933,9.98653892649964));
#54646=CARTESIAN_POINT('Ctrl Pts',(20.6514912601844,-5.2096335262144,9.97986911023992));
#54647=CARTESIAN_POINT('Ctrl Pts',(21.3979544325339,-4.42881997131726,9.93555336802176));
#54648=CARTESIAN_POINT('Ctrl Pts',(21.8107631282077,-3.99701484401668,9.91104589810155));
#54649=CARTESIAN_POINT('Ctrl Pts',(22.3076315955347,-3.48531200858995,9.87811544659317));
#54650=CARTESIAN_POINT('Ctrl Pts',(22.8472772295095,-2.92572478971589,9.83107499415808));
#54651=CARTESIAN_POINT('Ctrl Pts',(23.39531365686,-2.35743671154887,9.78330312337762));
#54652=CARTESIAN_POINT('Ctrl Pts',(23.9608264583112,-1.76507493700295,9.72269270625968));
#54653=CARTESIAN_POINT('Ctrl Pts',(24.5,-1.17476144568584,9.64284209699151));
#54654=CARTESIAN_POINT('Ctrl Pts',(2.79760018324017,-34.323788098568,17.5283403962136));
#54655=CARTESIAN_POINT('Ctrl Pts',(2.93205031708964,-34.0415378530154,17.3923990295756));
#54656=CARTESIAN_POINT('Ctrl Pts',(3.06670609136326,-33.7589461720905,17.256290336237));
#54657=CARTESIAN_POINT('Ctrl Pts',(3.20141516237076,-33.4762861111748,17.1201484566269));
#54658=CARTESIAN_POINT('Origin',(2.9,0.,0.));
#54659=CARTESIAN_POINT('Origin',(3.2,0.,0.));
#54660=CARTESIAN_POINT('Ctrl Pts',(2.1,-3.03642085633519,9.25886571362628));
#54661=CARTESIAN_POINT('Ctrl Pts',(2.73333333333333,-3.03642085633519,9.25886571362628));
#54662=CARTESIAN_POINT('Ctrl Pts',(3.36632482220385,-3.03636324782149,9.25886783371596));
#54663=CARTESIAN_POINT('Ctrl Pts',(4.12418518571929,-3.03634585734704,9.25886838619587));
#54664=CARTESIAN_POINT('Ctrl Pts',(4.3679354222169,-3.03750909441903,9.25849938516288));
#54665=CARTESIAN_POINT('Ctrl Pts',(4.86516885517288,-3.0428301752989,9.25682122204924));
#54666=CARTESIAN_POINT('Ctrl Pts',(5.74559105590866,-3.05539972951126,9.25287204039704));
#54667=CARTESIAN_POINT('Ctrl Pts',(6.51837844974244,-3.05559735374805,9.25281197487748));
#54668=CARTESIAN_POINT('Ctrl Pts',(7.10311570597879,-3.03287937787994,9.25984104765318));
#54669=CARTESIAN_POINT('Ctrl Pts',(7.23027107330381,-3.02779222743327,9.26147721945095));
#54670=CARTESIAN_POINT('Ctrl Pts',(7.4249517464998,-3.01943994533289,9.26424638408617));
#54671=CARTESIAN_POINT('Ctrl Pts',(7.61952199938249,-3.01043015254996,9.2672995518291));
#54672=CARTESIAN_POINT('Ctrl Pts',(8.01076939155846,-2.99081944883794,9.27400592468884));
#54673=CARTESIAN_POINT('Ctrl Pts',(8.60083990938693,-2.95480250579294,9.28632103618811));
#54674=CARTESIAN_POINT('Ctrl Pts',(9.25155102115583,-2.89826302827223,9.30424679722698));
#54675=CARTESIAN_POINT('Ctrl Pts',(9.76267543705633,-2.83990837348766,9.321312567219));
#54676=CARTESIAN_POINT('Ctrl Pts',(10.014174227857,-2.80574940848282,9.33079238677905));
#54677=CARTESIAN_POINT('Ctrl Pts',(10.7177547943786,-2.70119653739831,9.35897042938336));
#54678=CARTESIAN_POINT('Ctrl Pts',(11.8208662239638,-2.46633392199916,9.42626642479173));
#54679=CARTESIAN_POINT('Ctrl Pts',(12.8080235224918,-2.17401434547732,9.49797242406731));
#54680=CARTESIAN_POINT('Ctrl Pts',(13.5604138129135,-1.94092109890682,9.54355781467911));
#54681=CARTESIAN_POINT('Ctrl Pts',(14.1415326282582,-1.74098713062143,9.58078876510701));
#54682=CARTESIAN_POINT('Ctrl Pts',(15.2007206633323,-1.31387162315598,9.6515367181008));
#54683=CARTESIAN_POINT('Ctrl Pts',(15.9284925857039,-0.969988518465284,
9.69257775062039));
#54684=CARTESIAN_POINT('Ctrl Pts',(16.6747535574971,-0.611827371798453,
9.71611760998629));
#54685=CARTESIAN_POINT('Ctrl Pts',(17.2497597626852,-0.315563297197225,
9.72974158816072));
#54686=CARTESIAN_POINT('Ctrl Pts',(18.2984383463456,0.287775723800367,9.73535495662825));
#54687=CARTESIAN_POINT('Ctrl Pts',(19.0236515282951,0.752799571120926,9.7093944714803));
#54688=CARTESIAN_POINT('Ctrl Pts',(19.7681804380506,1.23052258053206,9.65365157938199));
#54689=CARTESIAN_POINT('Ctrl Pts',(20.3331320101339,1.61226392856985,9.598203157932));
#54690=CARTESIAN_POINT('Ctrl Pts',(21.3722761216913,2.37000412517729,9.44736748792574));
#54691=CARTESIAN_POINT('Ctrl Pts',(22.0962297345818,2.93224573984147,9.28523329835205));
#54692=CARTESIAN_POINT('Ctrl Pts',(23.2302247323429,3.79027058202878,8.97091205690245));
#54693=CARTESIAN_POINT('Ctrl Pts',(23.8854423668127,4.30028496502052,8.73255554778861));
#54694=CARTESIAN_POINT('Ctrl Pts',(24.5000000001022,4.7944580651727,8.44852886727892));
#54695=CARTESIAN_POINT('Ctrl Pts',(2.1,-3.9674280119859,13.3378745796554));
#54696=CARTESIAN_POINT('Ctrl Pts',(2.73333333333334,-3.9674280119859,13.3378745796554));
#54697=CARTESIAN_POINT('Ctrl Pts',(3.36613139261334,-3.96736212926572,13.3378808260227));
#54698=CARTESIAN_POINT('Ctrl Pts',(4.12377368580981,-3.96734259158422,13.3378825752465));
#54699=CARTESIAN_POINT('Ctrl Pts',(4.36467137386139,-3.96900709328001,13.3374064013275));
#54700=CARTESIAN_POINT('Ctrl Pts',(4.8600155516962,-3.97665156700167,13.3352304723138));
#54701=CARTESIAN_POINT('Ctrl Pts',(5.74114572251817,-3.99476856002092,13.3300899277835));
#54702=CARTESIAN_POINT('Ctrl Pts',(6.5237150074899,-3.99519388303041,13.3299818397575));
#54703=CARTESIAN_POINT('Ctrl Pts',(7.12009244527277,-3.96202698639281,13.3392674770816));
#54704=CARTESIAN_POINT('Ctrl Pts',(7.24739585324286,-3.95469236122976,13.3414037080991));
#54705=CARTESIAN_POINT('Ctrl Pts',(7.44368077169637,-3.94259427005441,13.3450474937973));
#54706=CARTESIAN_POINT('Ctrl Pts',(7.63959476887961,-3.92955381947168,13.3490688516567));
#54707=CARTESIAN_POINT('Ctrl Pts',(8.03421163923334,-3.90113824280286,13.3579171972697));
#54708=CARTESIAN_POINT('Ctrl Pts',(8.63054470873523,-3.84890354226684,13.3741911829931));
#54709=CARTESIAN_POINT('Ctrl Pts',(9.29110836512143,-3.76667328277033,13.3977994858214));
#54710=CARTESIAN_POINT('Ctrl Pts',(9.81209593588223,-3.68156553543029,13.4201847887225));
#54711=CARTESIAN_POINT('Ctrl Pts',(10.0692696198173,-3.63164870785884,13.4325883482395));
#54712=CARTESIAN_POINT('Ctrl Pts',(10.7901202392243,-3.47870991632635,13.4694216078752));
#54713=CARTESIAN_POINT('Ctrl Pts',(11.91641837421,-3.13571689561405,13.5575476160895));
#54714=CARTESIAN_POINT('Ctrl Pts',(12.9133332403102,-2.71251888458363,13.6487541609417));
#54715=CARTESIAN_POINT('Ctrl Pts',(13.6697365991946,-2.3766290909733,13.7045556427394));
#54716=CARTESIAN_POINT('Ctrl Pts',(14.2631492845408,-2.08523598290125,13.750506108406));
#54717=CARTESIAN_POINT('Ctrl Pts',(15.3329180253697,-1.46723682092391,13.8346922664385));
#54718=CARTESIAN_POINT('Ctrl Pts',(16.0654005693691,-0.972621989855104,
13.8792388488393));
#54719=CARTESIAN_POINT('Ctrl Pts',(16.8131010844738,-0.459790126624247,
13.8977377982197));
#54720=CARTESIAN_POINT('Ctrl Pts',(17.3939180876432,-0.0325415261246532,
13.905223318781));
#54721=CARTESIAN_POINT('Ctrl Pts',(18.4451545927817,0.83183807171203,13.8877537393552));
#54722=CARTESIAN_POINT('Ctrl Pts',(19.1720400984934,1.49522468250933,13.8310899003084));
#54723=CARTESIAN_POINT('Ctrl Pts',(19.9173951349631,2.17510085402637,13.7308930222181));
#54724=CARTESIAN_POINT('Ctrl Pts',(20.4826309364167,2.71876059724247,13.6358544771289));
#54725=CARTESIAN_POINT('Ctrl Pts',(21.5194122431661,3.79340188359948,13.388510786001));
#54726=CARTESIAN_POINT('Ctrl Pts',(22.2433206777627,4.58878559274361,13.1334972537449));
#54727=CARTESIAN_POINT('Ctrl Pts',(23.3780690493382,5.80072380280333,12.6475690238019));
#54728=CARTESIAN_POINT('Ctrl Pts',(24.0312127056184,6.51778005882525,12.2868361640544));
#54729=CARTESIAN_POINT('Ctrl Pts',(24.6419825553303,7.20914878794909,11.8621651263229));
#54730=CARTESIAN_POINT('Ctrl Pts',(2.1,-6.13977804183754,22.8555619337232));
#54731=CARTESIAN_POINT('Ctrl Pts',(2.73333333333333,-6.13977804183754,22.8555619337232));
#54732=CARTESIAN_POINT('Ctrl Pts',(3.365653360318,-6.13958582290045,22.8555736551316));
#54733=CARTESIAN_POINT('Ctrl Pts',(4.12277939961604,-6.13952862263624,22.8555767795658));
#54734=CARTESIAN_POINT('Ctrl Pts',(4.35701675178739,-6.14231565013462,22.854858979794));
#54735=CARTESIAN_POINT('Ctrl Pts',(4.84796106875134,-6.15528607005645,22.8515379397375));
#54736=CARTESIAN_POINT('Ctrl Pts',(5.73069923341384,-6.18633589313978,22.8436124669418));
#54737=CARTESIAN_POINT('Ctrl Pts',(6.53615142020775,-6.18749861931354,22.8433054821354));
#54738=CARTESIAN_POINT('Ctrl Pts',(7.15941690945266,-6.12850524487919,22.858168796905));
#54739=CARTESIAN_POINT('Ctrl Pts',(7.28706050168627,-6.11590359601848,22.861475915022));
#54740=CARTESIAN_POINT('Ctrl Pts',(7.4870444530628,-6.09485029109773,22.8672064973101));
#54741=CARTESIAN_POINT('Ctrl Pts',(7.68604635674693,-6.07220014505125,22.8735294015587));
#54742=CARTESIAN_POINT('Ctrl Pts',(8.08839747562535,-6.02271325537101,22.8874888199869));
#54743=CARTESIAN_POINT('Ctrl Pts',(8.69897241247564,-5.93135368058952,22.9132453728314));
#54744=CARTESIAN_POINT('Ctrl Pts',(9.38147318650496,-5.78652324369514,22.9506361922822));
#54745=CARTESIAN_POINT('Ctrl Pts',(9.92347837816972,-5.63556090051135,22.986091535273));
#54746=CARTESIAN_POINT('Ctrl Pts',(10.1922189143493,-5.54658888375171,23.0057398011073));
#54747=CARTESIAN_POINT('Ctrl Pts',(10.9470029906827,-5.27303275877381,23.064114912156));
#54748=CARTESIAN_POINT('Ctrl Pts',(12.1071873865115,-4.66475748602104,23.2025540475673));
#54749=CARTESIAN_POINT('Ctrl Pts',(13.1093438615391,-3.93318930439982,23.3383945039618));
#54750=CARTESIAN_POINT('Ctrl Pts',(13.8683635369228,-3.35571311089366,23.4172941333814));
#54751=CARTESIAN_POINT('Ctrl Pts',(14.4658066929412,-2.84996101905094,23.4828359475912));
#54752=CARTESIAN_POINT('Ctrl Pts',(15.5292048935208,-1.79474291067229,23.596261658863));
#54753=CARTESIAN_POINT('Ctrl Pts',(16.2561263101303,-0.953642037383936,
23.6478267525734));
#54754=CARTESIAN_POINT('Ctrl Pts',(17.0018250896354,-0.0807357451548354,
23.6536420885738));
#54755=CARTESIAN_POINT('Ctrl Pts',(17.5709881811724,0.63849429415504,23.6465481777418));
#54756=CARTESIAN_POINT('Ctrl Pts',(18.6067936674288,2.09172765883662,23.5771001185496));
#54757=CARTESIAN_POINT('Ctrl Pts',(19.3243419048038,3.20806192731327,23.4509787255064));
#54758=CARTESIAN_POINT('Ctrl Pts',(20.0666595174772,4.35754559455055,23.2485161668225));
#54759=CARTESIAN_POINT('Ctrl Pts',(20.6167887455572,5.25952111571729,23.0664267245431));
#54760=CARTESIAN_POINT('Ctrl Pts',(21.6393774029147,7.05499561655517,22.6043830858133));
#54761=CARTESIAN_POINT('Ctrl Pts',(22.3554860515227,8.38662026867344,22.139813592925));
#54762=CARTESIAN_POINT('Ctrl Pts',(23.4867391132867,10.4237640547879,21.261199459697));
#54763=CARTESIAN_POINT('Ctrl Pts',(24.125337196037,11.6072194078008,20.6279190418669));
#54764=CARTESIAN_POINT('Ctrl Pts',(24.727756995987,12.7519254968117,19.8878182601865));
#54765=CARTESIAN_POINT('Ctrl Pts',(2.1,-8.31212807168918,32.3732492877911));
#54766=CARTESIAN_POINT('Ctrl Pts',(2.73333333333334,-8.31212807168918,32.3732492877911));
#54767=CARTESIAN_POINT('Ctrl Pts',(3.3651165217007,-8.31196521408208,32.3732548809116));
#54768=CARTESIAN_POINT('Ctrl Pts',(4.12171258497796,-8.31191956967934,32.373255625749));
#54769=CARTESIAN_POINT('Ctrl Pts',(4.34927314647352,-8.31575317642587,32.3723152953323));
#54770=CARTESIAN_POINT('Ctrl Pts',(4.83587777455348,-8.33390159830587,32.3678881761052));
#54771=CARTESIAN_POINT('Ctrl Pts',(5.72001511869128,-8.37798521810356,32.3571598115706));
#54772=CARTESIAN_POINT('Ctrl Pts',(6.54876817834788,-8.38086727009316,32.3564666313068));
#54773=CARTESIAN_POINT('Ctrl Pts',(7.19754786253593,-8.29309470443329,32.3775894934029));
#54774=CARTESIAN_POINT('Ctrl Pts',(7.32550632174358,-8.27518440760661,32.3820760814367));
#54775=CARTESIAN_POINT('Ctrl Pts',(7.52896484904414,-8.24473551321405,32.3899925863444));
#54776=CARTESIAN_POINT('Ctrl Pts',(7.73081920990065,-8.21207597448873,32.3987063856483));
#54777=CARTESIAN_POINT('Ctrl Pts',(8.14025197937804,-8.1404418280831,32.4180128546022));
#54778=CARTESIAN_POINT('Ctrl Pts',(8.76332110590288,-8.00782017521505,32.4537361641667));
#54779=CARTESIAN_POINT('Ctrl Pts',(9.46279421342106,-7.79614249898192,32.5057982306959));
#54780=CARTESIAN_POINT('Ctrl Pts',(10.0176607623637,-7.57530053425566,32.5550946973183));
#54781=CARTESIAN_POINT('Ctrl Pts',(10.2919185676042,-7.44544358684942,32.5823081235974));
#54782=CARTESIAN_POINT('Ctrl Pts',(11.0596890924163,-7.04744605634131,32.6628595055625));
#54783=CARTESIAN_POINT('Ctrl Pts',(12.2113652017898,-6.18519408845136,32.8488994631672));
#54784=CARTESIAN_POINT('Ctrl Pts',(13.2034569104159,-5.16113729306093,33.0272278258128));
#54785=CARTESIAN_POINT('Ctrl Pts',(13.9587908471046,-4.34811174973568,33.1287391841076));
#54786=CARTESIAN_POINT('Ctrl Pts',(14.5428233206545,-3.64944819484762,33.2119379485251));
#54787=CARTESIAN_POINT('Ctrl Pts',(15.5915789891506,-2.18333872119813,33.354588850131));
#54788=CARTESIAN_POINT('Ctrl Pts',(16.3123176996232,-1.00843242986031,33.4154605432175));
#54789=CARTESIAN_POINT('Ctrl Pts',(17.0563515829208,0.220802504435864,33.4113265350998));
#54790=CARTESIAN_POINT('Ctrl Pts',(17.6162737851969,1.21359139026907,33.3925683370578));
#54791=CARTESIAN_POINT('Ctrl Pts',(18.645166902744,3.2420318553855,33.2784109512797));
#54792=CARTESIAN_POINT('Ctrl Pts',(19.3594014713778,4.80559392504864,33.0891039142606));
#54793=CARTESIAN_POINT('Ctrl Pts',(20.1008953939689,6.42413294926228,32.7902804240861));
#54794=CARTESIAN_POINT('Ctrl Pts',(20.6466151397584,7.67767483344647,32.5272511447639));
#54795=CARTESIAN_POINT('Ctrl Pts',(21.6663777991218,10.1933701488225,31.8609543508366));
#54796=CARTESIAN_POINT('Ctrl Pts',(22.3810344430405,12.0629280929144,31.194399788557));
#54797=CARTESIAN_POINT('Ctrl Pts',(23.5117469294374,14.9301557887008,29.9342669882141));
#54798=CARTESIAN_POINT('Ctrl Pts',(24.1480627906507,16.5833947234935,29.0351406353916));
#54799=CARTESIAN_POINT('Ctrl Pts',(24.7493903499091,18.1865024531276,27.9850142240257));
#54800=CARTESIAN_POINT('Ctrl Pts',(2.1,-9.55347094589012,37.8119277758299));
#54801=CARTESIAN_POINT('Ctrl Pts',(2.73333333333333,-9.55347094589012,37.8119277758299));
#54802=CARTESIAN_POINT('Ctrl Pts',(3.36479086716999,-9.55332620888327,37.8119309402221));
#54803=CARTESIAN_POINT('Ctrl Pts',(4.12108065676893,-9.55328738573655,37.8119307163399));
#54804=CARTESIAN_POINT('Ctrl Pts',(4.3448181830341,-9.55769178776168,37.8108695150359));
#54805=CARTESIAN_POINT('Ctrl Pts',(4.82897857397213,-9.57873699892895,37.8058249605254));
#54806=CARTESIAN_POINT('Ctrl Pts',(5.7138061276864,-9.63030673302427,37.7934862692131));
#54807=CARTESIAN_POINT('Ctrl Pts',(6.55611484843184,-9.63436371607534,37.7925312363998));
#54808=CARTESIAN_POINT('Ctrl Pts',(7.21874443048418,-9.52930083738139,37.8174231056462));
#54809=CARTESIAN_POINT('Ctrl Pts',(7.34686974636372,-9.50834537407352,37.8225859538797));
#54810=CARTESIAN_POINT('Ctrl Pts',(7.55219545109428,-9.47240667129618,37.8317783930218));
#54811=CARTESIAN_POINT('Ctrl Pts',(7.75555860205759,-9.43392187323299,37.8418815248632));
#54812=CARTESIAN_POINT('Ctrl Pts',(8.16870204156915,-9.34936587598233,37.8643012012295));
#54813=CARTESIAN_POINT('Ctrl Pts',(8.79805949449897,-9.19266019289524,37.905829016536));
#54814=CARTESIAN_POINT('Ctrl Pts',(9.50503273203101,-8.94227483367107,37.9663720914973));
#54815=CARTESIAN_POINT('Ctrl Pts',(10.0644372381433,-8.68184358810197,38.0234930381843));
#54816=CARTESIAN_POINT('Ctrl Pts',(10.3401591124554,-8.52923778582887,38.0548984873651));
#54817=CARTESIAN_POINT('Ctrl Pts',(11.1103063578917,-8.06278464620136,38.1475814285387));
#54818=CARTESIAN_POINT('Ctrl Pts',(12.254581323623,-7.06313343123591,38.3594886709139));
#54819=CARTESIAN_POINT('Ctrl Pts',(13.2428739922751,-5.87394568173444,38.5622360887224));
#54820=CARTESIAN_POINT('Ctrl Pts',(13.9964028454091,-4.92726867958817,38.6768476218439));
#54821=CARTESIAN_POINT('Ctrl Pts',(14.5753784070292,-4.12028262080844,38.7702148495551));
#54822=CARTESIAN_POINT('Ctrl Pts',(15.6192587771561,-2.41889470565338,38.9302475922307));
#54823=CARTESIAN_POINT('Ctrl Pts',(16.3373897865161,-1.05306307057831,38.9969282755714));
#54824=CARTESIAN_POINT('Ctrl Pts',(17.0806184187258,0.379671476043331,38.987618323965));
#54825=CARTESIAN_POINT('Ctrl Pts',(17.6369976627039,1.53007193924879,38.9625497856577));
#54826=CARTESIAN_POINT('Ctrl Pts',(18.6627888667656,3.88910869530589,38.8233284163515));
#54827=CARTESIAN_POINT('Ctrl Pts',(19.3754497970284,5.70863796723174,38.5983466101282));
#54828=CARTESIAN_POINT('Ctrl Pts',(20.1166099111039,7.59519646062446,38.2449529383188));
#54829=CARTESIAN_POINT('Ctrl Pts',(20.6599925696541,9.05087668442584,37.9357680733157));
#54830=CARTESIAN_POINT('Ctrl Pts',(21.6777820692419,11.9791501652495,37.152965907212));
#54831=CARTESIAN_POINT('Ctrl Pts',(22.3917974672498,14.1564098065562,36.3714296771662));
#54832=CARTESIAN_POINT('Ctrl Pts',(23.5225006119247,17.4981794009821,34.8939592200085));
#54833=CARTESIAN_POINT('Ctrl Pts',(24.157514841919,19.4205715247346,33.8431819361365));
#54834=CARTESIAN_POINT('Ctrl Pts',(24.7577717974218,21.2859250779863,32.6159836188887));
#54835=CARTESIAN_POINT('',(24.5,4.79445806514251,8.44852886740476));
#54836=CARTESIAN_POINT('Ctrl Pts',(24.5,4.79445806514251,8.44852886740476));
#54837=CARTESIAN_POINT('Ctrl Pts',(23.8274939346094,4.35568028974841,8.91358816488541));
#54838=CARTESIAN_POINT('Ctrl Pts',(23.3366347313997,4.04378531189072,9.23377527570042));
#54839=CARTESIAN_POINT('Ctrl Pts',(22.5855494187791,3.55891095582593,9.72812650348976));
#54840=CARTESIAN_POINT('Ctrl Pts',(22.2454144274676,3.33933172545618,9.95199741101992));
#54841=CARTESIAN_POINT('Ctrl Pts',(21.8382660749528,3.06477302734464,10.2233469033816));
#54842=CARTESIAN_POINT('Ctrl Pts',(21.3802156956953,2.74923897182448,10.5336111540776));
#54843=CARTESIAN_POINT('Ctrl Pts',(20.7694693297252,2.32851826843566,10.9473053069133));
#54844=CARTESIAN_POINT('Ctrl Pts',(20.1629003035507,1.90499719987852,11.3653835171637));
#54845=CARTESIAN_POINT('Ctrl Pts',(19.5574857571565,1.50134669736388,11.8035248325835));
#54846=CARTESIAN_POINT('Ctrl Pts',(18.641852941928,0.890863106926371,12.4661725480953));
#54847=CARTESIAN_POINT('Ctrl Pts',(17.7734813326701,0.243584198973207,13.1563618703622));
#54848=CARTESIAN_POINT('Ctrl Pts',(16.962125311809,-0.331821443170173,13.8621101827577));
#54849=CARTESIAN_POINT('Ctrl Pts',(16.8133360674514,-0.437341299426043,
13.9915327240442));
#54850=CARTESIAN_POINT('Ctrl Pts',(16.6656205372049,-0.541439795542996,
14.1222413658163));
#54851=CARTESIAN_POINT('Ctrl Pts',(16.5183901926363,-0.644331843442893,
14.2548376268699));
#54852=CARTESIAN_POINT('Ctrl Pts',(15.7264522885918,-1.19777830174949,14.9680601990961));
#54853=CARTESIAN_POINT('Ctrl Pts',(14.9462259717254,-1.80687549737941,15.7377680928373));
#54854=CARTESIAN_POINT('Ctrl Pts',(14.2963150412586,-2.29120527971764,16.427159456152));
#54855=CARTESIAN_POINT('Ctrl Pts',(13.9908350932594,-2.51885653127744,16.7511965325329));
#54856=CARTESIAN_POINT('Ctrl Pts',(13.7077063566188,-2.72603668208911,17.0631221045243));
#54857=CARTESIAN_POINT('Ctrl Pts',(13.4460198946299,-2.912853579393,17.3603809857102));
#54858=CARTESIAN_POINT('Ctrl Pts',(12.8373295399365,-3.34739513961885,18.0518138265595));
#54859=CARTESIAN_POINT('Ctrl Pts',(12.3530827399975,-3.71561728956872,18.6436933223557));
#54860=CARTESIAN_POINT('Ctrl Pts',(11.9770275677491,-3.99381285826312,19.1192007097534));
#54861=CARTESIAN_POINT('Ctrl Pts',(11.6553972423526,-4.2317463794219,19.5258899591599));
#54862=CARTESIAN_POINT('Ctrl Pts',(11.368420561198,-4.44137691516221,19.9029426948744));
#54863=CARTESIAN_POINT('Ctrl Pts',(11.0710856780973,-4.65123335112424,20.3088271733505));
#54864=CARTESIAN_POINT('Ctrl Pts',(10.8141787015422,-4.83255611390069,20.6595245187428));
#54865=CARTESIAN_POINT('Ctrl Pts',(10.5576802661712,-5.00811817493636,21.0215354696975));
#54866=CARTESIAN_POINT('Ctrl Pts',(10.2957959918397,-5.17851079664651,21.4059609250791));
#54867=CARTESIAN_POINT('Ctrl Pts',(9.71459276345219,-5.55666539216075,22.2591214148127));
#54868=CARTESIAN_POINT('Ctrl Pts',(9.09527967376231,-5.92026467566564,23.2374837564195));
#54869=CARTESIAN_POINT('Ctrl Pts',(8.43168033652699,-6.29835966306905,24.399171350721));
#54870=CARTESIAN_POINT('Ctrl Pts',(7.97964340480278,-6.55591401614932,25.1905007964946));
#54871=CARTESIAN_POINT('Ctrl Pts',(7.52291961074439,-6.81145492791075,26.0436998588172));
#54872=CARTESIAN_POINT('Ctrl Pts',(7.10363554125516,-7.05116144768124,26.8754977861791));
#54873=CARTESIAN_POINT('Ctrl Pts',(6.5632779955574,-7.36008619855196,27.9474876833705));
#54874=CARTESIAN_POINT('Ctrl Pts',(6.08559840023997,-7.60156228988461,28.9826246131377));
#54875=CARTESIAN_POINT('Ctrl Pts',(5.61708670830474,-7.83933188747728,30.0695190297804));
#54876=CARTESIAN_POINT('Ctrl Pts',(5.04102956504787,-8.13168078185986,31.4059067943778));
#54877=CARTESIAN_POINT('Ctrl Pts',(4.50102820503747,-8.40458357383467,32.7783233096991));
#54878=CARTESIAN_POINT('Ctrl Pts',(4.,-8.71775829923914,34.1504314334527));
#54879=CARTESIAN_POINT('Ctrl Pts',(3.72183418897114,-8.89162975120532,34.9122120382685));
#54880=CARTESIAN_POINT('Ctrl Pts',(3.45538353518229,-9.06631722055977,35.6775678488616));
#54881=CARTESIAN_POINT('Ctrl Pts',(3.2,-9.24182505978395,36.4465179346992));
#54882=CARTESIAN_POINT('',(24.5,14.1269463268952,23.0093326169409));
#54883=CARTESIAN_POINT('Ctrl Pts',(24.5,14.1269463268952,23.0093326169409));
#54884=CARTESIAN_POINT('Ctrl Pts',(24.5,13.4659464214661,21.9617493509785));
#54885=CARTESIAN_POINT('Ctrl Pts',(24.5,12.8153888814878,20.9324081809094));
#54886=CARTESIAN_POINT('Ctrl Pts',(24.5,10.1230771830749,16.6815116258866));
#54887=CARTESIAN_POINT('Ctrl Pts',(24.5,7.25732475029689,12.1733125527324));
#54888=CARTESIAN_POINT('Ctrl Pts',(24.5,4.79445806514251,8.44852886740475));
#54889=CARTESIAN_POINT('',(10.2670750393577,-7.59968099677391,33.2963779888109));
#54890=CARTESIAN_POINT('Ctrl Pts',(10.2670750393577,-7.59968099677391,33.2963779888109));
#54891=CARTESIAN_POINT('Ctrl Pts',(11.2293198185888,-6.94998678548836,32.5415114357085));
#54892=CARTESIAN_POINT('Ctrl Pts',(12.092802582344,-6.1285541721914,32.0055482292145));
#54893=CARTESIAN_POINT('Ctrl Pts',(14.3080979519049,-3.73267662114747,30.7914887306174));
#54894=CARTESIAN_POINT('Ctrl Pts',(14.8952017874601,-3.00279024948747,30.5262846241022));
#54895=CARTESIAN_POINT('Ctrl Pts',(17.0803363586062,0.164443307829025,29.4613521690468));
#54896=CARTESIAN_POINT('Ctrl Pts',(17.6922811489506,1.12977118340571,29.1445663219268));
#54897=CARTESIAN_POINT('Ctrl Pts',(19.0755427322033,3.49373927319035,28.3603783727572));
#54898=CARTESIAN_POINT('Ctrl Pts',(20.2687424742408,5.60613398516095,27.6263721986722));
#54899=CARTESIAN_POINT('Ctrl Pts',(22.3267279388309,9.72640384774287,25.7483075490095));
#54900=CARTESIAN_POINT('Ctrl Pts',(23.4192562717209,11.8964803423963,24.5951094752949));
#54901=CARTESIAN_POINT('Ctrl Pts',(24.5,14.1269463268952,23.0093326169409));
#54902=CARTESIAN_POINT('Ctrl Pts',(6.,-9.62277221548328,37.7942092772018));
#54903=CARTESIAN_POINT('Ctrl Pts',(7.51604047332548,-9.13953643716897,35.6914341219625));
#54904=CARTESIAN_POINT('Ctrl Pts',(9.08449301626627,-8.31972209498318,34.2861963730775));
#54905=CARTESIAN_POINT('Ctrl Pts',(9.8624969752411,-7.86293097600567,33.6206016235852));
#54906=CARTESIAN_POINT('Ctrl Pts',(10.0667253012217,-7.73495433668603,33.4535493442768));
#54907=CARTESIAN_POINT('Ctrl Pts',(10.2670750393577,-7.59968099677391,33.2963779888109));
#54908=CARTESIAN_POINT('Origin',(24.5,-1.89142793862867,8.2868872535455));
#54909=CARTESIAN_POINT('',(24.5,6.80662575089405,6.93067919103514));
#54910=CARTESIAN_POINT('Ctrl Pts',(24.5,6.80662575089405,6.93067919103514));
#54911=CARTESIAN_POINT('Ctrl Pts',(24.5,6.60260497657294,7.13104816180033));
#54912=CARTESIAN_POINT('Ctrl Pts',(24.5,6.38964036397032,7.322503105027));
#54913=CARTESIAN_POINT('Ctrl Pts',(24.5,5.7372524804206,7.85873653774361));
#54914=CARTESIAN_POINT('Ctrl Pts',(24.5,5.27749333642741,8.17441104304659));
#54915=CARTESIAN_POINT('Ctrl Pts',(24.5,4.79445806514251,8.44852886740476));
#54916=CARTESIAN_POINT('',(24.5,18.3068383223113,19.8458980809827));
#54917=CARTESIAN_POINT('Ctrl Pts',(24.5,6.80662575089405,6.93067919103514));
#54918=CARTESIAN_POINT('Ctrl Pts',(24.5,9.62249333717013,10.1909289822772));
#54919=CARTESIAN_POINT('Ctrl Pts',(24.5,13.4561052459601,14.4744049170257));
#54920=CARTESIAN_POINT('Ctrl Pts',(24.5,18.3068383223113,19.8458980809827));
#54921=CARTESIAN_POINT('Origin',(24.5,0.,0.));
#54922=CARTESIAN_POINT('Ctrl Pts',(24.5,18.3068385298747,19.845897889516));
#54923=CARTESIAN_POINT('Ctrl Pts',(24.5,7.85498547538757,29.4872044845456));
#54924=CARTESIAN_POINT('Ctrl Pts',(24.5,-6.00806521682049,26.3230536289092));
#54925=CARTESIAN_POINT('Ctrl Pts',(24.5,-32.3311188457297,20.3149884120888));
#54926=CARTESIAN_POINT('Ctrl Pts',(24.5,-26.3230536289092,-6.00806521682049));
#54927=CARTESIAN_POINT('Ctrl Pts',(24.5,-20.3149884120888,-32.3311188457297));
#54928=CARTESIAN_POINT('Ctrl Pts',(24.5,6.00806521682049,-26.3230536289092));
#54929=CARTESIAN_POINT('Ctrl Pts',(24.5,32.3311188457297,-20.3149884120888));
#54930=CARTESIAN_POINT('Ctrl Pts',(24.5,26.3230536289092,6.00806521682049));
#54931=CARTESIAN_POINT('Ctrl Pts',(24.5,24.4602079634702,14.1697253493454));
#54932=CARTESIAN_POINT('Ctrl Pts',(24.5,18.3068385298747,19.845897889516));
#54933=CARTESIAN_POINT('Ctrl Pts',(24.3078118955742,18.3290687603783,19.8699970196806));
#54934=CARTESIAN_POINT('Ctrl Pts',(24.3078118955742,7.86452388571633,29.5230111778492));
#54935=CARTESIAN_POINT('Ctrl Pts',(24.3078118955742,-6.01536088802186,26.3550180529563));
#54936=CARTESIAN_POINT('Ctrl Pts',(24.3078118955742,-32.3703789409781,20.3396571649344));
#54937=CARTESIAN_POINT('Ctrl Pts',(24.3078118955742,-26.3550180529563,-6.01536088802186));
#54938=CARTESIAN_POINT('Ctrl Pts',(24.3078118955742,-20.3396571649344,-32.3703789409781));
#54939=CARTESIAN_POINT('Ctrl Pts',(24.3078118955742,6.01536088802186,-26.3550180529563));
#54940=CARTESIAN_POINT('Ctrl Pts',(24.3078118955742,32.3703789409781,-20.3396571649344));
#54941=CARTESIAN_POINT('Ctrl Pts',(24.3078118955742,26.3550180529563,6.01536088802186));
#54942=CARTESIAN_POINT('Ctrl Pts',(24.3078118955742,24.4899103099625,14.1869318298732));
#54943=CARTESIAN_POINT('Ctrl Pts',(24.3078118955742,18.3290687603783,19.8699970196806));
#54944=CARTESIAN_POINT('Ctrl Pts',(23.9225830034177,18.376353041482,19.9212564991933));
#54945=CARTESIAN_POINT('Ctrl Pts',(23.9225830034177,7.88481233370136,29.5991729500489));
#54946=CARTESIAN_POINT('Ctrl Pts',(23.9225830034177,-6.03087897128555,26.4230072180579));
#54947=CARTESIAN_POINT('Ctrl Pts',(23.9225830034177,-32.4538861893435,20.3921282467724));
#54948=CARTESIAN_POINT('Ctrl Pts',(23.9225830034177,-26.4230072180579,-6.03087897128555));
#54949=CARTESIAN_POINT('Ctrl Pts',(23.9225830034177,-20.3921282467724,-32.4538861893435));
#54950=CARTESIAN_POINT('Ctrl Pts',(23.9225830034177,6.03087897128555,-26.4230072180579));
#54951=CARTESIAN_POINT('Ctrl Pts',(23.9225830034177,32.4538861893435,-20.3921282467724));
#54952=CARTESIAN_POINT('Ctrl Pts',(23.9225830034177,26.4230072180579,6.03087897128555));
#54953=CARTESIAN_POINT('Ctrl Pts',(23.9225830034177,24.5530879770028,14.2235304635197));
#54954=CARTESIAN_POINT('Ctrl Pts',(23.9225830034177,18.376353041482,19.9212564991933));
#54955=CARTESIAN_POINT('Ctrl Pts',(23.3421815947946,18.4557508948393,20.007329345021));
#54956=CARTESIAN_POINT('Ctrl Pts',(23.3421815947946,7.91887987539518,29.7270607190791));
#54957=CARTESIAN_POINT('Ctrl Pts',(23.3421815947946,-6.05693630938179,26.5371718756275));
#54958=CARTESIAN_POINT('Ctrl Pts',(23.3421815947946,-32.5941081850093,20.4802355662457));
#54959=CARTESIAN_POINT('Ctrl Pts',(23.3421815947946,-26.5371718756275,-6.05693630938179));
#54960=CARTESIAN_POINT('Ctrl Pts',(23.3421815947946,-20.4802355662457,-32.5941081850093));
#54961=CARTESIAN_POINT('Ctrl Pts',(23.3421815947946,6.05693630938179,-26.5371718756275));
#54962=CARTESIAN_POINT('Ctrl Pts',(23.3421815947946,32.5941081850093,-20.4802355662457));
#54963=CARTESIAN_POINT('Ctrl Pts',(23.3421815947946,26.5371718756275,6.05693630938179));
#54964=CARTESIAN_POINT('Ctrl Pts',(23.3421815947946,24.6591733615329,14.2849854096353));
#54965=CARTESIAN_POINT('Ctrl Pts',(23.3421815947946,18.4557508948393,20.007329345021));
#54966=CARTESIAN_POINT('Ctrl Pts',(22.5631762070947,18.5786269363992,20.140535598514));
#54967=CARTESIAN_POINT('Ctrl Pts',(22.5631762070947,7.97160277018397,29.9249797075388));
#54968=CARTESIAN_POINT('Ctrl Pts',(22.5631762070947,-6.09726262078022,26.7138529899778));
#54969=CARTESIAN_POINT('Ctrl Pts',(22.5631762070947,-32.811115610758,20.6165903691975));
#54970=CARTESIAN_POINT('Ctrl Pts',(22.5631762070947,-26.7138529899778,-6.09726262078022));
#54971=CARTESIAN_POINT('Ctrl Pts',(22.5631762070947,-20.6165903691975,-32.811115610758));
#54972=CARTESIAN_POINT('Ctrl Pts',(22.5631762070947,6.09726262078022,-26.7138529899778));
#54973=CARTESIAN_POINT('Ctrl Pts',(22.5631762070947,32.811115610758,-20.6165903691975));
#54974=CARTESIAN_POINT('Ctrl Pts',(22.5631762070947,26.7138529899778,6.09726262078022));
#54975=CARTESIAN_POINT('Ctrl Pts',(22.5631762070947,24.823351000691,14.3800930251898));
#54976=CARTESIAN_POINT('Ctrl Pts',(22.5631762070947,18.5786269363992,20.140535598514));
#54977=CARTESIAN_POINT('Ctrl Pts',(21.5808622776984,18.7610722387808,20.3383191117939));
#54978=CARTESIAN_POINT('Ctrl Pts',(21.5808622776984,8.049885276359,30.2188481398075));
#54979=CARTESIAN_POINT('Ctrl Pts',(21.5808622776984,-6.15713878527593,26.9761876072355));
#54980=CARTESIAN_POINT('Ctrl Pts',(21.5808622776984,-33.1333263925114,20.8190488219595));
#54981=CARTESIAN_POINT('Ctrl Pts',(21.5808622776984,-26.9761876072355,-6.15713878527593));
#54982=CARTESIAN_POINT('Ctrl Pts',(21.5808622776984,-20.8190488219595,-33.1333263925114));
#54983=CARTESIAN_POINT('Ctrl Pts',(21.5808622776984,6.15713878527593,-26.9761876072355));
#54984=CARTESIAN_POINT('Ctrl Pts',(21.5808622776984,33.1333263925114,-20.8190488219595));
#54985=CARTESIAN_POINT('Ctrl Pts',(21.5808622776984,26.9761876072355,6.15713878527593));
#54986=CARTESIAN_POINT('Ctrl Pts',(21.5808622776984,25.0671205642303,14.521308004598));
#54987=CARTESIAN_POINT('Ctrl Pts',(21.5808622776984,18.7610722387808,20.3383191117939));
#54988=CARTESIAN_POINT('Ctrl Pts',(20.5902243197586,18.9731487726588,20.5682249597772));
#54989=CARTESIAN_POINT('Ctrl Pts',(20.5902243197586,8.14088176876611,30.5604442111678));
#54990=CARTESIAN_POINT('Ctrl Pts',(20.5902243197586,-6.22673953280078,27.2811284065763));
#54991=CARTESIAN_POINT('Ctrl Pts',(20.5902243197586,-33.5078679393771,21.0543888737755));
#54992=CARTESIAN_POINT('Ctrl Pts',(20.5902243197586,-27.2811284065763,-6.22673953280078));
#54993=CARTESIAN_POINT('Ctrl Pts',(20.5902243197586,-21.0543888737755,-33.5078679393771));
#54994=CARTESIAN_POINT('Ctrl Pts',(20.5902243197586,6.22673953280078,-27.2811284065763));
#54995=CARTESIAN_POINT('Ctrl Pts',(20.5902243197586,33.5078679393771,-21.0543888737755));
#54996=CARTESIAN_POINT('Ctrl Pts',(20.5902243197586,27.2811284065763,6.22673953280078));
#54997=CARTESIAN_POINT('Ctrl Pts',(20.5902243197586,25.3504811299752,14.6854579332265));
#54998=CARTESIAN_POINT('Ctrl Pts',(20.5902243197586,18.9731487726588,20.5682249597772));
#54999=CARTESIAN_POINT('Ctrl Pts',(19.591895069338,19.2158583309824,20.831339156335));
#55000=CARTESIAN_POINT('Ctrl Pts',(19.591895069338,8.24502209055126,30.9513815302994));
#55001=CARTESIAN_POINT('Ctrl Pts',(19.591895069338,-6.30639363871178,27.6301158469569));
#55002=CARTESIAN_POINT('Ctrl Pts',(19.591895069338,-33.9365094856687,21.3237222082451));
#55003=CARTESIAN_POINT('Ctrl Pts',(19.591895069338,-27.6301158469569,-6.30639363871178));
#55004=CARTESIAN_POINT('Ctrl Pts',(19.591895069338,-21.3237222082451,-33.9365094856687));
#55005=CARTESIAN_POINT('Ctrl Pts',(19.591895069338,6.30639363871178,-27.6301158469569));
#55006=CARTESIAN_POINT('Ctrl Pts',(19.591895069338,33.9365094856687,-21.3237222082451));
#55007=CARTESIAN_POINT('Ctrl Pts',(19.591895069338,27.6301158469569,6.30639363871178));
#55008=CARTESIAN_POINT('Ctrl Pts',(19.591895069338,25.6747712176182,14.8733182115315));
#55009=CARTESIAN_POINT('Ctrl Pts',(19.591895069338,19.2158583309824,20.831339156335));
#55010=CARTESIAN_POINT('Ctrl Pts',(18.5871162949016,19.4903525092225,21.1289101117858));
#55011=CARTESIAN_POINT('Ctrl Pts',(18.5871162949016,8.36280036120327,31.3935149959097));
#55012=CARTESIAN_POINT('Ctrl Pts',(18.5871162949016,-6.3964790415962,28.0248057855197));
#55013=CARTESIAN_POINT('Ctrl Pts',(18.5871162949016,-34.4212848271159,21.6283267439235));
#55014=CARTESIAN_POINT('Ctrl Pts',(18.5871162949016,-28.0248057855197,-6.3964790415962));
#55015=CARTESIAN_POINT('Ctrl Pts',(18.5871162949016,-21.6283267439235,-34.4212848271159));
#55016=CARTESIAN_POINT('Ctrl Pts',(18.5871162949016,6.3964790415962,-28.0248057855197));
#55017=CARTESIAN_POINT('Ctrl Pts',(18.5871162949016,34.4212848271159,-21.6283267439235));
#55018=CARTESIAN_POINT('Ctrl Pts',(18.5871162949016,28.0248057855197,6.3964790415962));
#55019=CARTESIAN_POINT('Ctrl Pts',(18.5871162949016,26.041529501609,15.085780189022));
#55020=CARTESIAN_POINT('Ctrl Pts',(18.5871162949016,19.4903525092225,21.1289101117858));
#55021=CARTESIAN_POINT('Ctrl Pts',(17.577868433379,19.7977977061578,21.4622022842733));
#55022=CARTESIAN_POINT('Ctrl Pts',(17.577868433379,8.49471705192315,31.8887233507017));
#55023=CARTESIAN_POINT('Ctrl Pts',(17.577868433379,-6.49737853829363,28.4668753648014));
#55024=CARTESIAN_POINT('Ctrl Pts',(17.577868433379,-34.964253903095,21.9694968265077));
#55025=CARTESIAN_POINT('Ctrl Pts',(17.577868433379,-28.4668753648014,-6.49737853829363));
#55026=CARTESIAN_POINT('Ctrl Pts',(17.577868433379,-21.9694968265077,-34.964253903095));
#55027=CARTESIAN_POINT('Ctrl Pts',(17.577868433379,6.49737853829363,-28.4668753648014));
#55028=CARTESIAN_POINT('Ctrl Pts',(17.577868433379,34.964253903095,-21.9694968265077));
#55029=CARTESIAN_POINT('Ctrl Pts',(17.577868433379,28.4668753648014,6.49737853829363));
#55030=CARTESIAN_POINT('Ctrl Pts',(17.577868433379,26.4523144354541,15.3237466731552));
#55031=CARTESIAN_POINT('Ctrl Pts',(17.577868433379,19.7977977061578,21.4622022842733));
#55032=CARTESIAN_POINT('Ctrl Pts',(16.5668667015923,20.1391691218662,21.8322728591294));
#55033=CARTESIAN_POINT('Ctrl Pts',(16.5668667015923,8.64119059555145,32.4385773696654));
#55034=CARTESIAN_POINT('Ctrl Pts',(16.5668667015923,-6.60941217672811,28.9577268063763));
#55035=CARTESIAN_POINT('Ctrl Pts',(16.5668667015923,-35.5671389831044,22.3483146296482));
#55036=CARTESIAN_POINT('Ctrl Pts',(16.5668667015923,-28.9577268063763,-6.60941217672811));
#55037=CARTESIAN_POINT('Ctrl Pts',(16.5668667015923,-22.3483146296482,-35.5671389831044));
#55038=CARTESIAN_POINT('Ctrl Pts',(16.5668667015923,6.60941217672811,-28.9577268063763));
#55039=CARTESIAN_POINT('Ctrl Pts',(16.5668667015923,35.5671389831044,-22.3483146296482));
#55040=CARTESIAN_POINT('Ctrl Pts',(16.5668667015923,28.9577268063763,6.60941217672811));
#55041=CARTESIAN_POINT('Ctrl Pts',(16.5668667015923,26.9084290074696,15.5879724811674));
#55042=CARTESIAN_POINT('Ctrl Pts',(16.5668667015923,20.1391691218662,21.8322728591294));
#55043=CARTESIAN_POINT('Ctrl Pts',(15.5576189940876,20.5150087935408,22.239709442716));
#55044=CARTESIAN_POINT('Ctrl Pts',(15.5576189940876,8.80245356606713,33.0439501233491));
#55045=CARTESIAN_POINT('Ctrl Pts',(15.5576189940876,-6.7327578464244,29.4981394951766));
#55046=CARTESIAN_POINT('Ctrl Pts',(15.5576189940876,-36.230897341601,22.7653816487522));
#55047=CARTESIAN_POINT('Ctrl Pts',(15.5576189940876,-29.4981394951766,-6.7327578464244));
#55048=CARTESIAN_POINT('Ctrl Pts',(15.5576189940876,-22.7653816487522,-36.230897341601));
#55049=CARTESIAN_POINT('Ctrl Pts',(15.5576189940876,6.7327578464244,-29.4981394951766));
#55050=CARTESIAN_POINT('Ctrl Pts',(15.5576189940876,36.230897341601,-22.7653816487522));
#55051=CARTESIAN_POINT('Ctrl Pts',(15.5576189940876,29.4981394951766,6.7327578464244));
#55052=CARTESIAN_POINT('Ctrl Pts',(15.5576189940876,27.4105974466067,15.8788771567249));
#55053=CARTESIAN_POINT('Ctrl Pts',(15.5576189940876,20.5150087935408,22.239709442716));
#55054=CARTESIAN_POINT('Ctrl Pts',(14.5544447688713,20.9251959536421,22.6843811145439));
#55055=CARTESIAN_POINT('Ctrl Pts',(14.5544447688713,8.97845414527848,33.7046470889725));
#55056=CARTESIAN_POINT('Ctrl Pts',(14.5544447688713,-6.86737591305397,30.0879397818628));
#55057=CARTESIAN_POINT('Ctrl Pts',(14.5544447688713,-36.9553156949167,23.2205638688088));
#55058=CARTESIAN_POINT('Ctrl Pts',(14.5544447688713,-30.0879397818628,-6.86737591305397));
#55059=CARTESIAN_POINT('Ctrl Pts',(14.5544447688713,-23.2205638688088,-36.9553156949167));
#55060=CARTESIAN_POINT('Ctrl Pts',(14.5544447688713,6.86737591305397,-30.0879397818628));
#55061=CARTESIAN_POINT('Ctrl Pts',(14.5544447688713,36.9553156949167,-23.2205638688088));
#55062=CARTESIAN_POINT('Ctrl Pts',(14.5544447688713,30.0879397818628,6.86737591305397));
#55063=CARTESIAN_POINT('Ctrl Pts',(14.5544447688713,27.9586583924468,16.1963672242196));
#55064=CARTESIAN_POINT('Ctrl Pts',(14.5544447688713,20.9251959536421,22.6843811145439));
#55065=CARTESIAN_POINT('Ctrl Pts',(13.5625963827217,21.3685644590621,23.1650236936344));
#55066=CARTESIAN_POINT('Ctrl Pts',(13.5625963827217,9.16869197168609,34.4187899356465));
#55067=CARTESIAN_POINT('Ctrl Pts',(13.5625963827217,-7.012883663685,30.7254508915224));
#55068=CARTESIAN_POINT('Ctrl Pts',(13.5625963827217,-37.7383345552074,23.7125672278374));
#55069=CARTESIAN_POINT('Ctrl Pts',(13.5625963827217,-30.7254508915224,-7.012883663685));
#55070=CARTESIAN_POINT('Ctrl Pts',(13.5625963827217,-23.7125672278374,-37.7383345552074));
#55071=CARTESIAN_POINT('Ctrl Pts',(13.5625963827217,7.012883663685,-30.7254508915224));
#55072=CARTESIAN_POINT('Ctrl Pts',(13.5625963827217,37.7383345552074,-23.7125672278374));
#55073=CARTESIAN_POINT('Ctrl Pts',(13.5625963827217,30.7254508915224,7.012883663685));
#55074=CARTESIAN_POINT('Ctrl Pts',(13.5625963827217,28.5510537330912,16.5395400740865));
#55075=CARTESIAN_POINT('Ctrl Pts',(13.5625963827217,21.3685644590621,23.1650236936344));
#55076=CARTESIAN_POINT('Ctrl Pts',(12.5880795783847,21.8428970524859,23.679233517433));
#55077=CARTESIAN_POINT('Ctrl Pts',(12.5880795783847,9.37221567818334,35.1828072810307));
#55078=CARTESIAN_POINT('Ctrl Pts',(12.5880795783847,-7.16855342343642,31.4074846721918));
#55079=CARTESIAN_POINT('Ctrl Pts',(12.5880795783847,-38.5760380956282,24.2389312487553));
#55080=CARTESIAN_POINT('Ctrl Pts',(12.5880795783847,-31.4074846721918,-7.16855342343642));
#55081=CARTESIAN_POINT('Ctrl Pts',(12.5880795783847,-24.2389312487553,-38.5760380956282));
#55082=CARTESIAN_POINT('Ctrl Pts',(12.5880795783847,7.16855342343642,-31.4074846721918));
#55083=CARTESIAN_POINT('Ctrl Pts',(12.5880795783847,38.5760380956282,-24.2389312487553));
#55084=CARTESIAN_POINT('Ctrl Pts',(12.5880795783847,31.4074846721918,7.16855342343642));
#55085=CARTESIAN_POINT('Ctrl Pts',(12.5880795783847,29.1848209376287,16.9066795210254));
#55086=CARTESIAN_POINT('Ctrl Pts',(12.5880795783847,21.8428970524859,23.679233517433));
#55087=CARTESIAN_POINT('Ctrl Pts',(11.6370973936883,22.3454091248114,24.2239918742266));
#55088=CARTESIAN_POINT('Ctrl Pts',(11.6370973936883,9.58783046185459,35.9922138974944));
#55089=CARTESIAN_POINT('Ctrl Pts',(11.6370973936883,-7.33347131998334,32.1300371876035));
#55090=CARTESIAN_POINT('Ctrl Pts',(11.6370973936883,-39.4635085075868,24.7965658676202));
#55091=CARTESIAN_POINT('Ctrl Pts',(11.6370973936883,-32.1300371876035,-7.33347131998334));
#55092=CARTESIAN_POINT('Ctrl Pts',(11.6370973936883,-24.7965658676202,-39.4635085075868));
#55093=CARTESIAN_POINT('Ctrl Pts',(11.6370973936883,7.33347131998334,-32.1300371876035));
#55094=CARTESIAN_POINT('Ctrl Pts',(11.6370973936883,39.4635085075868,-24.7965658676202));
#55095=CARTESIAN_POINT('Ctrl Pts',(11.6370973936883,32.1300371876035,7.33347131998334));
#55096=CARTESIAN_POINT('Ctrl Pts',(11.6370973936883,29.856239422758,17.2956302422525));
#55097=CARTESIAN_POINT('Ctrl Pts',(11.6370973936883,22.3454091248114,24.2239918742266));
#55098=CARTESIAN_POINT('Ctrl Pts',(10.7155646400367,22.8730721573722,24.7960156372148));
#55099=CARTESIAN_POINT('Ctrl Pts',(10.7155646400367,9.81423686457129,36.8421316872136));
#55100=CARTESIAN_POINT('Ctrl Pts',(10.7155646400367,-7.5066434330687,32.8887537885844));
#55101=CARTESIAN_POINT('Ctrl Pts',(10.7155646400367,-40.3953972216531,25.3821103555157));
#55102=CARTESIAN_POINT('Ctrl Pts',(10.7155646400367,-32.8887537885844,-7.5066434330687));
#55103=CARTESIAN_POINT('Ctrl Pts',(10.7155646400367,-25.3821103555157,-40.3953972216531));
#55104=CARTESIAN_POINT('Ctrl Pts',(10.7155646400367,7.5066434330687,-32.8887537885844));
#55105=CARTESIAN_POINT('Ctrl Pts',(10.7155646400367,40.3953972216531,-25.3821103555157));
#55106=CARTESIAN_POINT('Ctrl Pts',(10.7155646400367,32.8887537885844,7.5066434330687));
#55107=CARTESIAN_POINT('Ctrl Pts',(10.7155646400367,30.5612627117334,17.7040481258859));
#55108=CARTESIAN_POINT('Ctrl Pts',(10.7155646400367,22.8730721573722,24.7960156372148));
#55109=CARTESIAN_POINT('Ctrl Pts',(9.82859575068344,23.4229557116635,25.392128005376));
#55110=CARTESIAN_POINT('Ctrl Pts',(9.82859575068344,10.0501775118362,37.7278405321141));
#55111=CARTESIAN_POINT('Ctrl Pts',(9.82859575068344,-7.68710803106292,33.6794208535527));
#55112=CARTESIAN_POINT('Ctrl Pts',(9.82859575068344,-41.3665288846156,25.9923128224897));
#55113=CARTESIAN_POINT('Ctrl Pts',(9.82859575068344,-33.6794208535527,-7.68710803106292));
#55114=CARTESIAN_POINT('Ctrl Pts',(9.82859575068344,-25.9923128224897,-41.3665288846156));
#55115=CARTESIAN_POINT('Ctrl Pts',(9.82859575068344,7.68710803106292,-33.6794208535527));
#55116=CARTESIAN_POINT('Ctrl Pts',(9.82859575068344,41.3665288846156,-25.9923128224897));
#55117=CARTESIAN_POINT('Ctrl Pts',(9.82859575068344,33.6794208535527,7.68710803106292));
#55118=CARTESIAN_POINT('Ctrl Pts',(9.82859575068344,31.2959753750754,18.1296649753334));
#55119=CARTESIAN_POINT('Ctrl Pts',(9.82859575068344,23.4229557116635,25.392128005376));
#55120=CARTESIAN_POINT('Ctrl Pts',(8.97989469943246,23.9925534429024,26.00961192505));
#55121=CARTESIAN_POINT('Ctrl Pts',(8.97989469943246,10.2945769966732,38.6453034106753));
#55122=CARTESIAN_POINT('Ctrl Pts',(8.97989469943246,-7.87404256435504,34.4984345571934));
#55123=CARTESIAN_POINT('Ctrl Pts',(8.97989469943246,-42.3724771215484,26.6243919928384));
#55124=CARTESIAN_POINT('Ctrl Pts',(8.97989469943246,-34.4984345571934,-7.87404256435504));
#55125=CARTESIAN_POINT('Ctrl Pts',(8.97989469943246,-26.6243919928384,-42.3724771215484));
#55126=CARTESIAN_POINT('Ctrl Pts',(8.97989469943246,7.87404256435504,-34.4984345571934));
#55127=CARTESIAN_POINT('Ctrl Pts',(8.97989469943246,42.3724771215484,-26.6243919928384));
#55128=CARTESIAN_POINT('Ctrl Pts',(8.97989469943246,34.4984345571934,7.87404256435504));
#55129=CARTESIAN_POINT('Ctrl Pts',(8.97989469943246,32.057028625143,18.5705408479257));
#55130=CARTESIAN_POINT('Ctrl Pts',(8.97989469943246,23.9925534429024,26.00961192505));
#55131=CARTESIAN_POINT('Ctrl Pts',(8.1713316609345,24.5800320418402,26.6464799603347));
#55132=CARTESIAN_POINT('Ctrl Pts',(8.1713316609345,10.5466486940461,39.5915673736694));
#55133=CARTESIAN_POINT('Ctrl Pts',(8.1713316609345,-8.06684536480278,35.3431588191374));
#55134=CARTESIAN_POINT('Ctrl Pts',(8.1713316609345,-43.4100041839401,27.2763134543346));
#55135=CARTESIAN_POINT('Ctrl Pts',(8.1713316609345,-35.3431588191374,-8.06684536480278));
#55136=CARTESIAN_POINT('Ctrl Pts',(8.1713316609345,-27.2763134543346,-43.4100041839401));
#55137=CARTESIAN_POINT('Ctrl Pts',(8.1713316609345,8.06684536480278,-35.3431588191374));
#55138=CARTESIAN_POINT('Ctrl Pts',(8.1713316609345,43.4100041839401,-27.2763134543346));
#55139=CARTESIAN_POINT('Ctrl Pts',(8.1713316609345,35.3431588191374,8.06684536480278));
#55140=CARTESIAN_POINT('Ctrl Pts',(8.1713316609345,32.8419729332853,19.0252567390383));
#55141=CARTESIAN_POINT('Ctrl Pts',(8.1713316609345,24.5800320418402,26.6464799603347));
#55142=CARTESIAN_POINT('Ctrl Pts',(7.40358438374929,25.1841184850965,27.3013520645346));
#55143=CARTESIAN_POINT('Ctrl Pts',(7.40358438374929,10.8058463829268,40.5645819359366));
#55144=CARTESIAN_POINT('Ctrl Pts',(7.40358438374929,-8.26509864276547,36.2117631833691));
#55145=CARTESIAN_POINT('Ctrl Pts',(7.40358438374929,-44.4768618261345,27.9466645406036));
#55146=CARTESIAN_POINT('Ctrl Pts',(7.40358438374929,-36.2117631833691,-8.26509864276547));
#55147=CARTESIAN_POINT('Ctrl Pts',(7.40358438374929,-27.9466645406036,-44.4768618261345));
#55148=CARTESIAN_POINT('Ctrl Pts',(7.40358438374929,8.26509864276547,-36.2117631833691));
#55149=CARTESIAN_POINT('Ctrl Pts',(7.40358438374929,44.4768618261345,-27.9466645406036));
#55150=CARTESIAN_POINT('Ctrl Pts',(7.40358438374929,36.2117631833691,8.26509864276547));
#55151=CARTESIAN_POINT('Ctrl Pts',(7.40358438374929,33.6491073822974,19.4928273124192));
#55152=CARTESIAN_POINT('Ctrl Pts',(7.40358438374929,25.1841184850965,27.3013520645346));
#55153=CARTESIAN_POINT('Ctrl Pts',(6.82198164612729,25.6800473090374,27.8389737180133));
#55154=CARTESIAN_POINT('Ctrl Pts',(6.82198164612729,11.0186364669452,41.3633847776977));
#55155=CARTESIAN_POINT('Ctrl Pts',(6.82198164612729,-8.42785600320625,36.9248497716085));
#55156=CARTESIAN_POINT('Ctrl Pts',(6.82198164612729,-45.3527057748147,28.4969937684022));
#55157=CARTESIAN_POINT('Ctrl Pts',(6.82198164612729,-36.9248497716085,-8.42785600320625));
#55158=CARTESIAN_POINT('Ctrl Pts',(6.82198164612729,-28.4969937684022,-45.3527057748147));
#55159=CARTESIAN_POINT('Ctrl Pts',(6.82198164612729,8.42785600320625,-36.9248497716085));
#55160=CARTESIAN_POINT('Ctrl Pts',(6.82198164612729,45.3527057748147,-28.4969937684022));
#55161=CARTESIAN_POINT('Ctrl Pts',(6.82198164612729,36.9248497716085,8.42785600320625));
#55162=CARTESIAN_POINT('Ctrl Pts',(6.82198164612729,34.3117298306725,19.8766825158504));
#55163=CARTESIAN_POINT('Ctrl Pts',(6.82198164612729,25.6800473090374,27.8389737180133));
#55164=CARTESIAN_POINT('Ctrl Pts',(6.40395249919757,26.0589392503377,28.2497191761072));
#55165=CARTESIAN_POINT('Ctrl Pts',(6.40395249919757,11.1812090865047,41.9736738853683));
#55166=CARTESIAN_POINT('Ctrl Pts',(6.40395249919757,-8.55220338791415,37.4696512606331));
#55167=CARTESIAN_POINT('Ctrl Pts',(6.40395249919757,-46.0218546485472,28.9174478727189));
#55168=CARTESIAN_POINT('Ctrl Pts',(6.40395249919757,-37.4696512606331,-8.55220338791415));
#55169=CARTESIAN_POINT('Ctrl Pts',(6.40395249919757,-28.9174478727189,-46.0218546485472));
#55170=CARTESIAN_POINT('Ctrl Pts',(6.40395249919757,8.55220338791415,-37.4696512606331));
#55171=CARTESIAN_POINT('Ctrl Pts',(6.40395249919757,46.0218546485472,-28.9174478727189));
#55172=CARTESIAN_POINT('Ctrl Pts',(6.40395249919757,37.4696512606331,8.55220338791415));
#55173=CARTESIAN_POINT('Ctrl Pts',(6.40395249919757,34.8179764807844,20.1699496868337));
#55174=CARTESIAN_POINT('Ctrl Pts',(6.40395249919757,26.0589392503377,28.2497191761072));
#55175=CARTESIAN_POINT('Ctrl Pts',(6.13331019225912,26.3146081748953,28.5268822352565));
#55176=CARTESIAN_POINT('Ctrl Pts',(6.13331019225912,11.2909099333019,42.3854851244564));
#55177=CARTESIAN_POINT('Ctrl Pts',(6.13331019225912,-8.63611058850204,37.8372727263161));
#55178=CARTESIAN_POINT('Ctrl Pts',(6.13331019225912,-46.4733833148181,29.201162137814));
#55179=CARTESIAN_POINT('Ctrl Pts',(6.13331019225912,-37.8372727263161,-8.63611058850204));
#55180=CARTESIAN_POINT('Ctrl Pts',(6.13331019225912,-29.201162137814,-46.4733833148181));
#55181=CARTESIAN_POINT('Ctrl Pts',(6.13331019225912,8.63611058850204,-37.8372727263161));
#55182=CARTESIAN_POINT('Ctrl Pts',(6.13331019225912,46.4733833148181,-29.201162137814));
#55183=CARTESIAN_POINT('Ctrl Pts',(6.13331019225912,37.8372727263161,8.63611058850204));
#55184=CARTESIAN_POINT('Ctrl Pts',(6.13331019225912,35.1595818898379,20.3678406790677));
#55185=CARTESIAN_POINT('Ctrl Pts',(6.13331019225912,26.3146081748953,28.5268822352565));
#55186=CARTESIAN_POINT('Ctrl Pts',(6.,26.4432112098191,28.666296951523));
#55187=CARTESIAN_POINT('Ctrl Pts',(6.,11.3460901311154,42.5926286998992));
#55188=CARTESIAN_POINT('Ctrl Pts',(6.,-8.67831642429626,38.0221885750911));
#55189=CARTESIAN_POINT('Ctrl Pts',(6.,-46.7005049993874,29.3438721507949));
#55190=CARTESIAN_POINT('Ctrl Pts',(6.,-38.0221885750911,-8.67831642429626));
#55191=CARTESIAN_POINT('Ctrl Pts',(6.,-29.3438721507949,-46.7005049993874));
#55192=CARTESIAN_POINT('Ctrl Pts',(6.,8.67831642429626,-38.0221885750911));
#55193=CARTESIAN_POINT('Ctrl Pts',(6.,46.7005049993874,-29.3438721507949));
#55194=CARTESIAN_POINT('Ctrl Pts',(6.,38.0221885750911,8.67831642429626));
#55195=CARTESIAN_POINT('Ctrl Pts',(6.,35.3314115027902,20.4673810601656));
#55196=CARTESIAN_POINT('Ctrl Pts',(6.,26.4432112098191,28.666296951523));
#55197=CARTESIAN_POINT('Ctrl Pts',(24.5,18.3068383223113,19.8458980809827));
#55198=CARTESIAN_POINT('Ctrl Pts',(23.5178991898112,16.2627537755328,21.9594009189012));
#55199=CARTESIAN_POINT('Ctrl Pts',(22.3947886245986,13.9837756084006,23.7568819701794));
#55200=CARTESIAN_POINT('Ctrl Pts',(21.1743874927566,11.5811351476418,25.2768725242511));
#55201=CARTESIAN_POINT('Ctrl Pts',(20.503187179342,10.2597228773583,26.1128420343255));
#55202=CARTESIAN_POINT('Ctrl Pts',(19.8411792966381,8.88159416625748,26.8568611155666));
#55203=CARTESIAN_POINT('Ctrl Pts',(19.1295827650218,7.49741935561041,27.5300055539183));
#55204=CARTESIAN_POINT('Ctrl Pts',(18.8261415870883,6.90717528281466,27.8170498721766));
#55205=CARTESIAN_POINT('Ctrl Pts',(18.5104994276256,6.31111450131055,28.0937655905368));
#55206=CARTESIAN_POINT('Ctrl Pts',(18.2016639423759,5.75492178098747,28.3466719251461));
#55207=CARTESIAN_POINT('Ctrl Pts',(17.6747132403632,4.80591767224158,28.778193485753));
#55208=CARTESIAN_POINT('Ctrl Pts',(17.2016343370993,3.9436255315325,29.1307365554341));
#55209=CARTESIAN_POINT('Ctrl Pts',(16.8729352926459,3.36394482370453,29.365352154054));
#55210=CARTESIAN_POINT('Ctrl Pts',(16.6342454025476,2.94300072064618,29.5357218962085));
#55211=CARTESIAN_POINT('Ctrl Pts',(16.5014949770664,2.71490739519207,29.6262286540088));
#55212=CARTESIAN_POINT('Ctrl Pts',(16.3424569562978,2.44504465168102,29.7338311889201));
#55213=CARTESIAN_POINT('Ctrl Pts',(15.993118510103,1.85227173456061,29.9701878926247));
#55214=CARTESIAN_POINT('Ctrl Pts',(15.6312480487537,1.26509075909629,30.2031020416042));
#55215=CARTESIAN_POINT('Ctrl Pts',(15.2503296894305,0.693179555091501,30.4420009717055));
#55216=CARTESIAN_POINT('Ctrl Pts',(14.7484414179076,-0.0603559955513863,
30.7567680816717));
#55217=CARTESIAN_POINT('Ctrl Pts',(14.2669345517206,-0.791651325392304,
31.0498576441856));
#55218=CARTESIAN_POINT('Ctrl Pts',(13.7912435751455,-1.46438575958394,31.3399123313253));
#55219=CARTESIAN_POINT('Ctrl Pts',(13.5533980868579,-1.80075297667976,31.4849396748952));
#55220=CARTESIAN_POINT('Ctrl Pts',(13.3161115657262,-2.1244256180349,31.6299384327499));
#55221=CARTESIAN_POINT('Ctrl Pts',(13.0766514227367,-2.43421540696108,31.7786491461901));
#55222=CARTESIAN_POINT('Ctrl Pts',(12.9188702359555,-2.63833706135937,31.8766351933073));
#55223=CARTESIAN_POINT('Ctrl Pts',(12.7601526360409,-2.83643714593442,31.9762372272926));
#55224=CARTESIAN_POINT('Ctrl Pts',(12.5997389313808,-3.02815130787591,32.0786431431723));
#55225=CARTESIAN_POINT('Ctrl Pts',(12.5166971934814,-3.12739642674706,32.1316558533011));
#55226=CARTESIAN_POINT('Ctrl Pts',(12.4397215765388,-3.21752746773653,32.1811723683389));
#55227=CARTESIAN_POINT('Ctrl Pts',(12.3478597934844,-3.32215188831681,32.2409557398963));
#55228=CARTESIAN_POINT('Ctrl Pts',(11.9116121727781,-3.8190087207047,32.5248643766822));
#55229=CARTESIAN_POINT('Ctrl Pts',(10.7144663992386,-5.25575553834431,33.2889282188856));
#55230=CARTESIAN_POINT('Ctrl Pts',(9.56604185022482,-6.09942127757595,34.2764524708192));
#55231=CARTESIAN_POINT('Ctrl Pts',(9.07284645450781,-6.46173681538865,34.7005486072444));
#55232=CARTESIAN_POINT('Ctrl Pts',(8.57333454992787,-6.74267387425559,35.171504935247));
#55233=CARTESIAN_POINT('Ctrl Pts',(8.00348148263079,-7.02395144844514,35.7754858324545));
#55234=CARTESIAN_POINT('Ctrl Pts',(7.63919428965979,-7.20376239240166,36.1615897569194));
#55235=CARTESIAN_POINT('Ctrl Pts',(7.24388644384695,-7.38116314765918,36.6129669384717));
#55236=CARTESIAN_POINT('Ctrl Pts',(6.94254646282575,-7.51431133904849,36.9770001219077));
#55237=CARTESIAN_POINT('Ctrl Pts',(6.91433564865292,-7.52677639221536,37.0110801416112));
#55238=CARTESIAN_POINT('Ctrl Pts',(6.88669635040566,-7.53896719832808,37.0446474052169));
#55239=CARTESIAN_POINT('Ctrl Pts',(6.85962514029878,-7.55089284691699,37.0776869008724));
#55240=CARTESIAN_POINT('Ctrl Pts',(6.44000062073739,-7.73574954670347,37.5898244239546));
#55241=CARTESIAN_POINT('Ctrl Pts',(6.15412442492902,-7.81952894703128,37.9841916530545));
#55242=CARTESIAN_POINT('Ctrl Pts',(6.,-7.86863926112478,38.1979648172293));
#55243=CARTESIAN_POINT('Ctrl Pts',(2.1,-1.28114692797347,9.65763472891602));
#55244=CARTESIAN_POINT('Ctrl Pts',(2.73333333333333,-1.28114692797347,9.65763472891602));
#55245=CARTESIAN_POINT('Ctrl Pts',(3.36701669548158,-1.28120274047516,9.65763272452521));
#55246=CARTESIAN_POINT('Ctrl Pts',(4.12582575310106,-1.28121960670544,9.65763220679461));
#55247=CARTESIAN_POINT('Ctrl Pts',(4.38278636589858,-1.28250284215921,9.65747570633452));
#55248=CARTESIAN_POINT('Ctrl Pts',(4.88875443651799,-1.28819124993779,9.65678908665978));
#55249=CARTESIAN_POINT('Ctrl Pts',(5.76580325925563,-1.30131080478345,9.65522040881189));
#55250=CARTESIAN_POINT('Ctrl Pts',(6.49302708244736,-1.30111147249391,9.65528059069283));
#55251=CARTESIAN_POINT('Ctrl Pts',(7.02340672589377,-1.27967384267621,9.6577356709489));
#55252=CARTESIAN_POINT('Ctrl Pts',(7.14986679476879,-1.2744035847383,9.65840531711269));
#55253=CARTESIAN_POINT('Ctrl Pts',(7.33705121725519,-1.26602996195062,9.65954820770469));
#55254=CARTESIAN_POINT('Ctrl Pts',(7.52532549516812,-1.25695505359351,9.66085108878951));
#55255=CARTESIAN_POINT('Ctrl Pts',(7.90080343897497,-1.23734054050575,9.66372617426799));
#55256=CARTESIAN_POINT('Ctrl Pts',(8.46124590624133,-1.20179139860997,9.66897349947471));
#55257=CARTESIAN_POINT('Ctrl Pts',(9.0650192250414,-1.14716675316572,9.67573613473312));
#55258=CARTESIAN_POINT('Ctrl Pts',(9.52839384147276,-1.09219084928558,9.68122767953111));
#55259=CARTESIAN_POINT('Ctrl Pts',(9.75198702930936,-1.06064937497063,9.68391236927288));
#55260=CARTESIAN_POINT('Ctrl Pts',(10.3692921392863,-0.965652648141829,
9.69126404805778));
#55261=CARTESIAN_POINT('Ctrl Pts',(11.3477764514917,-0.751349332513189,
9.71242942002159));
#55262=CARTESIAN_POINT('Ctrl Pts',(12.273624621788,-0.471227384196326,9.73058177218512));
#55263=CARTESIAN_POINT('Ctrl Pts',(13.0004910640178,-0.241262883353551,
9.73434036989634));
#55264=CARTESIAN_POINT('Ctrl Pts',(13.5002210053635,-0.0656770837232706,
9.73563225387362));
#55265=CARTESIAN_POINT('Ctrl Pts',(14.4706186721272,0.32956163981752,9.73289534983573));
#55266=CARTESIAN_POINT('Ctrl Pts',(15.1515630987551,0.653141644356525,9.71756271653061));
#55267=CARTESIAN_POINT('Ctrl Pts',(15.8843828864863,1.00441577560146,9.68186404942655));
#55268=CARTESIAN_POINT('Ctrl Pts',(16.3868682969429,1.26265129573327,9.65060020522716));
#55269=CARTESIAN_POINT('Ctrl Pts',(17.3638401545857,1.81703406288438,9.5663953411847));
#55270=CARTESIAN_POINT('Ctrl Pts',(18.0499667751367,2.24816630064726,9.47400212950933));
#55271=CARTESIAN_POINT('Ctrl Pts',(18.7841437937616,2.70564998147611,9.34646266782294));
#55272=CARTESIAN_POINT('Ctrl Pts',(19.2876952035555,3.03517152447214,9.24488767133294));
#55273=CARTESIAN_POINT('Ctrl Pts',(20.2707977577484,3.7219238542422,8.99850535487191));
#55274=CARTESIAN_POINT('Ctrl Pts',(20.9685540112183,4.235972155578,8.76598582891085));
#55275=CARTESIAN_POINT('Ctrl Pts',(22.6570377008399,5.43415064582254,8.1180933488664));
#55276=CARTESIAN_POINT('Ctrl Pts',(23.7241254823866,6.21485531376477,7.52080745806043));
#55277=CARTESIAN_POINT('Ctrl Pts',(24.6950729185821,6.9548534027433,6.78592542456852));
#55278=CARTESIAN_POINT('Ctrl Pts',(2.1,-2.21221115744603,13.7368936516971));
#55279=CARTESIAN_POINT('Ctrl Pts',(2.73333333333333,-2.21221115744603,13.7368936516971));
#55280=CARTESIAN_POINT('Ctrl Pts',(3.36721312611028,-2.212274819488,13.7368878045733));
#55281=CARTESIAN_POINT('Ctrl Pts',(4.12624134471083,-2.21229370557991,13.7368861759272));
#55282=CARTESIAN_POINT('Ctrl Pts',(4.3860549636034,-2.21413081411987,13.7366102290359));
#55283=CARTESIAN_POINT('Ctrl Pts',(4.89391292370119,-2.22224402939692,13.7354015386744));
#55284=CARTESIAN_POINT('Ctrl Pts',(5.77025435885904,-2.24089536952233,13.7326445504079));
#55285=CARTESIAN_POINT('Ctrl Pts',(6.48769850774887,-2.24046786125482,13.7327531026294));
#55286=CARTESIAN_POINT('Ctrl Pts',(7.00643829240506,-2.21043597265355,13.7370420202613));
#55287=CARTESIAN_POINT('Ctrl Pts',(7.13275034169493,-2.20294627186771,13.7382060585672));
#55288=CARTESIAN_POINT('Ctrl Pts',(7.31833052215287,-2.19110496486678,13.7401615208733));
#55289=CARTESIAN_POINT('Ctrl Pts',(7.50526106344739,-2.17826120362336,13.7423748920571));
#55290=CARTESIAN_POINT('Ctrl Pts',(7.87736941114561,-2.15053462971115,13.7472402835191));
#55291=CARTESIAN_POINT('Ctrl Pts',(8.43154979519769,-2.10033857529429,13.7561031931122));
#55292=CARTESIAN_POINT('Ctrl Pts',(9.02547054687868,-2.02346233065752,13.7678309754653));
#55293=CARTESIAN_POINT('Ctrl Pts',(9.47898143432341,-1.94636277550259,13.7777315018726));
#55294=CARTESIAN_POINT('Ctrl Pts',(9.69689934795854,-1.90224417438758,13.7827387521995));
#55295=CARTESIAN_POINT('Ctrl Pts',(10.2969337278913,-1.76957263587484,13.7967587059728));
#55296=CARTESIAN_POINT('Ctrl Pts',(11.2522303770065,-1.4696861906153,13.8352459397839));
#55297=CARTESIAN_POINT('Ctrl Pts',(12.1683201134608,-1.07356159461314,13.8726526533793));
#55298=CARTESIAN_POINT('Ctrl Pts',(12.8911734653119,-0.746687011509429,
13.8874770909768));
#55299=CARTESIAN_POINT('Ctrl Pts',(13.3786074158793,-0.500607932547462,
13.8966643733047));
#55300=CARTESIAN_POINT('Ctrl Pts',(14.3384206267996,0.0584081193865376,
13.9098212945186));
#55301=CARTESIAN_POINT('Ctrl Pts',(15.0146615424652,0.519121115919698,13.9020742478091));
#55302=CARTESIAN_POINT('Ctrl Pts',(15.746048046055,1.02169095472785,13.86617557386));
#55303=CARTESIAN_POINT('Ctrl Pts',(16.242728877042,1.38808517145924,13.8334463689218));
#55304=CARTESIAN_POINT('Ctrl Pts',(17.2171396935533,2.1807240013221,13.7384313437697));
#55305=CARTESIAN_POINT('Ctrl Pts',(17.901644760173,2.79999400820501,13.6257148243664));
#55306=CARTESIAN_POINT('Ctrl Pts',(18.635036129223,3.45866556557441,13.4635963097359));
#55307=CARTESIAN_POINT('Ctrl Pts',(19.138368982942,3.93302752738387,13.3339158646569));
#55308=CARTESIAN_POINT('Ctrl Pts',(20.1238246490668,4.92585190997813,13.0127240131391));
#55309=CARTESIAN_POINT('Ctrl Pts',(20.8219879064555,5.67099230989098,12.7030107212261));
#55310=CARTESIAN_POINT('Ctrl Pts',(22.5097170303094,7.41023638571154,11.829789792395));
#55311=CARTESIAN_POINT('Ctrl Pts',(23.5814142719248,8.55489393715888,11.0112481940202));
#55312=CARTESIAN_POINT('Ctrl Pts',(24.5630597774301,9.65314473468797,9.98522809376511));
#55313=CARTESIAN_POINT('Ctrl Pts',(2.1,-4.38469435954868,23.2551644715195));
#55314=CARTESIAN_POINT('Ctrl Pts',(2.73333333333333,-4.38469435954868,23.2551644715195));
#55315=CARTESIAN_POINT('Ctrl Pts',(3.36769471511647,-4.38488057129456,23.2551532064746));
#55316=CARTESIAN_POINT('Ctrl Pts',(4.1272406751542,-4.38493601711281,23.2551502171888));
#55317=CARTESIAN_POINT('Ctrl Pts',(4.39371542805278,-4.38811237897684,23.2545870692032));
#55318=CARTESIAN_POINT('Ctrl Pts',(4.90597407671282,-4.40197836606138,23.2521437544136));
#55319=CARTESIAN_POINT('Ctrl Pts',(5.7807080208241,-4.43354775064731,23.2466189723673));
#55320=CARTESIAN_POINT('Ctrl Pts',(6.47526981917573,-4.43237909948388,23.2469264289471));
#55321=CARTESIAN_POINT('Ctrl Pts',(6.96712055433637,-4.38373884372307,23.2551815947408));
#55322=CARTESIAN_POINT('Ctrl Pts',(7.09309241227956,-4.37109334355141,23.2574951210814));
#55323=CARTESIAN_POINT('Ctrl Pts',(7.27497337036715,-4.351375704304,23.2613005282899));
#55324=CARTESIAN_POINT('Ctrl Pts',(7.45881576444989,-4.32994273678029,23.2655958831574));
#55325=CARTESIAN_POINT('Ctrl Pts',(7.82318936765134,-4.28381461113148,23.274992130574));
#55326=CARTESIAN_POINT('Ctrl Pts',(8.36312569624925,-4.20072544276082,23.2920454909141));
#55327=CARTESIAN_POINT('Ctrl Pts',(8.93510635605503,-4.07458377982203,23.3148346780207));
#55328=CARTESIAN_POINT('Ctrl Pts',(9.36759672724957,-3.94929372225073,23.3343645701841));
#55329=CARTESIAN_POINT('Ctrl Pts',(9.57394607457417,-3.87811577159792,23.3443682182037));
#55330=CARTESIAN_POINT('Ctrl Pts',(10.1400380810636,-3.66525566654609,23.3725990353288));
#55331=CARTESIAN_POINT('Ctrl Pts',(11.0614325554581,-3.17865730581794,23.4497905636272));
#55332=CARTESIAN_POINT('Ctrl Pts',(11.9722693017586,-2.51485712541299,23.532986674016));
#55333=CARTESIAN_POINT('Ctrl Pts',(12.6924963782862,-1.96359415406124,23.5743666485978));
#55334=CARTESIAN_POINT('Ctrl Pts',(13.175889377178,-1.55399509894084,23.6027261013292));
#55335=CARTESIAN_POINT('Ctrl Pts',(14.1420689046042,-0.604663058554355,
23.6550841747934));
#55336=CARTESIAN_POINT('Ctrl Pts',(14.8238605574682,0.181234839702475,23.6661844031786));
#55337=CARTESIAN_POINT('Ctrl Pts',(15.5572436616688,1.03764444286935,23.6307306769521));
#55338=CARTESIAN_POINT('Ctrl Pts',(16.0655714023431,1.67005225479606,23.594824522056));
#55339=CARTESIAN_POINT('Ctrl Pts',(17.0554148112706,3.03886141709287,23.4727037999293));
#55340=CARTESIAN_POINT('Ctrl Pts',(17.7492194074361,4.10701720329462,23.31031570719));
#55341=CARTESIAN_POINT('Ctrl Pts',(18.4856236416724,5.23721796897442,23.0659994842294));
#55342=CARTESIAN_POINT('Ctrl Pts',(19.0039934118869,6.06901762023052,22.8653268989984));
#55343=CARTESIAN_POINT('Ctrl Pts',(20.0037041464425,7.79468578904712,22.3590924212079));
#55344=CARTESIAN_POINT('Ctrl Pts',(20.70921584779,9.08661075029831,21.861654374002));
#55345=CARTESIAN_POINT('Ctrl Pts',(22.4031172629537,12.0907653827351,20.4503412208277));
#55346=CARTESIAN_POINT('Ctrl Pts',(23.5045174575955,14.1205525667797,19.0832753645027));
#55347=CARTESIAN_POINT('Ctrl Pts',(24.5018789378046,16.0600964495426,17.350084418661));
#55348=CARTESIAN_POINT('Ctrl Pts',(2.1,-6.55717756165133,32.7734352913419));
#55349=CARTESIAN_POINT('Ctrl Pts',(2.73333333333333,-6.55717756165133,32.7734352913419));
#55350=CARTESIAN_POINT('Ctrl Pts',(3.36823422033876,-6.55733365835752,32.7734302460344));
#55351=CARTESIAN_POINT('Ctrl Pts',(4.12831140060925,-6.55737729440761,32.7734296688118));
#55352=CARTESIAN_POINT('Ctrl Pts',(4.40146367837934,-6.56196909742548,32.7725602253241));
#55353=CARTESIAN_POINT('Ctrl Pts',(4.91806272527724,-6.58173623082086,32.76884327078));
#55354=CARTESIAN_POINT('Ctrl Pts',(5.79139783182175,-6.62612337659199,32.7605686737685));
#55355=CARTESIAN_POINT('Ctrl Pts',(6.46265872030445,-6.62323378721398,32.761262568013));
#55356=CARTESIAN_POINT('Ctrl Pts',(6.9289941766225,-6.55893905781572,32.772802106805));
#55357=CARTESIAN_POINT('Ctrl Pts',(7.05465117146563,-6.54117940276051,32.7762565405843));
#55358=CARTESIAN_POINT('Ctrl Pts',(7.23305738134067,-6.51402594214224,32.7818127633436));
#55359=CARTESIAN_POINT('Ctrl Pts',(7.41404715164792,-6.48440358817651,32.7881007548297));
#55360=CARTESIAN_POINT('Ctrl Pts',(7.77133867510313,-6.4209500807349,32.8017918588461));
#55361=CARTESIAN_POINT('Ctrl Pts',(8.29877981539897,-6.30710599255026,32.8265515875734));
#55362=CARTESIAN_POINT('Ctrl Pts',(8.85378665049961,-6.13594718228628,32.8595134623599));
#55363=CARTESIAN_POINT('Ctrl Pts',(9.2734143759592,-5.96649254262646,32.8879015674141));
#55364=CARTESIAN_POINT('Ctrl Pts',(9.47424581976662,-5.87008555018478,32.9025811140304));
#55365=CARTESIAN_POINT('Ctrl Pts',(10.0273490535427,-5.58086225664978,32.9443886029256));
#55366=CARTESIAN_POINT('Ctrl Pts',(10.95724978738,-4.89624833181571,33.0629975685759));
#55367=CARTESIAN_POINT('Ctrl Pts',(11.8781516205332,-3.94888311770831,33.1941309591058));
#55368=CARTESIAN_POINT('Ctrl Pts',(12.602064400414,-3.16718879965623,33.2625544037443));
#55369=CARTESIAN_POINT('Ctrl Pts',(13.0988694696214,-2.57261376786209,33.3120220678116));
#55370=CARTESIAN_POINT('Ctrl Pts',(14.0796924707411,-1.2066313810241,33.4035962308661));
#55371=CARTESIAN_POINT('Ctrl Pts',(14.7676661666682,-0.0828568772261278,
33.4312577852876));
#55372=CARTESIAN_POINT('Ctrl Pts',(15.5027143066566,1.13114584822823,33.3935159926964));
#55373=CARTESIAN_POINT('Ctrl Pts',(16.0202838183814,2.0480009213489,33.3515195947089));
#55374=CARTESIAN_POINT('Ctrl Pts',(17.0170397773181,4.00663252246451,33.1950226426635));
#55375=CARTESIAN_POINT('Ctrl Pts',(17.7141529625547,5.52939972439683,32.9767008794832));
#55376=CARTESIAN_POINT('Ctrl Pts',(18.4513779804965,7.13168519855837,32.6442892324621));
#55377=CARTESIAN_POINT('Ctrl Pts',(18.9741471075058,8.32767525987012,32.3665292176382));
#55378=CARTESIAN_POINT('Ctrl Pts',(19.976694090316,10.7868079909045,31.6647961243488));
#55379=CARTESIAN_POINT('Ctrl Pts',(20.6835910141171,12.6238140087707,30.9721601751623));
#55380=CARTESIAN_POINT('Ctrl Pts',(22.3784981023364,16.8857640647611,29.0059479969508));
#55381=CARTESIAN_POINT('Ctrl Pts',(23.4839952293235,19.7901269247353,27.0797142961554));
#55382=CARTESIAN_POINT('Ctrl Pts',(24.4831092917558,22.5567994415466,24.6338907495562));
#55383=CARTESIAN_POINT('Ctrl Pts',(2.1,-7.79859653428142,38.2124471883833));
#55384=CARTESIAN_POINT('Ctrl Pts',(2.73333333333333,-7.79859653428142,38.2124471883833));
#55385=CARTESIAN_POINT('Ctrl Pts',(3.36856062451574,-7.79873444591204,38.2124447399906));
#55386=CARTESIAN_POINT('Ctrl Pts',(4.12894455864879,-7.79877122896585,38.2124451854717));
#55387=CARTESIAN_POINT('Ctrl Pts',(4.40592023303614,-7.8041991375916,38.2113944348269));
#55388=CARTESIAN_POINT('Ctrl Pts',(4.92496378260879,-7.82740050255151,38.206935096053));
#55389=CARTESIAN_POINT('Ctrl Pts',(5.79760871146345,-7.87907393959177,38.1970978805761));
#55390=CARTESIAN_POINT('Ctrl Pts',(6.45531298767032,-7.87500898787854,38.1980539230733));
#55391=CARTESIAN_POINT('Ctrl Pts',(6.9077976809273,-7.80261420329609,38.2112781567269));
#55392=CARTESIAN_POINT('Ctrl Pts',(7.0332878180794,-7.78194383532455,38.215382261872));
#55393=CARTESIAN_POINT('Ctrl Pts',(7.20982673716659,-7.75066227156594,38.2219121181203));
#55394=CARTESIAN_POINT('Ctrl Pts',(7.389307620971,-7.7164659210836,38.2293156575816));
#55395=CARTESIAN_POINT('Ctrl Pts',(7.74288824317936,-7.64337852998469,38.245403215072));
#55396=CARTESIAN_POINT('Ctrl Pts',(8.26404052600409,-7.51246641850933,38.274457453936));
#55397=CARTESIAN_POINT('Ctrl Pts',(8.81154663884202,-7.31609326494859,38.3131349275136));
#55398=CARTESIAN_POINT('Ctrl Pts',(9.22663616903524,-7.12105996837216,38.3466696593823));
#55399=CARTESIAN_POINT('Ctrl Pts',(9.42600345931065,-7.00962245615174,38.3641521150841));
#55400=CARTESIAN_POINT('Ctrl Pts',(9.97673035450293,-6.67410993020777,38.4142586338593));
#55401=CARTESIAN_POINT('Ctrl Pts',(10.9140328205435,-5.86861558602685,38.5578683438277));
#55402=CARTESIAN_POINT('Ctrl Pts',(11.8387370187856,-4.75720739105203,38.7162552762356));
#55403=CARTESIAN_POINT('Ctrl Pts',(12.5644578213362,-3.84288974266347,38.7999538670138));
#55404=CARTESIAN_POINT('Ctrl Pts',(13.066322703487,-3.14070085828515,38.8614056110336));
#55405=CARTESIAN_POINT('Ctrl Pts',(14.0520220952575,-1.53711560165909,38.9747074705805));
#55406=CARTESIAN_POINT('Ctrl Pts',(14.7426079813353,-0.220446917943601,
39.0113449605053));
#55407=CARTESIAN_POINT('Ctrl Pts',(15.4784644022037,1.19801237275349,38.9717886737579));
#55408=CARTESIAN_POINT('Ctrl Pts',(15.9995803483975,2.27611610107773,38.925960287591));
#55409=CARTESIAN_POINT('Ctrl Pts',(16.9994385686868,4.56988282057309,38.7493359633624));
#55410=CARTESIAN_POINT('Ctrl Pts',(17.6981355886256,6.35201308463761,38.4986340630539));
#55411=CARTESIAN_POINT('Ctrl Pts',(18.4357025434826,8.22406759263825,38.1153991106372));
#55412=CARTESIAN_POINT('Ctrl Pts',(18.9608213396521,9.62691357240197,37.7935110674948));
#55413=CARTESIAN_POINT('Ctrl Pts',(19.9653436397241,12.5041437675931,36.97985111824));
#55414=CARTESIAN_POINT('Ctrl Pts',(20.6729453639354,14.6522661765941,36.1753281013235));
#55415=CARTESIAN_POINT('Ctrl Pts',(22.3680401919045,19.6325296413544,33.8910883575064));
#55416=CARTESIAN_POINT('Ctrl Pts',(23.4757593035169,23.0350551290633,31.6450395565025));
#55417=CARTESIAN_POINT('Ctrl Pts',(24.4767076204831,26.2741907223813,28.7915599578483));
#55418=CARTESIAN_POINT('',(3.2,-7.48695481785667,36.8470556158206));
#55419=CARTESIAN_POINT('Ctrl Pts',(3.2,-7.48695481785667,36.8470556158206));
#55420=CARTESIAN_POINT('Ctrl Pts',(3.45174020136192,-7.31395079566958,36.089075469184));
#55421=CARTESIAN_POINT('Ctrl Pts',(3.71840125365622,-7.13890531377323,35.3221511031575));
#55422=CARTESIAN_POINT('Ctrl Pts',(4.,-6.96288805731186,34.5509691145741));
#55423=CARTESIAN_POINT('Ctrl Pts',(4.62816480834395,-6.57024481011749,32.8306866476012));
#55424=CARTESIAN_POINT('Ctrl Pts',(5.32582966279889,-6.23689128633005,31.0992624735586));
#55425=CARTESIAN_POINT('Ctrl Pts',(6.03866106850362,-5.87030121037977,29.5163236792264));
#55426=CARTESIAN_POINT('Ctrl Pts',(6.32798217235993,-5.72151112539207,28.8738469369729));
#55427=CARTESIAN_POINT('Ctrl Pts',(6.61604116347502,-5.5677970636221,28.26345485931));
#55428=CARTESIAN_POINT('Ctrl Pts',(6.89476148100328,-5.40504398120696,27.6978623915459));
#55429=CARTESIAN_POINT('Ctrl Pts',(7.65522893079838,-4.96098442132935,26.1546858287526));
#55430=CARTESIAN_POINT('Ctrl Pts',(8.35226709607949,-4.55968381483506,24.9175441087371));
#55431=CARTESIAN_POINT('Ctrl Pts',(8.78926323826716,-4.29164296772241,24.1737483921843));
#55432=CARTESIAN_POINT('Ctrl Pts',(8.99031957410375,-4.16832080221034,23.8315374961511));
#55433=CARTESIAN_POINT('Ctrl Pts',(9.18275521560808,-4.04719763389059,23.5131938148023));
#55434=CARTESIAN_POINT('Ctrl Pts',(9.37496045132061,-3.92148904458358,23.203169428056));
#55435=CARTESIAN_POINT('Ctrl Pts',(9.48075232667821,-3.8522976546506,23.0325285963487));
#55436=CARTESIAN_POINT('Ctrl Pts',(9.58626090583131,-3.78183212273648,22.8648155089132));
#55437=CARTESIAN_POINT('Ctrl Pts',(9.69257910363365,-3.70887202431335,22.6982720777597));
#55438=CARTESIAN_POINT('Ctrl Pts',(10.0319880462582,-3.47595507903542,22.1666008207471));
#55439=CARTESIAN_POINT('Ctrl Pts',(10.3788056733388,-3.21653295379331,21.6469362728903));
#55440=CARTESIAN_POINT('Ctrl Pts',(10.7756849077178,-2.90649416731403,21.0798294966464));
#55441=CARTESIAN_POINT('Ctrl Pts',(10.8890930398495,-2.81790066929938,20.917778891218));
#55442=CARTESIAN_POINT('Ctrl Pts',(11.0576203517596,-2.68502865207462,20.6789427589835));
#55443=CARTESIAN_POINT('Ctrl Pts',(11.2725125491579,-2.51363785689445,20.3827664323304));
#55444=CARTESIAN_POINT('Ctrl Pts',(11.5968279592171,-2.25497478446942,19.9357769744012));
#55445=CARTESIAN_POINT('Ctrl Pts',(12.0255678842989,-1.90626438158956,19.3605597033925));
#55446=CARTESIAN_POINT('Ctrl Pts',(12.532035905153,-1.51672858576023,18.715758252655));
#55447=CARTESIAN_POINT('Ctrl Pts',(13.0988763178897,-1.08075904337671,17.9940946817688));
#55448=CARTESIAN_POINT('Ctrl Pts',(13.7495416923942,-0.541391711628421,
17.2086401181151));
#55449=CARTESIAN_POINT('Ctrl Pts',(14.4398764947203,0.0176411498964413,
16.421589811873));
#55450=CARTESIAN_POINT('Ctrl Pts',(14.7901814044069,0.301317933115872,16.0222073882751));
#55451=CARTESIAN_POINT('Ctrl Pts',(15.1459546156529,0.582681643644018,15.6283594122733));
#55452=CARTESIAN_POINT('Ctrl Pts',(15.4570717747561,0.815857706666163,15.2925887900305));
#55453=CARTESIAN_POINT('Ctrl Pts',(15.7998231395665,1.0727429716009,14.922677212769));
#55454=CARTESIAN_POINT('Ctrl Pts',(16.0676294472855,1.27727353930151,14.6416351637504));
#55455=CARTESIAN_POINT('Ctrl Pts',(16.3615307941354,1.50139670385469,14.3383117695221));
#55456=CARTESIAN_POINT('Ctrl Pts',(17.0296616001641,2.01089961082543,13.6487616669271));
#55457=CARTESIAN_POINT('Ctrl Pts',(17.7084691863034,2.53245724211085,12.9775795790632));
#55458=CARTESIAN_POINT('Ctrl Pts',(18.4207032016838,3.01739152515405,12.3152017758896));
#55459=CARTESIAN_POINT('Ctrl Pts',(18.8298642041348,3.29597439691827,11.9346819465985));
#55460=CARTESIAN_POINT('Ctrl Pts',(19.2113759271843,3.56048865862558,11.5875850942181));
#55461=CARTESIAN_POINT('Ctrl Pts',(19.5701113606338,3.80689943954097,11.2647488766695));
#55462=CARTESIAN_POINT('Ctrl Pts',(20.1215476021662,4.18567394083428,10.768495722294));
#55463=CARTESIAN_POINT('Ctrl Pts',(20.6514912602097,4.55442248629506,10.2954021170133));
#55464=CARTESIAN_POINT('Ctrl Pts',(21.3979544325339,5.00660433247608,9.65730708454375));
#55465=CARTESIAN_POINT('Ctrl Pts',(21.8107631282391,5.25666971421805,9.30442808413761));
#55466=CARTESIAN_POINT('Ctrl Pts',(22.3076315955878,5.54996514997988,8.88383089702849));
#55467=CARTESIAN_POINT('Ctrl Pts',(22.8472772295773,5.86208436754307,8.41699874974435));
#55468=CARTESIAN_POINT('Ctrl Pts',(23.3953136569067,6.17905663623287,7.94290796489216));
#55469=CARTESIAN_POINT('Ctrl Pts',(23.9608264583334,6.50100102939092,7.44199090360229));
#55470=CARTESIAN_POINT('Ctrl Pts',(24.5,6.80662575089405,6.93067919103514));
#55471=CARTESIAN_POINT('Ctrl Pts',(2.7976125197915,-7.69632218254969,37.764160171016));
#55472=CARTESIAN_POINT('Ctrl Pts',(2.93206640474696,-7.62662479454036,37.4587302040282));
#55473=CARTESIAN_POINT('Ctrl Pts',(3.06672620115017,-7.55684524328147,37.1529290248933));
#55474=CARTESIAN_POINT('Ctrl Pts',(3.20143890385924,-7.48704899610989,36.8470537203075));
#55475=CARTESIAN_POINT('Origin',(2.9,0.,0.));
#55476=CARTESIAN_POINT('Origin',(3.2,0.,0.));
#55477=CARTESIAN_POINT('Ctrl Pts',(2.09999999999999,5.34569526878069,8.14677776873086));
#55478=CARTESIAN_POINT('Ctrl Pts',(2.73333333333333,5.34569526878069,8.14677776873086));
#55479=CARTESIAN_POINT('Ctrl Pts',(3.36630034669941,5.34572932827768,8.14673820499258));
#55480=CARTESIAN_POINT('Ctrl Pts',(4.12415222295647,5.34573957275389,8.1467261713621));
#55481=CARTESIAN_POINT('Ctrl Pts',(4.36790021147292,5.34472553942211,8.14740587797417));
#55482=CARTESIAN_POINT('Ctrl Pts',(4.86512966195106,5.34009529004106,8.15052042278991));
#55483=CARTESIAN_POINT('Ctrl Pts',(5.74554670028596,5.32916987892461,8.15788640243843));
#55484=CARTESIAN_POINT('Ctrl Pts',(6.51831318247728,5.32899607663781,8.15800776496995));
#55485=CARTESIAN_POINT('Ctrl Pts',(7.10304257246599,5.34865471993144,8.1446302741035));
#55486=CARTESIAN_POINT('Ctrl Pts',(7.23019774633306,5.35310568763719,8.14167315323862));
#55487=CARTESIAN_POINT('Ctrl Pts',(7.42487767291169,5.36047814040294,8.13686977999796));
#55488=CARTESIAN_POINT('Ctrl Pts',(7.61944738538559,5.36848260168234,8.13172941156603));
#55489=CARTESIAN_POINT('Ctrl Pts',(8.01069407403727,5.38595279816171,8.120578662717));
#55490=CARTESIAN_POINT('Ctrl Pts',(8.60076076555801,5.41803622104533,8.10009941893901));
#55491=CARTESIAN_POINT('Ctrl Pts',(9.2514693452681,5.46730206741326,8.06707288500877));
#55492=CARTESIAN_POINT('Ctrl Pts',(9.76259388701861,5.51702797098133,8.03209010716476));
#55493=CARTESIAN_POINT('Ctrl Pts',(10.0140925250858,5.54573721585672,8.01129437931371));
#55494=CARTESIAN_POINT('Ctrl Pts',(10.7176766675203,5.63295501491629,7.94712173936429));
#55495=CARTESIAN_POINT('Ctrl Pts',(11.8207864606551,5.83200083591163,7.80546186007917));
#55496=CARTESIAN_POINT('Ctrl Pts',(12.8079685189794,6.07032563529004,7.62162237801202));
#55497=CARTESIAN_POINT('Ctrl Pts',(13.5603848523328,6.25130155066986,7.46780194988823));
#55498=CARTESIAN_POINT('Ctrl Pts',(14.1415274513423,6.40507133769525,7.3346969582253));
#55499=CARTESIAN_POINT('Ctrl Pts',(15.2007173823881,6.72668652876932,7.04487589906985));
#55500=CARTESIAN_POINT('Ctrl Pts',(15.9285144230346,6.97318784291672,6.80160018473738));
#55501=CARTESIAN_POINT('Ctrl Pts',(16.6747983655381,7.21490870896561,6.53624796834907));
#55502=CARTESIAN_POINT('Ctrl Pts',(17.2498259297328,7.41028452077371,6.31310610738743));
#55503=CARTESIAN_POINT('Ctrl Pts',(18.298502385672,7.7908485469562,5.84489796690035));
#55504=CARTESIAN_POINT('Ctrl Pts',(19.0237218101043,8.06049256566364,5.46513485251275));
#55505=CARTESIAN_POINT('Ctrl Pts',(19.7682624700467,8.31477089119449,5.0568703055287));
#55506=CARTESIAN_POINT('Ctrl Pts',(20.3332247834019,8.50943535027493,4.72383204545389));
#55507=CARTESIAN_POINT('Ctrl Pts',(21.3723657664017,8.86395000435395,4.03736317745124));
#55508=CARTESIAN_POINT('Ctrl Pts',(22.0962933246612,9.08773286473061,3.49670452915844));
#55509=CARTESIAN_POINT('Ctrl Pts',(23.230285826829,9.37695244520676,2.62988617519763));
#55510=CARTESIAN_POINT('Ctrl Pts',(23.8854423668127,9.50857067043872,2.08256115897413));
#55511=CARTESIAN_POINT('Ctrl Pts',(24.5000000001022,9.59462155805315,1.51911333273275));
#55512=CARTESIAN_POINT('Ctrl Pts',(2.09999999999999,7.95431935050272,11.4178889030821));
#55513=CARTESIAN_POINT('Ctrl Pts',(2.73333333333333,7.95431935050272,11.4178889030821));
#55514=CARTESIAN_POINT('Ctrl Pts',(3.36609905747045,7.95436068480874,11.4178460511122));
#55515=CARTESIAN_POINT('Ctrl Pts',(4.12372996076631,7.95437287171506,11.4178332681552));
#55516=CARTESIAN_POINT('Ctrl Pts',(4.36462463573312,7.95296242822486,11.4188381049305));
#55517=CARTESIAN_POINT('Ctrl Pts',(4.8599634841508,7.94649420404603,11.4234589089508));
#55518=CARTESIAN_POINT('Ctrl Pts',(5.7410868750954,7.93117831228565,11.4344193928147));
#55519=CARTESIAN_POINT('Ctrl Pts',(6.5236282796852,7.93082369663374,11.4346895818339));
#55520=CARTESIAN_POINT('Ctrl Pts',(7.11999518656519,7.95876090338528,11.4145500209094));
#55521=CARTESIAN_POINT('Ctrl Pts',(7.24729832679298,7.96500410071765,11.4101475403836));
#55522=CARTESIAN_POINT('Ctrl Pts',(7.44358223949712,7.97539578806132,11.4029609179064));
#55523=CARTESIAN_POINT('Ctrl Pts',(7.63949549354406,7.98667025085612,11.3952729249967));
#55524=CARTESIAN_POINT('Ctrl Pts',(8.03411141548379,8.01130481419146,11.3785737699017));
#55525=CARTESIAN_POINT('Ctrl Pts',(8.63043907126314,8.0565947486948,11.3478833478014));
#55526=CARTESIAN_POINT('Ctrl Pts',(9.29099904315616,8.12632114559454,11.2983139694396));
#55527=CARTESIAN_POINT('Ctrl Pts',(9.81198649015675,8.19688630646801,11.2457313990878));
#55528=CARTESIAN_POINT('Ctrl Pts',(10.0691598295132,8.23770627585821,11.2144385788119));
#55529=CARTESIAN_POINT('Ctrl Pts',(10.7900135369803,8.36185925360191,11.1178323753134));
#55530=CARTESIAN_POINT('Ctrl Pts',(11.9163064264562,8.64460860281135,10.9046196798766));
#55531=CARTESIAN_POINT('Ctrl Pts',(12.9132493179395,8.97978135610216,10.630613017264));
#55532=CARTESIAN_POINT('Ctrl Pts',(13.6696831671135,9.23283835425736,10.4027912554835));
#55533=CARTESIAN_POINT('Ctrl Pts',(14.2631240428071,9.45044991189978,10.2036164976331));
#55534=CARTESIAN_POINT('Ctrl Pts',(15.3328942858921,9.90158336336293,9.77293765230881));
#55535=CARTESIAN_POINT('Ctrl Pts',(16.0654073723091,10.2448029848828,9.41400445161443));
#55536=CARTESIAN_POINT('Ctrl Pts',(16.8131365772258,10.57901850791,9.02458364992901));
#55537=CARTESIAN_POINT('Ctrl Pts',(17.3939813143476,10.851263252928,8.69520722532973));
#55538=CARTESIAN_POINT('Ctrl Pts',(18.4452193504662,11.3765346858633,8.00852150865001));
#55539=CARTESIAN_POINT('Ctrl Pts',(19.1721170343286,11.7458521349479,7.45453132983995));
#55540=CARTESIAN_POINT('Ctrl Pts',(19.9174877328955,12.091418353064,6.86049809607568));
#55541=CARTESIAN_POINT('Ctrl Pts',(20.4827387246483,12.356087585852,6.37617988890529));
#55542=CARTESIAN_POINT('Ctrl Pts',(21.5195226714883,12.8327353582581,5.38177661181528));
#55543=CARTESIAN_POINT('Ctrl Pts',(22.2433987526262,13.1292643057035,4.60093146432436));
#55544=CARTESIAN_POINT('Ctrl Pts',(23.3781286077009,13.5049778910929,3.35041159552442));
#55545=CARTESIAN_POINT('Ctrl Pts',(24.0312127056184,13.6700047304202,2.56491139960509));
#55546=CARTESIAN_POINT('Ctrl Pts',(24.6419825553303,13.7690448953621,1.75959950001178));
#55547=CARTESIAN_POINT('Ctrl Pts',(2.09999999999999,14.0411088745208,19.0504815499016));
#55548=CARTESIAN_POINT('Ctrl Pts',(2.73333333333332,14.0411088745208,19.0504815499016));
#55549=CARTESIAN_POINT('Ctrl Pts',(3.36561005673443,14.0412263191859,19.0503511340209));
#55550=CARTESIAN_POINT('Ctrl Pts',(4.12272018987638,14.0412610463446,19.0503120245693));
#55551=CARTESIAN_POINT('Ctrl Pts',(4.35695331957966,14.0389612776608,19.0520444329267));
#55552=CARTESIAN_POINT('Ctrl Pts',(4.84789055187918,14.0282760040565,19.0601164814598));
#55553=CARTESIAN_POINT('Ctrl Pts',(5.73061998203781,14.0027176670903,19.0794536983509));
#55554=CARTESIAN_POINT('Ctrl Pts',(6.53603781131808,14.0017409829267,19.0801839394591));
#55555=CARTESIAN_POINT('Ctrl Pts',(7.15929021859793,14.0501390439893,19.0433328078394));
#55556=CARTESIAN_POINT('Ctrl Pts',(7.28693348498685,14.0605815697539,19.0355424902978));
#55557=CARTESIAN_POINT('Ctrl Pts',(7.48691623290952,14.078188038547,19.0226557527357));
#55558=CARTESIAN_POINT('Ctrl Pts',(7.68591744492013,14.0972533274485,19.0088897738562));
#55559=CARTESIAN_POINT('Ctrl Pts',(8.08826748913676,14.1390214221172,18.9789033544198));
#55560=CARTESIAN_POINT('Ctrl Pts',(8.69883992347527,14.2161182599971,18.923537563707));
#55561=CARTESIAN_POINT('Ctrl Pts',(9.38134013805784,14.3356504197161,18.8336195827372));
#55562=CARTESIAN_POINT('Ctrl Pts',(9.9233475627503,14.4574943433302,18.7376985909731));
#55563=CARTESIAN_POINT('Ctrl Pts',(10.1920889325272,14.5283291258725,18.680388177824));
#55564=CARTESIAN_POINT('Ctrl Pts',(10.9468888975129,14.7445321558586,18.5029076794783));
#55565=CARTESIAN_POINT('Ctrl Pts',(12.1070929839769,15.2320217055213,18.1136587205138));
#55566=CARTESIAN_POINT('Ctrl Pts',(13.1092959939513,15.7943764572631,17.6263674112012));
#55567=CARTESIAN_POINT('Ctrl Pts',(13.8683665989331,16.2161387424221,17.2240481534117));
#55568=CARTESIAN_POINT('Ctrl Pts',(14.465851216866,16.5827359029316,16.869477355448));
#55569=CARTESIAN_POINT('Ctrl Pts',(15.5292553024092,17.3293369894269,16.1151915443042));
#55570=CARTESIAN_POINT('Ctrl Pts',(16.2562016623198,17.8940957313968,15.4897104678438));
#55571=CARTESIAN_POINT('Ctrl Pts',(17.0019161442256,18.4429114016061,14.8108419597527));
#55572=CARTESIAN_POINT('Ctrl Pts',(17.5710904839668,18.8858158377931,14.2440758142749));
#55573=CARTESIAN_POINT('Ctrl Pts',(18.6068900718781,19.7375953416174,13.0645912504827));
#55574=CARTESIAN_POINT('Ctrl Pts',(19.324409219312,20.3350114167168,12.1131549555414));
#55575=CARTESIAN_POINT('Ctrl Pts',(20.0667073169345,20.8934110750517,11.088202506253));
#55576=CARTESIAN_POINT('Ctrl Pts',(20.6168193612055,21.3134200285188,10.2694650930084));
#55577=CARTESIAN_POINT('Ctrl Pts',(21.6393963370735,22.0716356556127,8.57762941163691));
#55578=CARTESIAN_POINT('Ctrl Pts',(22.3554514423905,22.5386470334874,7.24689507937901));
#55579=CARTESIAN_POINT('Ctrl Pts',(23.4866625010404,23.1218327822785,5.10639065291024));
#55580=CARTESIAN_POINT('Ctrl Pts',(24.1251846279709,23.3645442655133,3.78635366314737));
#55581=CARTESIAN_POINT('Ctrl Pts',(24.7276044279209,23.4996227468203,2.42994111486043));
#55582=CARTESIAN_POINT('Ctrl Pts',(2.09999999999999,20.1278983985389,26.6830741967211));
#55583=CARTESIAN_POINT('Ctrl Pts',(2.73333333333333,20.1278983985389,26.6830741967211));
#55584=CARTESIAN_POINT('Ctrl Pts',(3.3650650513931,20.1279907180548,26.6829648227731));
#55585=CARTESIAN_POINT('Ctrl Pts',(4.12164146402536,20.1280157003356,26.6829338985605));
#55586=CARTESIAN_POINT('Ctrl Pts',(4.34919679890247,20.1248892574282,26.6853459614754));
#55587=CARTESIAN_POINT('Ctrl Pts',(4.83579295504009,20.1101102777032,26.696777172012));
#55588=CARTESIAN_POINT('Ctrl Pts',(5.71992017424441,20.0742335862458,26.7245575404596));
#55589=CARTESIAN_POINT('Ctrl Pts',(6.54863427370623,20.0718789324825,26.7263949062999));
#55590=CARTESIAN_POINT('Ctrl Pts',(7.19739899140384,20.1431128638101,26.6709474908365));
#55591=CARTESIAN_POINT('Ctrl Pts',(7.32535704253212,20.1577873874664,26.6597421276243));
#55592=CARTESIAN_POINT('Ctrl Pts',(7.52881418015135,20.182960786228,26.6408726601145));
#55593=CARTESIAN_POINT('Ctrl Pts',(7.73066774801736,20.2101360022771,26.6207718311195));
#55594=CARTESIAN_POINT('Ctrl Pts',(8.14009928573882,20.2698930414322,26.5768039510723));
#55595=CARTESIAN_POINT('Ctrl Pts',(8.76316584740861,20.3805079701614,26.4953932538648));
#55596=CARTESIAN_POINT('Ctrl Pts',(9.46263854560405,20.5531886673258,26.3623600509603));
#55597=CARTESIAN_POINT('Ctrl Pts',(10.017507545926,20.7294232739755,26.2204349152997));
#55598=CARTESIAN_POINT('Ctrl Pts',(10.2917662953052,20.8316640419599,26.1358762893613));
#55599=CARTESIAN_POINT('Ctrl Pts',(11.0595542080066,21.1427939329773,25.8749304546139));
#55600=CARTESIAN_POINT('Ctrl Pts',(12.2112543073819,21.8258513926037,25.3167945268977));
#55601=CARTESIAN_POINT('Ctrl Pts',(13.2033940527264,22.6037886818375,24.6273187356927));
#55602=CARTESIAN_POINT('Ctrl Pts',(13.9587789479009,23.1900942266241,24.054937732768));
#55603=CARTESIAN_POINT('Ctrl Pts',(14.5428532084221,23.690775770569,23.5605522478501));
#55604=CARTESIAN_POINT('Ctrl Pts',(15.5916178900821,24.7164130754297,22.5032405024335));
#55605=CARTESIAN_POINT('Ctrl Pts',(16.3123893656982,25.4965693245089,21.6225906204811));
#55606=CARTESIAN_POINT('Ctrl Pts',(17.0564424910833,26.2597700017511,20.6589372504844));
#55607=CARTESIAN_POINT('Ctrl Pts',(17.616379707499,26.8641130888823,19.8710282227327));
#55608=CARTESIAN_POINT('Ctrl Pts',(18.6452710323621,28.039573237267,18.2139535665106));
#55609=CARTESIAN_POINT('Ctrl Pts',(19.3594959561944,28.8664279612339,16.8734755791401));
#55610=CARTESIAN_POINT('Ctrl Pts',(20.1009829497248,29.6419385160434,15.4217292188935));
#55611=CARTESIAN_POINT('Ctrl Pts',(20.6466969351181,30.2178627789357,14.2776672115503));
#55612=CARTESIAN_POINT('Ctrl Pts',(21.6664536129056,31.2654377485049,11.8953905111638));
#55613=CARTESIAN_POINT('Ctrl Pts',(22.3810862465992,31.9099310212778,10.0181473413673));
#55614=CARTESIAN_POINT('Ctrl Pts',(23.5117833300425,32.7123864767864,6.99078754096831));
#55615=CARTESIAN_POINT('Ctrl Pts',(24.1480627906507,33.0401645369321,5.13769400067936));
#55616=CARTESIAN_POINT('Ctrl Pts',(24.7493903499091,33.2186639686628,3.22959079971438));
#55617=CARTESIAN_POINT('Ctrl Pts',(2.09999999999999,23.6060638408349,31.0445557091894));
#55618=CARTESIAN_POINT('Ctrl Pts',(2.73333333333333,23.6060638408349,31.0445557091894));
#55619=CARTESIAN_POINT('Ctrl Pts',(3.36473746642767,23.6061425297296,31.0444589629108));
#55620=CARTESIAN_POINT('Ctrl Pts',(4.12100628902188,23.6061623402403,31.0444327844504));
#55621=CARTESIAN_POINT('Ctrl Pts',(4.34473822453751,23.6025854765119,31.0472157503264));
#55622=CARTESIAN_POINT('Ctrl Pts',(4.82888984385421,23.5855175045883,31.0605268452774));
#55623=CARTESIAN_POINT('Ctrl Pts',(5.71370711452889,23.5437141746986,31.0931560738764));
#55624=CARTESIAN_POINT('Ctrl Pts',(6.55597759920728,23.5404210020823,31.0957493072636));
#55625=CARTESIAN_POINT('Ctrl Pts',(7.21859239432847,23.6253815004145,31.0291339441544));
#55626=CARTESIAN_POINT('Ctrl Pts',(7.34671727862973,23.642483368885,31.0159694149875));
#55627=CARTESIAN_POINT('Ctrl Pts',(7.55204160508675,23.6720771362965,30.9936033840678));
#55628=CARTESIAN_POINT('Ctrl Pts',(7.75540399562257,23.703970579718,30.9698143809751));
#55629=CARTESIAN_POINT('Ctrl Pts',(8.1685462302919,23.7742182410811,30.9176848413218));
#55630=CARTESIAN_POINT('Ctrl Pts',(8.79790183526862,23.9043880616322,30.821062716188));
#55631=CARTESIAN_POINT('Ctrl Pts',(9.50487531095145,24.1078339771774,30.6630536225869));
#55632=CARTESIAN_POINT('Ctrl Pts',(10.0642822980701,24.3148700594436,30.4950542324297));
#55633=CARTESIAN_POINT('Ctrl Pts',(10.3400051840509,24.4345722367156,30.3953232126618));
#55634=CARTESIAN_POINT('Ctrl Pts',(11.1101689715184,24.7978712127453,30.0884174263745));
#55635=CARTESIAN_POINT('Ctrl Pts',(12.2544685115539,25.5868263762922,29.438979342731));
#55636=CARTESIAN_POINT('Ctrl Pts',(13.2428015568077,26.4868133212994,28.635622249399));
#55637=CARTESIAN_POINT('Ctrl Pts',(13.9963745203349,27.1666930320859,27.9669135540566));
#55638=CARTESIAN_POINT('Ctrl Pts',(14.5753856172388,27.7428627327012,27.3941772128234));
#55639=CARTESIAN_POINT('Ctrl Pts',(15.6192725488263,28.9287825114552,26.1637553334563));
#55640=CARTESIAN_POINT('Ctrl Pts',(16.3374308310286,29.8325152502563,25.1374605936698));
#55641=CARTESIAN_POINT('Ctrl Pts',(17.0806756556551,30.718544717149,24.0114822717043));
#55642=CARTESIAN_POINT('Ctrl Pts',(17.6370679821595,31.416219386984,23.0964177419519));
#55643=CARTESIAN_POINT('Ctrl Pts',(18.6628584031467,32.7782054424402,21.1652477398233));
#55644=CARTESIAN_POINT('Ctrl Pts',(19.3755147763723,33.7367580996321,19.6024095311255));
#55645=CARTESIAN_POINT('Ctrl Pts',(20.1166717274658,34.6367097434079,17.9070970149883));
#55646=CARTESIAN_POINT('Ctrl Pts',(20.6600520901303,35.3025782886813,16.5762223315018));
#55647=CARTESIAN_POINT('Ctrl Pts',(21.677838645414,36.5163042963535,13.7987400828508));
#55648=CARTESIAN_POINT('Ctrl Pts',(22.3918362246611,37.2627527205715,11.6092337566466));
#55649=CARTESIAN_POINT('Ctrl Pts',(23.5225266677048,38.1911612590058,8.07535257523923));
#55650=CARTESIAN_POINT('Ctrl Pts',(24.157514841919,38.568193396505,5.91726457407121));
#55651=CARTESIAN_POINT('Ctrl Pts',(24.7577717974218,38.7717600341623,3.69372680454323));
#55652=CARTESIAN_POINT('',(24.5,9.59462155813272,1.51911333283482));
#55653=CARTESIAN_POINT('Ctrl Pts',(24.5,9.59462155813272,1.51911333283482));
#55654=CARTESIAN_POINT('Ctrl Pts',(23.827493934627,9.68464608987473,2.15212334066745));
#55655=CARTESIAN_POINT('Ctrl Pts',(23.3366347313572,9.74051511545228,2.59560605191541));
#55656=CARTESIAN_POINT('Ctrl Pts',(22.5855494187791,9.82470025254072,3.28291903755242));
#55657=CARTESIAN_POINT('Ctrl Pts',(22.2454144273139,9.86282416523817,3.59417422067011));
#55658=CARTESIAN_POINT('Ctrl Pts',(21.8382660745341,9.90378919285794,3.97801649612276));
#55659=CARTESIAN_POINT('Ctrl Pts',(21.3802156951389,9.94963128619511,4.41815755084702));
#55660=CARTESIAN_POINT('Ctrl Pts',(20.7694693293574,10.0107553309835,5.0050243272898));
#55661=CARTESIAN_POINT('Ctrl Pts',(20.1629003033668,10.0735609707631,5.59681393246532));
#55662=CARTESIAN_POINT('Ctrl Pts',(19.5574857571565,10.1644416730676,6.18557724500365));
#55663=CARTESIAN_POINT('Ctrl Pts',(18.6418529412372,10.3018902261041,7.07602662905619));
#55664=CARTESIAN_POINT('Ctrl Pts',(17.7734813314344,10.4379301691332,8.01241566165726));
#55665=CARTESIAN_POINT('Ctrl Pts',(16.962125309797,10.6309468689446,8.90231278422673));
#55666=CARTESIAN_POINT('Ctrl Pts',(16.8133360661241,10.6663429318508,9.06550516375273));
#55667=CARTESIAN_POINT('Ctrl Pts',(16.6656205365448,10.7036307121431,9.22838814972182));
#55668=CARTESIAN_POINT('Ctrl Pts',(16.5183901926363,10.7431465007573,9.39150480786586));
#55669=CARTESIAN_POINT('Ctrl Pts',(15.7264522886848,10.9556981390766,10.2688936729658));
#55670=CARTESIAN_POINT('Ctrl Pts',(14.946225971903,11.1777141128626,11.2250100584366));
#55671=CARTESIAN_POINT('Ctrl Pts',(14.296315041466,11.4147273043975,12.0335028146403));
#55672=CARTESIAN_POINT('Ctrl Pts',(13.9908350933947,11.5261314584923,12.4135215427682));
#55673=CARTESIAN_POINT('Ctrl Pts',(13.7077063566838,11.640829979709,12.7699839203788));
#55674=CARTESIAN_POINT('Ctrl Pts',(13.4460198946299,11.7567579012083,13.1013811331617));
#55675=CARTESIAN_POINT('Ctrl Pts',(12.8373295403739,12.0264096327183,13.8722207297729));
#55676=CARTESIAN_POINT('Ctrl Pts',(12.3530827406682,12.2595769009129,14.5291392283553));
#55677=CARTESIAN_POINT('Ctrl Pts',(11.9770275685189,12.457891446445,15.0431152888451));
#55678=CARTESIAN_POINT('Ctrl Pts',(11.6553972427396,12.6275047814291,15.4827058064633));
#55679=CARTESIAN_POINT('Ctrl Pts',(11.368420561445,12.7915939796411,15.8816900946671));
#55680=CARTESIAN_POINT('Ctrl Pts',(11.0710856781132,12.9780838956265,16.2988272964875));
#55681=CARTESIAN_POINT('Ctrl Pts',(10.8141787015525,13.1392172276392,16.659247359313));
#55682=CARTESIAN_POINT('Ctrl Pts',(10.5576802661763,13.3127876314479,17.0222174418464));
#55683=CARTESIAN_POINT('Ctrl Pts',(10.2957959918397,13.5071054931829,17.3951211088922));
#55684=CARTESIAN_POINT('Ctrl Pts',(9.71459276345088,13.9383576898262,18.2227111416047));
#55685=CARTESIAN_POINT('Ctrl Pts',(9.09527967376,14.4765717245283,19.1169834509677));
#55686=CARTESIAN_POINT('Ctrl Pts',(8.43168033652509,15.1490772897656,20.1368903834754));
#55687=CARTESIAN_POINT('Ctrl Pts',(7.97964340480164,15.6071810509049,20.8316403245095));
#55688=CARTESIAN_POINT('Ctrl Pts',(7.52291961074447,16.1149117861986,21.5633911686948));
#55689=CARTESIAN_POINT('Ctrl Pts',(7.10363554125516,16.615783022346,22.2694187973217));
#55690=CARTESIAN_POINT('Ctrl Pts',(6.56327799554258,17.2612870411659,23.1793206618854));
#55691=CARTESIAN_POINT('Ctrl Pts',(6.08559840021217,17.920031801205,24.0135115916133));
#55692=CARTESIAN_POINT('Ctrl Pts',(5.61708670826502,18.6215531549853,24.8770749330837));
#55693=CARTESIAN_POINT('Ctrl Pts',(5.04102956502363,19.4841066278815,25.9388666451068));
#55694=CARTESIAN_POINT('Ctrl Pts',(4.50102820502663,20.3869529589021,27.0079183407073));
#55695=CARTESIAN_POINT('Ctrl Pts',(4.,21.2644490398942,28.1082636227258));
#55696=CARTESIAN_POINT('Ctrl Pts',(3.72183418897234,21.7516260223353,28.7191642361292));
#55697=CARTESIAN_POINT('Ctrl Pts',(3.45538353518276,22.241089434693,29.3329319419627));
#55698=CARTESIAN_POINT('Ctrl Pts',(3.2,22.7328514723457,29.9495820327475));
#55699=CARTESIAN_POINT('',(24.5,26.7974275967278,3.30119284473541));
#55700=CARTESIAN_POINT('Ctrl Pts',(24.5,26.7974275967278,3.30119284473543));
#55701=CARTESIAN_POINT('Ctrl Pts',(24.5,25.566267318827,3.1648258977828));
#55702=CARTESIAN_POINT('Ctrl Pts',(24.5,24.3558799941678,3.03166854152344));
#55703=CARTESIAN_POINT('Ctrl Pts',(24.5,19.3537663513507,2.48621193714647));
#55704=CARTESIAN_POINT('Ctrl Pts',(24.5,14.0423469702365,1.915931263191));
#55705=CARTESIAN_POINT('Ctrl Pts',(24.5,9.59462155813271,1.51911333283482));
#55706=CARTESIAN_POINT('',(10.2670750393577,21.2938329649397,26.7016219748491));
#55707=CARTESIAN_POINT('Ctrl Pts',(10.2670750393577,21.2938329649397,26.7016219748491));
#55708=CARTESIAN_POINT('Ctrl Pts',(11.2293198185888,21.1087322437254,25.7230189888652));
#55709=CARTESIAN_POINT('Ctrl Pts',(12.092802582344,21.2018541927487,24.7466295176431));
#55710=CARTESIAN_POINT('Ctrl Pts',(14.3080979519049,21.7464694747342,22.1165033038735));
#55711=CARTESIAN_POINT('Ctrl Pts',(14.8952017874601,21.9942012642266,21.3805031040621));
#55712=CARTESIAN_POINT('Ctrl Pts',(17.0803363586062,23.1363413672538,18.2402856712274));
#55713=CARTESIAN_POINT('Ctrl Pts',(17.6922811489506,23.4905403046472,17.2880492021451));
#55714=CARTESIAN_POINT('Ctrl Pts',(19.0755427322033,24.3513474737146,14.9508913369539));
#55715=CARTESIAN_POINT('Ctrl Pts',(20.2687424742408,25.0945348989029,12.841709283693));
#55716=CARTESIAN_POINT('Ctrl Pts',(22.3267279388309,26.1951510699121,8.4493984325661));
#55717=CARTESIAN_POINT('Ctrl Pts',(23.4192562717209,26.6465650740303,6.03375707119804));
#55718=CARTESIAN_POINT('Ctrl Pts',(24.5,26.7974275967278,3.30119284473544));
#55719=CARTESIAN_POINT('Ctrl Pts',(6.,23.5490023259382,31.0876903203335));
#55720=CARTESIAN_POINT('Ctrl Pts',(7.51604047332546,22.2062790886928,29.3988225104988));
#55721=CARTESIAN_POINT('Ctrl Pts',(9.08449301626627,21.6187658580324,27.8817144423825));
#55722=CARTESIAN_POINT('Ctrl Pts',(9.8624969752411,21.383187532576,27.1095892261748));
#55723=CARTESIAN_POINT('Ctrl Pts',(10.0667253012217,21.3323729308866,26.9053776680083));
#55724=CARTESIAN_POINT('Ctrl Pts',(10.2670750393577,21.2938329649397,26.7016219748491));
#55725=CARTESIAN_POINT('Origin',(24.5,5.29966331579924,6.64556760097825));
#55726=CARTESIAN_POINT('',(24.5,9.71413754081038,0.));
#55727=CARTESIAN_POINT('Ctrl Pts',(24.5,9.71413754081038,-6.93889390390723E-17));
#55728=CARTESIAN_POINT('Ctrl Pts',(24.5,9.71413754081038,0.274177179878995));
#55729=CARTESIAN_POINT('Ctrl Pts',(24.5,9.70252976905084,0.548413945873121));
#55730=CARTESIAN_POINT('Ctrl Pts',(24.5,9.65945653318739,1.05563169561816));
#55731=CARTESIAN_POINT('Ctrl Pts',(24.5,9.63118849993238,1.28815889347686));
#55732=CARTESIAN_POINT('Ctrl Pts',(24.5,9.59462155813272,1.51911333283482));
#55733=CARTESIAN_POINT('',(24.5,9.66248492718882,-1.00042650586162));
#55734=CARTESIAN_POINT('Ctrl Pts',(24.5,9.66248492718882,-1.00042650586162));
#55735=CARTESIAN_POINT('Ctrl Pts',(24.5,9.69691073862103,-0.667929433741795));
#55736=CARTESIAN_POINT('Ctrl Pts',(24.5,9.71413754081038,-0.334008932195348));
#55737=CARTESIAN_POINT('Ctrl Pts',(24.5,9.71413754081038,1.38777878078145E-16));
#55738=CARTESIAN_POINT('',(24.5,26.9302749158019,-1.93914748261464));
#55739=CARTESIAN_POINT('Ctrl Pts',(24.5,9.66248492718882,-1.00042650586161));
#55740=CARTESIAN_POINT('Ctrl Pts',(24.5,13.9671155781194,-1.16922793892204));
#55741=CARTESIAN_POINT('Ctrl Pts',(24.5,19.7062898477147,-1.49576285895545));
#55742=CARTESIAN_POINT('Ctrl Pts',(24.5,26.9302749158019,-1.93914748261464));
#55743=CARTESIAN_POINT('Origin',(24.5,0.,0.));
#55744=CARTESIAN_POINT('Ctrl Pts',(24.5,26.9302748955208,-1.93914776427185));
#55745=CARTESIAN_POINT('Ctrl Pts',(24.5,27.9515281336428,12.2436963424502));
#55746=CARTESIAN_POINT('Ctrl Pts',(24.5,16.8342246501858,21.1094500266368));
#55747=CARTESIAN_POINT('Ctrl Pts',(24.5,-4.275225376451,37.9436746768226));
#55748=CARTESIAN_POINT('Ctrl Pts',(24.5,-21.1094500266368,16.8342246501858));
#55749=CARTESIAN_POINT('Ctrl Pts',(24.5,-37.9436746768226,-4.275225376451));
#55750=CARTESIAN_POINT('Ctrl Pts',(24.5,-16.8342246501858,-21.1094500266368));
#55751=CARTESIAN_POINT('Ctrl Pts',(24.5,4.275225376451,-37.9436746768226));
#55752=CARTESIAN_POINT('Ctrl Pts',(24.5,21.1094500266368,-16.8342246501858));
#55753=CARTESIAN_POINT('Ctrl Pts',(24.5,26.329027592611,-10.2890814031001));
#55754=CARTESIAN_POINT('Ctrl Pts',(24.5,26.9302748955208,-1.93914776427185));
#55755=CARTESIAN_POINT('Ctrl Pts',(24.3078118955742,26.9629766761956,-1.94150249645076));
#55756=CARTESIAN_POINT('Ctrl Pts',(24.3078118955742,27.9854700353166,12.2585640210755));
#55757=CARTESIAN_POINT('Ctrl Pts',(24.3078118955742,16.854666666633,21.1350835044834));
#55758=CARTESIAN_POINT('Ctrl Pts',(24.3078118955742,-4.28041683785042,37.9897501711163));
#55759=CARTESIAN_POINT('Ctrl Pts',(24.3078118955742,-21.1350835044834,16.854666666633));
#55760=CARTESIAN_POINT('Ctrl Pts',(24.3078118955742,-37.9897501711163,-4.28041683785042));
#55761=CARTESIAN_POINT('Ctrl Pts',(24.3078118955742,-16.854666666633,-21.1350835044834));
#55762=CARTESIAN_POINT('Ctrl Pts',(24.3078118955742,4.28041683785042,-37.9897501711163));
#55763=CARTESIAN_POINT('Ctrl Pts',(24.3078118955742,21.1350835044834,-16.854666666633));
#55764=CARTESIAN_POINT('Ctrl Pts',(24.3078118955742,26.3609992709193,-10.3015755675561));
#55765=CARTESIAN_POINT('Ctrl Pts',(24.3078118955742,26.9629766761956,-1.94150249645076));
#55766=CARTESIAN_POINT('Ctrl Pts',(23.9225830034177,27.0325342181099,-1.94651107331878));
#55767=CARTESIAN_POINT('Ctrl Pts',(23.9225830034177,28.0576653469971,12.2901879619685));
#55768=CARTESIAN_POINT('Ctrl Pts',(23.9225830034177,16.8981473697169,21.1896065816043));
#55769=CARTESIAN_POINT('Ctrl Pts',(23.9225830034177,-4.29145921188742,38.0877539513211));
#55770=CARTESIAN_POINT('Ctrl Pts',(23.9225830034177,-21.1896065816043,16.8981473697169));
#55771=CARTESIAN_POINT('Ctrl Pts',(23.9225830034177,-38.0877539513211,-4.29145921188742));
#55772=CARTESIAN_POINT('Ctrl Pts',(23.9225830034177,-16.8981473697169,-21.1896065816043));
#55773=CARTESIAN_POINT('Ctrl Pts',(23.9225830034177,4.29145921188742,-38.0877539513211));
#55774=CARTESIAN_POINT('Ctrl Pts',(23.9225830034177,21.1896065816043,-16.8981473697169));
#55775=CARTESIAN_POINT('Ctrl Pts',(23.9225830034177,26.4290038660243,-10.3281509817965));
#55776=CARTESIAN_POINT('Ctrl Pts',(23.9225830034177,27.0325342181099,-1.94651107331878));
#55777=CARTESIAN_POINT('Ctrl Pts',(23.3421815947946,27.1493324306214,-1.95492127312333));
#55778=CARTESIAN_POINT('Ctrl Pts',(23.3421815947946,28.178892795868,12.3432896051147));
#55779=CARTESIAN_POINT('Ctrl Pts',(23.3421815947946,16.9711584086233,21.2811595286045));
#55780=CARTESIAN_POINT('Ctrl Pts',(23.3421815947946,-4.31000111998121,38.2523179372279));
#55781=CARTESIAN_POINT('Ctrl Pts',(23.3421815947946,-21.2811595286045,16.9711584086233));
#55782=CARTESIAN_POINT('Ctrl Pts',(23.3421815947946,-38.2523179372279,-4.31000111998121));
#55783=CARTESIAN_POINT('Ctrl Pts',(23.3421815947946,-16.9711584086233,-21.2811595286045));
#55784=CARTESIAN_POINT('Ctrl Pts',(23.3421815947946,4.31000111998121,-38.2523179372279));
#55785=CARTESIAN_POINT('Ctrl Pts',(23.3421815947946,21.2811595286045,-16.9711584086233));
#55786=CARTESIAN_POINT('Ctrl Pts',(23.3421815947946,26.5431944330316,-10.372775343075));
#55787=CARTESIAN_POINT('Ctrl Pts',(23.3421815947946,27.1493324306214,-1.95492127312333));
#55788=CARTESIAN_POINT('Ctrl Pts',(22.5631762070947,27.3300892320692,-1.96793689025922));
#55789=CARTESIAN_POINT('Ctrl Pts',(22.5631762070947,28.3665042792493,12.4254696570208));
#55790=CARTESIAN_POINT('Ctrl Pts',(22.5631762070947,17.0841502222764,21.4228467814061));
#55791=CARTESIAN_POINT('Ctrl Pts',(22.5631762070947,-4.33869655912967,38.5069970036825));
#55792=CARTESIAN_POINT('Ctrl Pts',(22.5631762070947,-21.4228467814061,17.0841502222764));
#55793=CARTESIAN_POINT('Ctrl Pts',(22.5631762070947,-38.5069970036825,-4.33869655912967));
#55794=CARTESIAN_POINT('Ctrl Pts',(22.5631762070947,-17.0841502222764,-21.4228467814061));
#55795=CARTESIAN_POINT('Ctrl Pts',(22.5631762070947,4.33869655912967,-38.5069970036825));
#55796=CARTESIAN_POINT('Ctrl Pts',(22.5631762070947,21.4228467814061,-17.0841502222764));
#55797=CARTESIAN_POINT('Ctrl Pts',(22.5631762070947,26.7199156448029,-10.4418359617087));
#55798=CARTESIAN_POINT('Ctrl Pts',(22.5631762070947,27.3300892320692,-1.96793689025922));
#55799=CARTESIAN_POINT('Ctrl Pts',(21.5808622776984,27.5984753948965,-1.98726236798372));
#55800=CARTESIAN_POINT('Ctrl Pts',(21.5808622776984,28.6450682155646,12.5474898997744));
#55801=CARTESIAN_POINT('Ctrl Pts',(21.5808622776984,17.2519195070522,21.633222810393));
#55802=CARTESIAN_POINT('Ctrl Pts',(21.5808622776984,-4.38130330334076,38.8851423174452));
#55803=CARTESIAN_POINT('Ctrl Pts',(21.5808622776984,-21.633222810393,17.2519195070522));
#55804=CARTESIAN_POINT('Ctrl Pts',(21.5808622776984,-38.8851423174452,-4.38130330334076));
#55805=CARTESIAN_POINT('Ctrl Pts',(21.5808622776984,-17.2519195070522,-21.633222810393));
#55806=CARTESIAN_POINT('Ctrl Pts',(21.5808622776984,4.38130330334076,-38.8851423174452));
#55807=CARTESIAN_POINT('Ctrl Pts',(21.5808622776984,21.633222810393,-17.2519195070522));
#55808=CARTESIAN_POINT('Ctrl Pts',(21.5808622776984,26.9823097983707,-10.5443765814205));
#55809=CARTESIAN_POINT('Ctrl Pts',(21.5808622776984,27.5984753948965,-1.98726236798372));
#55810=CARTESIAN_POINT('Ctrl Pts',(20.5902243197586,27.9104505809399,-2.00972652725693));
#55811=CARTESIAN_POINT('Ctrl Pts',(20.5902243197586,28.9688741634622,12.6893276440645));
#55812=CARTESIAN_POINT('Ctrl Pts',(20.5902243197586,17.4469364679823,21.8777663445708));
#55813=CARTESIAN_POINT('Ctrl Pts',(20.5902243197586,-4.43082987658852,39.3247028125531));
#55814=CARTESIAN_POINT('Ctrl Pts',(20.5902243197586,-21.8777663445708,17.4469364679823));
#55815=CARTESIAN_POINT('Ctrl Pts',(20.5902243197586,-39.3247028125531,-4.43082987658852));
#55816=CARTESIAN_POINT('Ctrl Pts',(20.5902243197586,-17.4469364679823,-21.8777663445708));
#55817=CARTESIAN_POINT('Ctrl Pts',(20.5902243197586,4.43082987658852,-39.3247028125531));
#55818=CARTESIAN_POINT('Ctrl Pts',(20.5902243197586,21.8777663445708,-17.4469364679823));
#55819=CARTESIAN_POINT('Ctrl Pts',(20.5902243197586,27.2873198034082,-10.6635709861342));
#55820=CARTESIAN_POINT('Ctrl Pts',(20.5902243197586,27.9104505809399,-2.00972652725693));
#55821=CARTESIAN_POINT('Ctrl Pts',(19.591895069338,28.2674884777214,-2.03543548277225));
#55822=CARTESIAN_POINT('Ctrl Pts',(19.591895069338,29.3394516958262,12.8516528935431));
#55823=CARTESIAN_POINT('Ctrl Pts',(19.591895069338,17.6701223131461,22.157632542334));
#55824=CARTESIAN_POINT('Ctrl Pts',(19.591895069338,-4.48751022918786,39.8277548554801));
#55825=CARTESIAN_POINT('Ctrl Pts',(19.591895069338,-22.157632542334,17.6701223131461));
#55826=CARTESIAN_POINT('Ctrl Pts',(19.591895069338,-39.8277548554801,-4.48751022918786));
#55827=CARTESIAN_POINT('Ctrl Pts',(19.591895069338,-17.6701223131461,-22.157632542334));
#55828=CARTESIAN_POINT('Ctrl Pts',(19.591895069338,4.48751022918786,-39.8277548554801));
#55829=CARTESIAN_POINT('Ctrl Pts',(19.591895069338,22.157632542334,-17.6701223131461));
#55830=CARTESIAN_POINT('Ctrl Pts',(19.591895069338,27.6363864457815,-10.7999822184082));
#55831=CARTESIAN_POINT('Ctrl Pts',(19.591895069338,28.2674884777214,-2.03543548277225));
#55832=CARTESIAN_POINT('Ctrl Pts',(18.5871162949016,28.6712831397633,-2.06451121702157));
#55833=CARTESIAN_POINT('Ctrl Pts',(18.5871162949016,29.7585591093251,13.0352358404652));
#55834=CARTESIAN_POINT('Ctrl Pts',(18.5871162949016,17.9225360029332,22.47414929801));
#55835=CARTESIAN_POINT('Ctrl Pts',(18.5871162949016,-4.55161329507687,40.3966853009432));
#55836=CARTESIAN_POINT('Ctrl Pts',(18.5871162949016,-22.47414929801,17.9225360029332));
#55837=CARTESIAN_POINT('Ctrl Pts',(18.5871162949016,-40.3966853009432,-4.55161329507687));
#55838=CARTESIAN_POINT('Ctrl Pts',(18.5871162949016,-17.9225360029332,-22.47414929801));
#55839=CARTESIAN_POINT('Ctrl Pts',(18.5871162949016,4.55161329507687,-40.3966853009432));
#55840=CARTESIAN_POINT('Ctrl Pts',(18.5871162949016,22.47414929801,-17.9225360029332));
#55841=CARTESIAN_POINT('Ctrl Pts',(18.5871162949016,28.0311659584264,-10.9542575150402));
#55842=CARTESIAN_POINT('Ctrl Pts',(18.5871162949016,28.6712831397633,-2.06451121702157));
#55843=CARTESIAN_POINT('Ctrl Pts',(17.577868433379,29.1235503979937,-2.09707728053386));
#55844=CARTESIAN_POINT('Ctrl Pts',(17.577868433379,30.2279773028415,13.2408565776054));
#55845=CARTESIAN_POINT('Ctrl Pts',(17.577868433379,18.2052501102534,22.8286615754873));
#55846=CARTESIAN_POINT('Ctrl Pts',(17.577868433379,-4.62341146523393,41.0339116857407));
#55847=CARTESIAN_POINT('Ctrl Pts',(17.577868433379,-22.8286615754873,18.2052501102534));
#55848=CARTESIAN_POINT('Ctrl Pts',(17.577868433379,-41.0339116857407,-4.62341146523393));
#55849=CARTESIAN_POINT('Ctrl Pts',(17.577868433379,-18.2052501102534,-22.8286615754873));
#55850=CARTESIAN_POINT('Ctrl Pts',(17.577868433379,4.62341146523393,-41.0339116857407));
#55851=CARTESIAN_POINT('Ctrl Pts',(17.577868433379,22.8286615754873,-18.2052501102534));
#55852=CARTESIAN_POINT('Ctrl Pts',(17.577868433379,28.4733358645036,-11.1270524328026));
#55853=CARTESIAN_POINT('Ctrl Pts',(17.577868433379,29.1235503979937,-2.09707728053386));
#55854=CARTESIAN_POINT('Ctrl Pts',(16.5668667015923,29.6257248204915,-2.1332369711586));
#55855=CARTESIAN_POINT('Ctrl Pts',(16.5668667015923,30.7491952463233,13.4691673231831));
#55856=CARTESIAN_POINT('Ctrl Pts',(16.5668667015923,18.5191613894625,23.2222938691605));
#55857=CARTESIAN_POINT('Ctrl Pts',(16.5668667015923,-4.703132479698,41.7414552586229));
#55858=CARTESIAN_POINT('Ctrl Pts',(16.5668667015923,-23.2222938691605,18.5191613894625));
#55859=CARTESIAN_POINT('Ctrl Pts',(16.5668667015923,-41.7414552586229,-4.703132479698));
#55860=CARTESIAN_POINT('Ctrl Pts',(16.5668667015923,-18.5191613894625,-23.2222938691605));
#55861=CARTESIAN_POINT('Ctrl Pts',(16.5668667015923,4.703132479698,-41.7414552586229));
#55862=CARTESIAN_POINT('Ctrl Pts',(16.5668667015923,23.2222938691605,-18.5191613894625));
#55863=CARTESIAN_POINT('Ctrl Pts',(16.5668667015923,28.964298703819,-11.3189150681333));
#55864=CARTESIAN_POINT('Ctrl Pts',(16.5668667015923,29.6257248204915,-2.1332369711586));
#55865=CARTESIAN_POINT('Ctrl Pts',(15.5576189940876,30.1786037710718,-2.17304770406385));
#55866=CARTESIAN_POINT('Ctrl Pts',(15.5576189940876,31.3230405413156,13.7205305941226));
#55867=CARTESIAN_POINT('Ctrl Pts',(15.5576189940876,18.8647682759327,23.6556711972172));
#55868=CARTESIAN_POINT('Ctrl Pts',(15.5576189940876,-4.79090292128452,42.5204394731498));
#55869=CARTESIAN_POINT('Ctrl Pts',(15.5576189940876,-23.6556711972172,18.8647682759327));
#55870=CARTESIAN_POINT('Ctrl Pts',(15.5576189940876,-42.5204394731498,-4.79090292128452));
#55871=CARTESIAN_POINT('Ctrl Pts',(15.5576189940876,-18.8647682759327,-23.6556711972172));
#55872=CARTESIAN_POINT('Ctrl Pts',(15.5576189940876,4.79090292128452,-42.5204394731498));
#55873=CARTESIAN_POINT('Ctrl Pts',(15.5576189940876,23.6556711972172,-18.8647682759327));
#55874=CARTESIAN_POINT('Ctrl Pts',(15.5576189940876,29.5048340381843,-11.5301500648294));
#55875=CARTESIAN_POINT('Ctrl Pts',(15.5576189940876,30.1786037710718,-2.17304770406385));
#55876=CARTESIAN_POINT('Ctrl Pts',(14.5544447688713,30.7820095946451,-2.2164966869751));
#55877=CARTESIAN_POINT('Ctrl Pts',(14.5544447688713,31.9493287956705,13.9948656205477));
#55878=CARTESIAN_POINT('Ctrl Pts',(14.5544447688713,19.2419597167431,24.1286543036994));
#55879=CARTESIAN_POINT('Ctrl Pts',(14.5544447688713,-4.88669458695623,43.3706140204425));
#55880=CARTESIAN_POINT('Ctrl Pts',(14.5544447688713,-24.1286543036994,19.2419597167431));
#55881=CARTESIAN_POINT('Ctrl Pts',(14.5544447688713,-43.3706140204425,-4.88669458695623));
#55882=CARTESIAN_POINT('Ctrl Pts',(14.5544447688713,-19.2419597167431,-24.1286543036994));
#55883=CARTESIAN_POINT('Ctrl Pts',(14.5544447688713,4.88669458695623,-43.3706140204425));
#55884=CARTESIAN_POINT('Ctrl Pts',(14.5544447688713,24.1286543036994,-19.2419597167431));
#55885=CARTESIAN_POINT('Ctrl Pts',(14.5544447688713,30.0947681788509,-11.760689547324));
#55886=CARTESIAN_POINT('Ctrl Pts',(14.5544447688713,30.7820095946451,-2.2164966869751));
#55887=CARTESIAN_POINT('Ctrl Pts',(13.5625963827217,31.4342268363874,-2.26346039644524));
#55888=CARTESIAN_POINT('Ctrl Pts',(13.5625963827217,32.6262795008725,14.2913924806776));
#55889=CARTESIAN_POINT('Ctrl Pts',(13.5625963827217,19.6496633740883,24.6398985195302));
#55890=CARTESIAN_POINT('Ctrl Pts',(13.5625963827217,-4.99023514544193,44.2895618936185));
#55891=CARTESIAN_POINT('Ctrl Pts',(13.5625963827217,-24.6398985195302,19.6496633740883));
#55892=CARTESIAN_POINT('Ctrl Pts',(13.5625963827217,-44.2895618936185,-4.99023514544193));
#55893=CARTESIAN_POINT('Ctrl Pts',(13.5625963827217,-19.6496633740883,-24.6398985195302));
#55894=CARTESIAN_POINT('Ctrl Pts',(13.5625963827217,4.99023514544193,-44.2895618936185));
#55895=CARTESIAN_POINT('Ctrl Pts',(13.5625963827217,24.6398985195302,-19.6496633740883));
#55896=CARTESIAN_POINT('Ctrl Pts',(13.5625963827217,30.7324239703655,-12.0098781025402));
#55897=CARTESIAN_POINT('Ctrl Pts',(13.5625963827217,31.4342268363874,-2.26346039644524));
#55898=CARTESIAN_POINT('Ctrl Pts',(12.5880795783847,32.1319937999165,-2.31370396999061));
#55899=CARTESIAN_POINT('Ctrl Pts',(12.5880795783847,33.3505072700831,14.6086282627996));
#55900=CARTESIAN_POINT('Ctrl Pts',(12.5880795783847,20.0858403482595,25.1868471453426));
#55901=CARTESIAN_POINT('Ctrl Pts',(12.5880795783847,-5.10100679708313,45.2726874936021));
#55902=CARTESIAN_POINT('Ctrl Pts',(12.5880795783847,-25.1868471453426,20.0858403482595));
#55903=CARTESIAN_POINT('Ctrl Pts',(12.5880795783847,-45.2726874936021,-5.10100679708313));
#55904=CARTESIAN_POINT('Ctrl Pts',(12.5880795783847,-20.0858403482595,-25.1868471453426));
#55905=CARTESIAN_POINT('Ctrl Pts',(12.5880795783847,5.10100679708313,-45.2726874936021));
#55906=CARTESIAN_POINT('Ctrl Pts',(12.5880795783847,25.1868471453426,-20.0858403482595));
#55907=CARTESIAN_POINT('Ctrl Pts',(12.5880795783847,31.4146125372199,-12.276469554577));
#55908=CARTESIAN_POINT('Ctrl Pts',(12.5880795783847,32.1319937999165,-2.31370396999061));
#55909=CARTESIAN_POINT('Ctrl Pts',(11.6370973936883,32.8712141860011,-2.36693244851678));
#55910=CARTESIAN_POINT('Ctrl Pts',(11.6370973936883,34.1177604637013,14.9447106077621));
#55911=CARTESIAN_POINT('Ctrl Pts',(11.6370973936883,20.5479300259039,25.766289273552));
#55912=CARTESIAN_POINT('Ctrl Pts',(11.6370973936883,-5.21835924764815,46.3142192994559));
#55913=CARTESIAN_POINT('Ctrl Pts',(11.6370973936883,-25.766289273552,20.5479300259039));
#55914=CARTESIAN_POINT('Ctrl Pts',(11.6370973936883,-46.3142192994559,-5.21835924764815));
#55915=CARTESIAN_POINT('Ctrl Pts',(11.6370973936883,-20.5479300259039,-25.766289273552));
#55916=CARTESIAN_POINT('Ctrl Pts',(11.6370973936883,5.21835924764815,-46.3142192994559));
#55917=CARTESIAN_POINT('Ctrl Pts',(11.6370973936883,25.766289273552,-20.5479300259039));
#55918=CARTESIAN_POINT('Ctrl Pts',(11.6370973936883,32.1373290344614,-12.5588988560514));
#55919=CARTESIAN_POINT('Ctrl Pts',(11.6370973936883,32.8712141860011,-2.36693244851678));
#55920=CARTESIAN_POINT('Ctrl Pts',(10.7155646400367,33.6474328922446,-2.42282503686346));
#55921=CARTESIAN_POINT('Ctrl Pts',(10.7155646400367,34.9234150323828,15.297614028594));
#55922=CARTESIAN_POINT('Ctrl Pts',(10.7155646400367,21.0331475043468,26.3747327466602));
#55923=CARTESIAN_POINT('Ctrl Pts',(10.7155646400367,-5.34158524231336,47.4078802510069));
#55924=CARTESIAN_POINT('Ctrl Pts',(10.7155646400367,-26.3747327466602,21.0331475043468));
#55925=CARTESIAN_POINT('Ctrl Pts',(10.7155646400367,-47.4078802510069,-5.34158524231336));
#55926=CARTESIAN_POINT('Ctrl Pts',(10.7155646400367,-21.0331475043468,-26.3747327466602));
#55927=CARTESIAN_POINT('Ctrl Pts',(10.7155646400367,5.34158524231336,-47.4078802510069));
#55928=CARTESIAN_POINT('Ctrl Pts',(10.7155646400367,26.3747327466602,-21.0331475043468));
#55929=CARTESIAN_POINT('Ctrl Pts',(10.7155646400367,32.8962178246381,-12.8554638739033));
#55930=CARTESIAN_POINT('Ctrl Pts',(10.7155646400367,33.6474328922446,-2.42282503686346));
#55931=CARTESIAN_POINT('Ctrl Pts',(9.82859575068344,34.456339097072,-2.48107132898941));
#55932=CARTESIAN_POINT('Ctrl Pts',(9.82859575068344,35.76299667904,15.66537863478));
#55933=CARTESIAN_POINT('Ctrl Pts',(9.82859575068344,21.5387980714436,27.0087985025163));
#55934=CARTESIAN_POINT('Ctrl Pts',(9.82859575068344,-5.47000043107262,48.5475965739599));
#55935=CARTESIAN_POINT('Ctrl Pts',(9.82859575068344,-27.0087985025163,21.5387980714436));
#55936=CARTESIAN_POINT('Ctrl Pts',(9.82859575068344,-48.5475965739599,-5.47000043107262));
#55937=CARTESIAN_POINT('Ctrl Pts',(9.82859575068344,-21.5387980714436,-27.0087985025163));
#55938=CARTESIAN_POINT('Ctrl Pts',(9.82859575068344,5.47000043107262,-48.5475965739599));
#55939=CARTESIAN_POINT('Ctrl Pts',(9.82859575068344,27.0087985025163,-21.5387980714436));
#55940=CARTESIAN_POINT('Ctrl Pts',(9.82859575068344,33.6870643298952,-13.1645175995423));
#55941=CARTESIAN_POINT('Ctrl Pts',(9.82859575068344,34.456339097072,-2.48107132898941));
#55942=CARTESIAN_POINT('Ctrl Pts',(8.97989469943246,35.2942458419803,-2.54140584088581));
#55943=CARTESIAN_POINT('Ctrl Pts',(8.97989469943246,36.6326786278703,16.0463281716024));
#55944=CARTESIAN_POINT('Ctrl Pts',(8.97989469943246,22.0625769943999,27.6655964976071));
#55945=CARTESIAN_POINT('Ctrl Pts',(8.97989469943246,-5.60301950320719,49.7281734920069));
#55946=CARTESIAN_POINT('Ctrl Pts',(8.97989469943246,-27.6655964976071,22.0625769943999));
#55947=CARTESIAN_POINT('Ctrl Pts',(8.97989469943246,-49.7281734920069,-5.60301950320719));
#55948=CARTESIAN_POINT('Ctrl Pts',(8.97989469943246,-22.0625769943999,-27.6655964976071));
#55949=CARTESIAN_POINT('Ctrl Pts',(8.97989469943246,5.60301950320719,-49.7281734920069));
#55950=CARTESIAN_POINT('Ctrl Pts',(8.97989469943246,27.6655964976071,-22.0625769943999));
#55951=CARTESIAN_POINT('Ctrl Pts',(8.97989469943246,34.506263907037,-13.4846513798329));
#55952=CARTESIAN_POINT('Ctrl Pts',(8.97989469943246,35.2942458419803,-2.54140584088581));
#55953=CARTESIAN_POINT('Ctrl Pts',(8.1713316609345,36.1584562373913,-2.60363437968177));
#55954=CARTESIAN_POINT('Ctrl Pts',(8.1713316609345,37.5296617175133,16.4392365135503));
#55955=CARTESIAN_POINT('Ctrl Pts',(8.1713316609345,22.6027984365433,28.3430127596098));
#55956=CARTESIAN_POINT('Ctrl Pts',(8.1713316609345,-5.74021432306655,50.9458111961531));
#55957=CARTESIAN_POINT('Ctrl Pts',(8.1713316609345,-28.3430127596098,22.6027984365433));
#55958=CARTESIAN_POINT('Ctrl Pts',(8.1713316609345,-50.9458111961531,-5.74021432306655));
#55959=CARTESIAN_POINT('Ctrl Pts',(8.1713316609345,-22.6027984365433,-28.3430127596098));
#55960=CARTESIAN_POINT('Ctrl Pts',(8.1713316609345,5.74021432306655,-50.9458111961531));
#55961=CARTESIAN_POINT('Ctrl Pts',(8.1713316609345,28.3430127596098,-22.6027984365433));
#55962=CARTESIAN_POINT('Ctrl Pts',(8.1713316609345,35.3511798774411,-13.8148348310708));
#55963=CARTESIAN_POINT('Ctrl Pts',(8.1713316609345,36.1584562373913,-2.60363437968177));
#55964=CARTESIAN_POINT('Ctrl Pts',(7.40358438374929,37.0470976022564,-2.66762210066133));
#55965=CARTESIAN_POINT('Ctrl Pts',(7.40358438374929,38.4520022508761,16.843252256834));
#55966=CARTESIAN_POINT('Ctrl Pts',(7.40358438374929,23.1582917773139,29.039579376772));
#55967=CARTESIAN_POINT('Ctrl Pts',(7.40358438374929,-5.88128759945806,52.1978711540859));
#55968=CARTESIAN_POINT('Ctrl Pts',(7.40358438374929,-29.039579376772,23.1582917773139));
#55969=CARTESIAN_POINT('Ctrl Pts',(7.40358438374929,-52.1978711540859,-5.88128759945806));
#55970=CARTESIAN_POINT('Ctrl Pts',(7.40358438374929,-23.1582917773139,-29.039579376772));
#55971=CARTESIAN_POINT('Ctrl Pts',(7.40358438374929,5.88128759945806,-52.1978711540859));
#55972=CARTESIAN_POINT('Ctrl Pts',(7.40358438374929,29.039579376772,-23.1582917773139));
#55973=CARTESIAN_POINT('Ctrl Pts',(7.40358438374929,36.2199813696739,-14.1543524697407));
#55974=CARTESIAN_POINT('Ctrl Pts',(7.40358438374929,37.0470976022564,-2.66762210066133));
#55975=CARTESIAN_POINT('Ctrl Pts',(6.82198164612729,37.7766337007775,-2.72015325007928));
#55976=CARTESIAN_POINT('Ctrl Pts',(6.82198164612729,39.209203908172,17.1749316955253));
#55977=CARTESIAN_POINT('Ctrl Pts',(6.82198164612729,23.6143277673129,29.6114304207775));
#55978=CARTESIAN_POINT('Ctrl Pts',(6.82198164612729,-5.99710265346455,53.2257581880904));
#55979=CARTESIAN_POINT('Ctrl Pts',(6.82198164612729,-29.6114304207775,23.6143277673129));
#55980=CARTESIAN_POINT('Ctrl Pts',(6.82198164612729,-53.2257581880904,-5.99710265346455));
#55981=CARTESIAN_POINT('Ctrl Pts',(6.82198164612729,-23.6143277673129,-29.6114304207775));
#55982=CARTESIAN_POINT('Ctrl Pts',(6.82198164612729,5.99710265346455,-53.2257581880904));
#55983=CARTESIAN_POINT('Ctrl Pts',(6.82198164612729,29.6114304207775,-23.6143277673129));
#55984=CARTESIAN_POINT('Ctrl Pts',(6.82198164612729,36.9332297914701,-14.4330817561407));
#55985=CARTESIAN_POINT('Ctrl Pts',(6.82198164612729,37.7766337007775,-2.72015325007928));
#55986=CARTESIAN_POINT('Ctrl Pts',(6.40395249919757,38.3340026926033,-2.76028729395988));
#55987=CARTESIAN_POINT('Ctrl Pts',(6.40395249919757,39.787709516313,17.4283363381844));
#55988=CARTESIAN_POINT('Ctrl Pts',(6.40395249919757,23.9627413968747,30.048327293349));
#55989=CARTESIAN_POINT('Ctrl Pts',(6.40395249919757,-6.08558589647433,54.0110686902236));
#55990=CARTESIAN_POINT('Ctrl Pts',(6.40395249919757,-30.048327293349,23.9627413968747));
#55991=CARTESIAN_POINT('Ctrl Pts',(6.40395249919757,-54.0110686902236,-6.08558589647433));
#55992=CARTESIAN_POINT('Ctrl Pts',(6.40395249919757,-23.9627413968747,-30.048327293349));
#55993=CARTESIAN_POINT('Ctrl Pts',(6.40395249919757,6.08558589647433,-54.0110686902236));
#55994=CARTESIAN_POINT('Ctrl Pts',(6.40395249919757,30.048327293349,-23.9627413968747));
#55995=CARTESIAN_POINT('Ctrl Pts',(6.40395249919757,37.4781549220891,-14.646032234764));
#55996=CARTESIAN_POINT('Ctrl Pts',(6.40395249919757,38.3340026926033,-2.76028729395988));
#55997=CARTESIAN_POINT('Ctrl Pts',(6.13331019225912,38.7101044651372,-2.78736896743619));
#55998=CARTESIAN_POINT('Ctrl Pts',(6.13331019225912,40.1780738670996,17.5993288703672));
#55999=CARTESIAN_POINT('Ctrl Pts',(6.13331019225912,24.1978441485076,30.3431368191721));
#56000=CARTESIAN_POINT('Ctrl Pts',(6.13331019225912,-6.14529267066447,54.5409809676797));
#56001=CARTESIAN_POINT('Ctrl Pts',(6.13331019225912,-30.3431368191721,24.1978441485076));
#56002=CARTESIAN_POINT('Ctrl Pts',(6.13331019225912,-54.5409809676797,-6.14529267066447));
#56003=CARTESIAN_POINT('Ctrl Pts',(6.13331019225912,-24.1978441485076,-30.3431368191721));
#56004=CARTESIAN_POINT('Ctrl Pts',(6.13331019225912,6.14529267066447,-54.5409809676797));
#56005=CARTESIAN_POINT('Ctrl Pts',(6.13331019225912,30.3431368191721,-24.1978441485076));
#56006=CARTESIAN_POINT('Ctrl Pts',(6.13331019225912,37.8458598187191,-14.7897270826059));
#56007=CARTESIAN_POINT('Ctrl Pts',(6.13331019225912,38.7101044651372,-2.78736896743619));
#56008=CARTESIAN_POINT('Ctrl Pts',(6.,38.8992859601968,-2.80099121505934));
#56009=CARTESIAN_POINT('Ctrl Pts',(6.,40.374429526373,17.6853391613169));
#56010=CARTESIAN_POINT('Ctrl Pts',(6.,24.3161022724906,30.4914278162532));
#56011=CARTESIAN_POINT('Ctrl Pts',(6.,-6.17532554376255,54.8075300887438));
#56012=CARTESIAN_POINT('Ctrl Pts',(6.,-30.4914278162532,24.3161022724906));
#56013=CARTESIAN_POINT('Ctrl Pts',(6.,-54.8075300887438,-6.17532554376255));
#56014=CARTESIAN_POINT('Ctrl Pts',(6.,-24.3161022724906,-30.4914278162532));
#56015=CARTESIAN_POINT('Ctrl Pts',(6.,6.17532554376255,-54.8075300887438));
#56016=CARTESIAN_POINT('Ctrl Pts',(6.,30.4914278162532,-24.3161022724906));
#56017=CARTESIAN_POINT('Ctrl Pts',(6.,38.0308176337714,-14.8620064711446));
#56018=CARTESIAN_POINT('Ctrl Pts',(6.,38.8992859601968,-2.80099121505934));
#56019=CARTESIAN_POINT('Ctrl Pts',(24.5,26.9302749158019,-1.93914748261463));
#56020=CARTESIAN_POINT('Ctrl Pts',(23.5178991898112,27.3082121037186,0.976729634524829));
#56021=CARTESIAN_POINT('Ctrl Pts',(22.3947886245986,27.292619732882,3.87921761795231));
#56022=CARTESIAN_POINT('Ctrl Pts',(21.1743874927566,26.982974376293,6.70537618061041));
#56023=CARTESIAN_POINT('Ctrl Pts',(20.5031871793443,26.8126745830804,8.25971635902861));
#56024=CARTESIAN_POINT('Ctrl Pts',(19.8411792966425,26.5351229273328,9.80106908179735));
#56025=CARTESIAN_POINT('Ctrl Pts',(19.1295827650289,26.1983895630578,11.3029592184858));
#56026=CARTESIAN_POINT('Ctrl Pts',(18.8261415870933,26.054798687939,11.9433998220584));
#56027=CARTESIAN_POINT('Ctrl Pts',(18.5104994276281,25.8995059296898,12.5819483349197));
#56028=CARTESIAN_POINT('Ctrl Pts',(18.2016639423759,25.7504555752122,13.1744818344469));
#56029=CARTESIAN_POINT('Ctrl Pts',(17.6747132403633,25.4961383329334,14.1854924159764));
#56030=CARTESIAN_POINT('Ctrl Pts',(17.2016343370993,25.234137247781,15.0794665673296));
#56031=CARTESIAN_POINT('Ctrl Pts',(16.872935292646,25.0561420993951,15.6789596275853));
#56032=CARTESIAN_POINT('Ctrl Pts',(16.6342454025477,24.9268881720619,16.1142907764943));
#56033=CARTESIAN_POINT('Ctrl Pts',(16.5014949770664,24.8554353423937,16.3490513597629));
#56034=CARTESIAN_POINT('Ctrl Pts',(16.3424569562979,24.7713057233,16.6271276317564));
#56035=CARTESIAN_POINT('Ctrl Pts',(15.993118510103,24.5865089667059,17.2379421546763));
#56036=CARTESIAN_POINT('Ctrl Pts',(15.6312480487537,24.4025072310428,17.842238323798));
#56037=CARTESIAN_POINT('Ctrl Pts',(15.2503296894305,24.2327051324582,18.4383275548583));
#56038=CARTESIAN_POINT('Ctrl Pts',(14.7484414179076,24.0089782375114,19.2237194545343));
#56039=CARTESIAN_POINT('Ctrl Pts',(14.2669345517206,23.7821697043648,19.9782075196444));
#56040=CARTESIAN_POINT('Ctrl Pts',(13.7912435751455,23.5895005313304,20.6850186190487));
#56041=CARTESIAN_POINT('Ctrl Pts',(13.5533980868579,23.4931659448132,21.0384241687508));
#56042=CARTESIAN_POINT('Ctrl Pts',(13.3161115657262,23.4047239475972,21.3818868765805));
#56043=CARTESIAN_POINT('Ctrl Pts',(13.0766514227367,23.3278398910295,21.7168098997672));
#56044=CARTESIAN_POINT('Ctrl Pts',(12.9188702359555,23.2771806976525,21.9374919365312));
#56045=CARTESIAN_POINT('Ctrl Pts',(12.760152636041,23.2315393210602,22.1544736717658));
#56046=CARTESIAN_POINT('Ctrl Pts',(12.5997389313808,23.1920716652435,22.3682108834076));
#56047=CARTESIAN_POINT('Ctrl Pts',(12.5166971934814,23.1716403514927,22.4788567259566));
#56048=CARTESIAN_POINT('Ctrl Pts',(12.4397215765388,23.1541581369635,22.5801970534995));
#56049=CARTESIAN_POINT('Ctrl Pts',(12.3478597934844,23.135666399718,22.6992700418308));
#56050=CARTESIAN_POINT('Ctrl Pts',(11.9116121727781,23.0478499421241,23.2647424953666));
#56051=CARTESIAN_POINT('Ctrl Pts',(10.7144663992386,22.7494221199229,24.8644224033158));
#56052=CARTESIAN_POINT('Ctrl Pts',(9.56604185022483,22.9954826851968,26.1397381390956));
#56053=CARTESIAN_POINT('Ctrl Pts',(9.07284645450935,23.1011543533655,26.687427449212));
#56054=CARTESIAN_POINT('Ctrl Pts',(8.57333454993108,23.2942014462969,27.200709354055));
#56055=CARTESIAN_POINT('Ctrl Pts',(8.00348148263612,23.5910390275427,27.7971969467927));
#56056=CARTESIAN_POINT('Ctrl Pts',(7.63919428966324,23.7807969413751,28.1785106630337));
#56057=CARTESIAN_POINT('Ctrl Pts',(7.24388644384776,24.0230902706367,28.5986372279999));
#56058=CARTESIAN_POINT('Ctrl Pts',(6.94254646282495,24.224686334644,28.9297076532741));
#56059=CARTESIAN_POINT('Ctrl Pts',(6.9143356486524,24.243559333442,28.9607017690026));
#56060=CARTESIAN_POINT('Ctrl Pts',(6.8866963504054,24.2622024336213,28.9911617715523));
#56061=CARTESIAN_POINT('Ctrl Pts',(6.85962514029879,24.2805982312137,29.0210854076675));
#56062=CARTESIAN_POINT('Ctrl Pts',(6.4400006207374,24.5657472029905,29.4849247180966));
#56063=CARTESIAN_POINT('Ctrl Pts',(6.15412442492902,24.8218403166442,29.7963100363863));
#56064=CARTESIAN_POINT('Ctrl Pts',(6.,24.9583551264995,29.9679914138325));
#56065=CARTESIAN_POINT('Ctrl Pts',(2.09999999999999,6.75186083300313,7.02307776555548));
#56066=CARTESIAN_POINT('Ctrl Pts',(2.73333333333332,6.75186083300313,7.02307776555548));
#56067=CARTESIAN_POINT('Ctrl Pts',(3.36743543952785,6.75183177141242,7.02311078228488));
#56068=CARTESIAN_POINT('Ctrl Pts',(4.25158796552468,6.75181603731384,7.02312801127863));
#56069=CARTESIAN_POINT('Ctrl Pts',(4.76433649975501,6.74814750679869,7.02673437605219));
#56070=CARTESIAN_POINT('Ctrl Pts',(5.76343391408727,6.73741073604095,7.03732555416368));
#56071=CARTESIAN_POINT('Ctrl Pts',(6.49282537630615,6.73758367376741,7.037202522005));
#56072=CARTESIAN_POINT('Ctrl Pts',(7.02318175216964,6.75287253869763,7.02196831057607));
#56073=CARTESIAN_POINT('Ctrl Pts',(7.14965217142688,6.75668208482572,7.01826529498886));
#56074=CARTESIAN_POINT('Ctrl Pts',(7.33684129238207,6.76279679807891,7.01243069802765));
#56075=CARTESIAN_POINT('Ctrl Pts',(7.52512455501651,6.76947383888626,7.00614752519297));
#56076=CARTESIAN_POINT('Ctrl Pts',(7.90060975758075,6.78395137112435,6.99260449234284));
#56077=CARTESIAN_POINT('Ctrl Pts',(8.46111568560639,6.81022178214197,6.96807725147119));
#56078=CARTESIAN_POINT('Ctrl Pts',(9.0649318004708,6.84956899053507,6.92958262645135));
#56079=CARTESIAN_POINT('Ctrl Pts',(9.52832373202331,6.8881411385333,6.89002179737934));
#56080=CARTESIAN_POINT('Ctrl Pts',(9.75191892912806,6.90990515851168,6.8670359880604));
#56081=CARTESIAN_POINT('Ctrl Pts',(10.3693392952773,6.9748999842145,6.79732375550614));
#56082=CARTESIAN_POINT('Ctrl Pts',(11.1025266505574,7.08737323265808,6.68172752983343));
#56083=CARTESIAN_POINT('Ctrl Pts',(12.0426911089806,7.26677575080387,6.48709341783056));
#56084=CARTESIAN_POINT('Ctrl Pts',(12.499722130795,7.3594489260534,6.38005936900193));
#56085=CARTESIAN_POINT('Ctrl Pts',(13.0012698578513,7.46041400993639,6.25761556166667));
#56086=CARTESIAN_POINT('Ctrl Pts',(13.5007180547461,7.57082916437595,6.12120949789655));
#56087=CARTESIAN_POINT('Ctrl Pts',(14.4711813662111,7.81513023260049,5.8104756958165));
#56088=CARTESIAN_POINT('Ctrl Pts',(15.1519969212886,8.00485912494299,5.54793502163326));
#56089=CARTESIAN_POINT('Ctrl Pts',(15.8847991347671,8.19595990286687,5.25102186548175));
#56090=CARTESIAN_POINT('Ctrl Pts',(16.3872971149165,8.33252921025319,5.0295981284336));
#56091=CARTESIAN_POINT('Ctrl Pts',(17.3643064948304,8.61235770932072,4.54363935262331));
#56092=CARTESIAN_POINT('Ctrl Pts',(18.0507589576911,8.80903169625677,4.14872708560309));
#56093=CARTESIAN_POINT('Ctrl Pts',(18.6483680950931,8.96006699947368,3.79286285126064));
#56094=CARTESIAN_POINT('Ctrl Pts',(18.9044434426896,9.02412347576023,3.63492996765564));
#56095=CARTESIAN_POINT('Ctrl Pts',(19.4121342092306,9.15024194464128,3.30386179229804));
#56096=CARTESIAN_POINT('Ctrl Pts',(20.2666508045858,9.35464157539163,2.70286662391449));
#56097=CARTESIAN_POINT('Ctrl Pts',(20.9684455414225,9.49456951845435,2.15371671276294));
#56098=CARTESIAN_POINT('Ctrl Pts',(22.6563363377109,9.73492158768411,0.813372498605933));
#56099=CARTESIAN_POINT('Ctrl Pts',(23.7241254823848,9.75490295250663,-0.169822791436732));
#56100=CARTESIAN_POINT('Ctrl Pts',(24.6950729185804,9.64173030469554,-1.20656804782375));
#56101=CARTESIAN_POINT('Ctrl Pts',(2.09999999999999,9.3606448320155,10.2943894298461));
#56102=CARTESIAN_POINT('Ctrl Pts',(2.73333333333332,9.3606448320155,10.2943894298461));
#56103=CARTESIAN_POINT('Ctrl Pts',(3.36780698153315,9.36061008131633,10.2944242783898));
#56104=CARTESIAN_POINT('Ctrl Pts',(4.25233231972465,9.36058995842981,10.2944437790382));
#56105=CARTESIAN_POINT('Ctrl Pts',(4.76998297705552,9.35518711781965,10.2994669666885));
#56106=CARTESIAN_POINT('Ctrl Pts',(5.76686224093397,9.33945332871658,10.3141494019522));
#56107=CARTESIAN_POINT('Ctrl Pts',(6.48740862524488,9.3398050883223,10.3138785526291));
#56108=CARTESIAN_POINT('Ctrl Pts',(7.0061130401074,9.36188714675425,10.2930675210009));
#56109=CARTESIAN_POINT('Ctrl Pts',(7.13243989848971,9.36746702831866,10.2879375119643));
#56110=CARTESIAN_POINT('Ctrl Pts',(7.31802664417342,9.37637918639968,10.279898312667));
#56111=CARTESIAN_POINT('Ctrl Pts',(7.5049699541733,9.38611799055235,10.2712361195763));
#56112=CARTESIAN_POINT('Ctrl Pts',(7.87708859115843,9.40720946420748,10.252591673622));
#56113=CARTESIAN_POINT('Ctrl Pts',(8.43135921890744,9.44543964035596,10.2188661544007));
#56114=CARTESIAN_POINT('Ctrl Pts',(9.02534159402558,9.50254288340357,10.1660693364088));
#56115=CARTESIAN_POINT('Ctrl Pts',(9.47887696115925,9.55835634760375,10.1119599660578));
#56116=CARTESIAN_POINT('Ctrl Pts',(9.69679911910571,9.58977777808015,10.0805889174017));
#56117=CARTESIAN_POINT('Ctrl Pts',(10.2969891502313,9.68347956139936,9.98557550000814));
#56118=CARTESIAN_POINT('Ctrl Pts',(11.0126425549871,9.84610155233706,9.82790341081631));
#56119=CARTESIAN_POINT('Ctrl Pts',(11.9399904897231,10.1078040659667,9.56020772764343));
#56120=CARTESIAN_POINT('Ctrl Pts',(12.3932824025843,10.243807857196,9.41208245856254));
#56121=CARTESIAN_POINT('Ctrl Pts',(12.8921398066301,10.3924251346088,9.24213401999094));
#56122=CARTESIAN_POINT('Ctrl Pts',(13.3792097412206,10.5529434552443,9.05554252681676));
#56123=CARTESIAN_POINT('Ctrl Pts',(14.3391036396927,10.9117909671869,8.6266652169495));
#56124=CARTESIAN_POINT('Ctrl Pts',(15.0151384665191,11.1929514360095,8.26160510734747));
#56125=CARTESIAN_POINT('Ctrl Pts',(15.7464682979872,11.4782327955903,7.84625032020446));
#56126=CARTESIAN_POINT('Ctrl Pts',(16.2431121097701,11.6811022331859,7.53930863556436));
#56127=CARTESIAN_POINT('Ctrl Pts',(17.2175647308135,12.1010374264068,6.86032054045774));
#56128=CARTESIAN_POINT('Ctrl Pts',(17.902233226602,12.3991880824743,6.30544044686097));
#56129=CARTESIAN_POINT('Ctrl Pts',(18.4992586458284,12.6303406807946,5.80396967282006));
#56130=CARTESIAN_POINT('Ctrl Pts',(18.7551887763511,12.7288128543355,5.58197357903342));
#56131=CARTESIAN_POINT('Ctrl Pts',(19.2633718823391,12.9238162767338,5.1151491998172));
#56132=CARTESIAN_POINT('Ctrl Pts',(20.11959381405,13.2431270393567,4.26551003148763));
#56133=CARTESIAN_POINT('Ctrl Pts',(20.8219603861067,13.4673930095846,3.48645537953313));
#56134=CARTESIAN_POINT('Ctrl Pts',(22.5090412631404,13.8688229753371,1.58275022437511));
#56135=CARTESIAN_POINT('Ctrl Pts',(23.5814142719244,13.9428296252028,0.176915545464796));
#56136=CARTESIAN_POINT('Ctrl Pts',(24.5630597774298,13.8254029813209,-1.32144457270545));
#56137=CARTESIAN_POINT('Ctrl Pts',(2.09999999999999,15.4478074963777,17.9274499798575));
#56138=CARTESIAN_POINT('Ctrl Pts',(2.73333333333332,15.4478074963777,17.9274499798575));
#56139=CARTESIAN_POINT('Ctrl Pts',(3.36868154479411,15.4477062395499,17.9275615025271));
#56140=CARTESIAN_POINT('Ctrl Pts',(4.25408340297134,15.4476482838215,17.9276224710576));
#56141=CARTESIAN_POINT('Ctrl Pts',(4.78315784529757,15.4380783144895,17.9360630069014));
#56142=CARTESIAN_POINT('Ctrl Pts',(5.77489961286181,15.410701705442,17.9602815974078));
#56143=CARTESIAN_POINT('Ctrl Pts',(6.47472773803472,15.4116671302561,17.9595561186054));
#56144=CARTESIAN_POINT('Ctrl Pts',(6.96650688012029,15.4484582579053,17.9266626909592));
#56145=CARTESIAN_POINT('Ctrl Pts',(7.09250370718804,15.4581514578408,17.9182183607075));
#56146=CARTESIAN_POINT('Ctrl Pts',(7.27439470054606,15.4734212590436,17.9051740564475));
#56147=CARTESIAN_POINT('Ctrl Pts',(7.45825749071973,15.4901434795058,17.8910941766856));
#56148=CARTESIAN_POINT('Ctrl Pts',(7.82264750929872,15.526250828117,17.8608873548829));
#56149=CARTESIAN_POINT('Ctrl Pts',(8.36272090805856,15.5913967531887,17.8065467726089));
#56150=CARTESIAN_POINT('Ctrl Pts',(8.9347937479117,15.6878654162987,17.7221276981452));
#56151=CARTESIAN_POINT('Ctrl Pts',(9.3673174608011,15.7812559606787,17.6363424287067));
#56152=CARTESIAN_POINT('Ctrl Pts',(9.57367322901424,15.8334515307549,17.5869341162243));
#56153=CARTESIAN_POINT('Ctrl Pts',(10.1399697938406,15.9882956088782,17.4380475272674));
#56154=CARTESIAN_POINT('Ctrl Pts',(10.8299043390251,16.260489724366,17.1894479356455));
#56155=CARTESIAN_POINT('Ctrl Pts',(11.7453472913653,16.7114886332834,16.7550898933566));
#56156=CARTESIAN_POINT('Ctrl Pts',(12.1960662260621,16.9479824207621,16.5125039644984));
#56157=CARTESIAN_POINT('Ctrl Pts',(12.6932389229874,17.2075602912353,16.2328252357149));
#56158=CARTESIAN_POINT('Ctrl Pts',(13.1762447636157,17.4848403459161,15.9305412231499));
#56159=CARTESIAN_POINT('Ctrl Pts',(14.1425321130376,18.1177228777731,15.2209165121274));
#56160=CARTESIAN_POINT('Ctrl Pts',(14.8241183447167,18.6162256731906,14.6135421497294));
#56161=CARTESIAN_POINT('Ctrl Pts',(15.557455076331,19.1224107044634,13.9219028509968));
#56162=CARTESIAN_POINT('Ctrl Pts',(16.0657546221985,19.488599800816,13.4050818951716));
#56163=CARTESIAN_POINT('Ctrl Pts',(17.0556206253738,20.2465726772756,12.2587322070762));
#56164=CARTESIAN_POINT('Ctrl Pts',(17.7495638140097,20.7856973165121,11.3220806623194));
#56165=CARTESIAN_POINT('Ctrl Pts',(18.3487436972501,21.2036838733817,10.4790901221427));
#56166=CARTESIAN_POINT('Ctrl Pts',(18.612025577843,21.3865661773176,10.0983329331232));
#56167=CARTESIAN_POINT('Ctrl Pts',(19.1297981766656,21.7465060383579,9.30187623430936));
#56168=CARTESIAN_POINT('Ctrl Pts',(20.0013796142357,22.3387585237374,7.85056974085133));
#56169=CARTESIAN_POINT('Ctrl Pts',(20.7092009017835,22.7574098818365,6.52651913010203));
#56170=CARTESIAN_POINT('Ctrl Pts',(22.4028783154293,23.5268367952951,3.29839169345834));
#56171=CARTESIAN_POINT('Ctrl Pts',(23.5047783389009,23.72392704974,0.858352285640053));
#56172=CARTESIAN_POINT('Ctrl Pts',(24.5021398191099,23.5781496343124,-1.7386710629416));
#56173=CARTESIAN_POINT('Ctrl Pts',(2.09999999999999,21.5349701607399,25.5605105298689));
#56174=CARTESIAN_POINT('Ctrl Pts',(2.73333333333332,21.5349701607399,25.5605105298689));
#56175=CARTESIAN_POINT('Ctrl Pts',(3.36960345513781,21.5349002841666,25.5605959908683));
#56176=CARTESIAN_POINT('Ctrl Pts',(4.25591992477685,21.5348462612853,25.5606536627902));
#56177=CARTESIAN_POINT('Ctrl Pts',(4.79634591585354,21.5209380941788,25.5726342271993));
#56178=CARTESIAN_POINT('Ctrl Pts',(5.78315002628676,21.4819997663131,25.6063230410257));
#56179=CARTESIAN_POINT('Ctrl Pts',(6.46185830361957,21.4843332331369,25.6044986864714));
#56180=CARTESIAN_POINT('Ctrl Pts',(6.92808305094846,21.5334571899302,25.5614101034119));
#56181=CARTESIAN_POINT('Ctrl Pts',(7.05377527389461,21.5472310736336,25.5496786575521));
#56182=CARTESIAN_POINT('Ctrl Pts',(7.23219486078965,21.5685063162337,25.5319120478409));
#56183=CARTESIAN_POINT('Ctrl Pts',(7.41321273751603,21.5918930045168,25.5126713718753));
#56184=CARTESIAN_POINT('Ctrl Pts',(7.7705268524474,21.6421607895434,25.4715965020036));
#56185=CARTESIAN_POINT('Ctrl Pts',(8.29815375808789,21.7325147198659,25.398009361424));
#56186=CARTESIAN_POINT('Ctrl Pts',(8.85328711712096,21.8650097997443,25.284732553375));
#56187=CARTESIAN_POINT('Ctrl Pts',(9.27295730736894,21.9928668513882,25.1699371658014));
#56188=CARTESIAN_POINT('Ctrl Pts',(9.47380151199838,22.0644476167393,25.1037197872101));
#56189=CARTESIAN_POINT('Ctrl Pts',(10.0271380233308,22.2775584376402,24.9035623188132));
#56190=CARTESIAN_POINT('Ctrl Pts',(10.7235476395157,22.6663647053173,24.558430698775));
#56191=CARTESIAN_POINT('Ctrl Pts',(11.6486669181634,23.3175089627325,23.9475902405967));
#56192=CARTESIAN_POINT('Ctrl Pts',(12.1028988094896,23.6583108207624,23.6066868035363));
#56193=CARTESIAN_POINT('Ctrl Pts',(12.6025767950092,24.0316536446078,23.2143131766174));
#56194=CARTESIAN_POINT('Ctrl Pts',(13.0990670491153,24.4407347347225,22.7806015625178));
#56195=CARTESIAN_POINT('Ctrl Pts',(14.0799893422845,25.3640794214541,21.7696578909302));
#56196=CARTESIAN_POINT('Ctrl Pts',(14.7677959112514,26.0861779345459,20.9084699059958));
#56197=CARTESIAN_POINT('Ctrl Pts',(15.5028074614617,26.813528756118,19.9358348179631));
#56198=CARTESIAN_POINT('Ctrl Pts',(16.0203496811134,27.3522973394796,19.1928465593642));
#56199=CARTESIAN_POINT('Ctrl Pts',(17.0171201090766,28.4511404827417,17.5639244958532));
#56200=CARTESIAN_POINT('Ctrl Pts',(17.714304440299,29.2299144264984,16.2370885097335));
#56201=CARTESIAN_POINT('Ctrl Pts',(18.3140531613331,29.8312119354217,15.0493462693643));
#56202=CARTESIAN_POINT('Ctrl Pts',(18.57968756902,30.0985577909357,14.5049533809244));
#56203=CARTESIAN_POINT('Ctrl Pts',(19.0999585250603,30.6210412827048,13.3731171359211));
#56204=CARTESIAN_POINT('Ctrl Pts',(19.9749323946637,31.4801887347959,11.312487340323));
#56205=CARTESIAN_POINT('Ctrl Pts',(20.6834701629094,32.0857292798578,9.4412256669571));
#56206=CARTESIAN_POINT('Ctrl Pts',(22.3781974839993,33.2055779658264,4.88365565359388));
#56207=CARTESIAN_POINT('Ctrl Pts',(23.4839952293235,33.5107154880467,1.41138142910537));
#56208=CARTESIAN_POINT('Ctrl Pts',(24.4831092917558,33.3234857380685,-2.27663628466851));
#56209=CARTESIAN_POINT('Ctrl Pts',(2.09999999999999,25.0133488260897,29.9222594155897));
#56210=CARTESIAN_POINT('Ctrl Pts',(2.73333333333332,25.0133488260897,29.9222594155897));
#56211=CARTESIAN_POINT('Ctrl Pts',(3.37014129606584,25.0132924435726,29.9223328973726));
#56212=CARTESIAN_POINT('Ctrl Pts',(4.25699410199334,25.013238335837,29.9223902997194));
#56213=CARTESIAN_POINT('Ctrl Pts',(4.80385941094312,24.9967713049222,29.9364568785204));
#56214=CARTESIAN_POINT('Ctrl Pts',(5.78794827479898,24.9512639339237,29.9755275020668));
#56215=CARTESIAN_POINT('Ctrl Pts',(6.45435104299642,24.9545226111096,29.9729588969588));
#56216=CARTESIAN_POINT('Ctrl Pts',(6.90670004343609,25.0100143695501,29.9245879403802));
#56217=CARTESIAN_POINT('Ctrl Pts',(7.03223126266704,25.0261109239331,29.9109859351108));
#56218=CARTESIAN_POINT('Ctrl Pts',(7.20878525009786,25.0507211873179,29.8905989614722));
#56219=CARTESIAN_POINT('Ctrl Pts',(7.38829842209633,25.0778317796888,29.8684778712122));
#56220=CARTESIAN_POINT('Ctrl Pts',(7.74190502196492,25.1359797339948,29.8213652053168));
#56221=CARTESIAN_POINT('Ctrl Pts',(8.2632681014489,25.2403315305653,29.7371132972183));
#56222=CARTESIAN_POINT('Ctrl Pts',(8.8109192265095,25.3930143580939,29.607688829357));
#56223=CARTESIAN_POINT('Ctrl Pts',(9.22605445875268,25.5408427231815,29.4761049361433));
#56224=CARTESIAN_POINT('Ctrl Pts',(9.42544001170288,25.6239850096632,29.3998849476721));
#56225=CARTESIAN_POINT('Ctrl Pts',(9.97639186033999,25.872447788317,29.1687118961422));
#56226=CARTESIAN_POINT('Ctrl Pts',(10.678683794887,26.3323373759567,28.7644662975497));
#56227=CARTESIAN_POINT('Ctrl Pts',(11.608086592202,27.1000368221737,28.0503563808397));
#56228=CARTESIAN_POINT('Ctrl Pts',(12.0639991264766,27.5009668734956,27.6525244186972));
#56229=CARTESIAN_POINT('Ctrl Pts',(12.5648057854578,27.9395988072145,27.1951930011199));
#56230=CARTESIAN_POINT('Ctrl Pts',(13.0664437052645,28.4251541066641,26.6848057324192));
#56231=CARTESIAN_POINT('Ctrl Pts',(14.0522205556053,29.5136387397641,25.5016363032258));
#56232=CARTESIAN_POINT('Ctrl Pts',(14.7426920220945,30.363042461303,24.4952111898507));
#56233=CARTESIAN_POINT('Ctrl Pts',(15.4785261743036,31.2164651060287,23.361578969675));
#56234=CARTESIAN_POINT('Ctrl Pts',(15.9996237268621,31.8527864292697,22.4901162997247));
#56235=CARTESIAN_POINT('Ctrl Pts',(16.9994960598944,33.1448484343335,20.5866268135138));
#56236=CARTESIAN_POINT('Ctrl Pts',(17.6982394889886,34.0600327208692,19.0367862273239));
#56237=CARTESIAN_POINT('Ctrl Pts',(18.298237166506,34.7657918685104,17.6517850800479));
#56238=CARTESIAN_POINT('Ctrl Pts',(18.5651091495521,35.0809389837737,17.0144403165625));
#56239=CARTESIAN_POINT('Ctrl Pts',(19.0868378278895,35.6957114841769,15.6915333342249));
#56240=CARTESIAN_POINT('Ctrl Pts',(19.9639555678099,36.7065474912943,13.2834565162864));
#56241=CARTESIAN_POINT('Ctrl Pts',(20.6728745268687,37.4184664294856,11.0994371626769));
#56242=CARTESIAN_POINT('Ctrl Pts',(22.3678114775293,38.7375406454473,5.7819285727616));
#56243=CARTESIAN_POINT('Ctrl Pts',(23.4757593035169,39.1032101474444,1.72082814260715));
#56244=CARTESIAN_POINT('Ctrl Pts',(24.4767076204831,38.8918379719078,-2.59074546980443));
#56245=CARTESIAN_POINT('Ctrl Pts',(23.5150942984749,10.0178765673373,5.37305195213122E-15));
#56246=CARTESIAN_POINT('Ctrl Pts',(23.8466145076669,9.90590446299441,-0.33185457075138));
#56247=CARTESIAN_POINT('Ctrl Pts',(24.1779623791327,9.78743932459042,-0.667296721337579));
#56248=CARTESIAN_POINT('Ctrl Pts',(24.5,9.66248492718882,-1.00042650586162));
#56249=CARTESIAN_POINT('Ctrl Pts',(2.79812873401693,24.7266395770977,29.5627865234736));
#56250=CARTESIAN_POINT('Ctrl Pts',(2.93275536019486,24.5313029720328,29.3178596635568));
#56251=CARTESIAN_POINT('Ctrl Pts',(3.06761573260946,24.3357274348763,29.0726369769539));
#56252=CARTESIAN_POINT('Ctrl Pts',(3.20253312029778,24.1401036614866,28.8273556403295));
#56253=CARTESIAN_POINT('Origin',(2.9,0.,0.));
#56254=CARTESIAN_POINT('Ctrl Pts',(27.,9.2,0.));
#56255=CARTESIAN_POINT('Ctrl Pts',(27.,9.2,9.2));
#56256=CARTESIAN_POINT('Ctrl Pts',(27.,0.,9.2));
#56257=CARTESIAN_POINT('Ctrl Pts',(27.,-9.2,9.2));
#56258=CARTESIAN_POINT('Ctrl Pts',(27.,-9.2,0.));
#56259=CARTESIAN_POINT('Ctrl Pts',(27.,-9.2,-9.2));
#56260=CARTESIAN_POINT('Ctrl Pts',(27.,0.,-9.2));
#56261=CARTESIAN_POINT('Ctrl Pts',(27.,9.2,-9.2));
#56262=CARTESIAN_POINT('Ctrl Pts',(27.,9.2,0.));
#56263=CARTESIAN_POINT('Ctrl Pts',(26.796570998452,9.22636560737002,0.));
#56264=CARTESIAN_POINT('Ctrl Pts',(26.796570998452,9.22636560737001,9.22636560737001));
#56265=CARTESIAN_POINT('Ctrl Pts',(26.796570998452,0.,9.22636560737002));
#56266=CARTESIAN_POINT('Ctrl Pts',(26.796570998452,-9.22636560737001,9.22636560737001));
#56267=CARTESIAN_POINT('Ctrl Pts',(26.796570998452,-9.22636560737002,0.));
#56268=CARTESIAN_POINT('Ctrl Pts',(26.796570998452,-9.22636560737001,-9.22636560737001));
#56269=CARTESIAN_POINT('Ctrl Pts',(26.796570998452,0.,-9.22636560737002));
#56270=CARTESIAN_POINT('Ctrl Pts',(26.796570998452,9.22636560737001,-9.22636560737001));
#56271=CARTESIAN_POINT('Ctrl Pts',(26.796570998452,9.22636560737002,0.));
#56272=CARTESIAN_POINT('Ctrl Pts',(26.3874085880356,9.28597940593777,0.));
#56273=CARTESIAN_POINT('Ctrl Pts',(26.3874085880356,9.28597940593777,9.28597940593777));
#56274=CARTESIAN_POINT('Ctrl Pts',(26.3874085880356,0.,9.28597940593777));
#56275=CARTESIAN_POINT('Ctrl Pts',(26.3874085880356,-9.28597940593777,9.28597940593777));
#56276=CARTESIAN_POINT('Ctrl Pts',(26.3874085880356,-9.28597940593777,0.));
#56277=CARTESIAN_POINT('Ctrl Pts',(26.3874085880356,-9.28597940593777,-9.28597940593777));
#56278=CARTESIAN_POINT('Ctrl Pts',(26.3874085880356,0.,-9.28597940593777));
#56279=CARTESIAN_POINT('Ctrl Pts',(26.3874085880356,9.28597940593777,-9.28597940593777));
#56280=CARTESIAN_POINT('Ctrl Pts',(26.3874085880356,9.28597940593777,0.));
#56281=CARTESIAN_POINT('Ctrl Pts',(25.7667517823113,9.39604887090672,0.));
#56282=CARTESIAN_POINT('Ctrl Pts',(25.7667517823113,9.39604887090672,9.39604887090672));
#56283=CARTESIAN_POINT('Ctrl Pts',(25.7667517823113,0.,9.39604887090672));
#56284=CARTESIAN_POINT('Ctrl Pts',(25.7667517823113,-9.39604887090672,9.39604887090672));
#56285=CARTESIAN_POINT('Ctrl Pts',(25.7667517823113,-9.39604887090672,0.));
#56286=CARTESIAN_POINT('Ctrl Pts',(25.7667517823113,-9.39604887090672,-9.39604887090672));
#56287=CARTESIAN_POINT('Ctrl Pts',(25.7667517823113,0.,-9.39604887090672));
#56288=CARTESIAN_POINT('Ctrl Pts',(25.7667517823113,9.39604887090672,-9.39604887090672));
#56289=CARTESIAN_POINT('Ctrl Pts',(25.7667517823113,9.39604887090672,0.));
#56290=CARTESIAN_POINT('Ctrl Pts',(24.9253466419639,9.58420457526839,0.));
#56291=CARTESIAN_POINT('Ctrl Pts',(24.9253466419639,9.58420457526839,9.58420457526839));
#56292=CARTESIAN_POINT('Ctrl Pts',(24.9253466419639,0.,9.58420457526839));
#56293=CARTESIAN_POINT('Ctrl Pts',(24.9253466419639,-9.58420457526839,9.58420457526839));
#56294=CARTESIAN_POINT('Ctrl Pts',(24.9253466419639,-9.58420457526839,0.));
#56295=CARTESIAN_POINT('Ctrl Pts',(24.9253466419639,-9.58420457526839,-9.58420457526839));
#56296=CARTESIAN_POINT('Ctrl Pts',(24.9253466419639,0.,-9.58420457526839));
#56297=CARTESIAN_POINT('Ctrl Pts',(24.9253466419639,9.58420457526839,-9.58420457526839));
#56298=CARTESIAN_POINT('Ctrl Pts',(24.9253466419639,9.58420457526839,0.));
#56299=CARTESIAN_POINT('Ctrl Pts',(23.8505404645239,9.89058631634017,0.));
#56300=CARTESIAN_POINT('Ctrl Pts',(23.8505404645239,9.89058631634017,9.89058631634017));
#56301=CARTESIAN_POINT('Ctrl Pts',(23.8505404645239,0.,9.89058631634017));
#56302=CARTESIAN_POINT('Ctrl Pts',(23.8505404645239,-9.89058631634017,9.89058631634017));
#56303=CARTESIAN_POINT('Ctrl Pts',(23.8505404645239,-9.89058631634017,0.));
#56304=CARTESIAN_POINT('Ctrl Pts',(23.8505404645239,-9.89058631634017,-9.89058631634017));
#56305=CARTESIAN_POINT('Ctrl Pts',(23.8505404645239,0.,-9.89058631634017));
#56306=CARTESIAN_POINT('Ctrl Pts',(23.8505404645239,9.89058631634017,-9.89058631634017));
#56307=CARTESIAN_POINT('Ctrl Pts',(23.8505404645239,9.89058631634017,0.));
#56308=CARTESIAN_POINT('Ctrl Pts',(22.7532142104752,10.273481509771,0.));
#56309=CARTESIAN_POINT('Ctrl Pts',(22.7532142104752,10.273481509771,10.273481509771));
#56310=CARTESIAN_POINT('Ctrl Pts',(22.7532142104752,0.,10.273481509771));
#56311=CARTESIAN_POINT('Ctrl Pts',(22.7532142104752,-10.273481509771,10.273481509771));
#56312=CARTESIAN_POINT('Ctrl Pts',(22.7532142104752,-10.273481509771,0.));
#56313=CARTESIAN_POINT('Ctrl Pts',(22.7532142104752,-10.273481509771,-10.273481509771));
#56314=CARTESIAN_POINT('Ctrl Pts',(22.7532142104752,0.,-10.273481509771));
#56315=CARTESIAN_POINT('Ctrl Pts',(22.7532142104752,10.273481509771,-10.273481509771));
#56316=CARTESIAN_POINT('Ctrl Pts',(22.7532142104752,10.273481509771,0.));
#56317=CARTESIAN_POINT('Ctrl Pts',(21.6347255505832,10.7430346646081,0.));
#56318=CARTESIAN_POINT('Ctrl Pts',(21.6347255505832,10.7430346646081,10.7430346646081));
#56319=CARTESIAN_POINT('Ctrl Pts',(21.6347255505832,0.,10.7430346646081));
#56320=CARTESIAN_POINT('Ctrl Pts',(21.6347255505832,-10.7430346646081,10.7430346646081));
#56321=CARTESIAN_POINT('Ctrl Pts',(21.6347255505832,-10.7430346646081,0.));
#56322=CARTESIAN_POINT('Ctrl Pts',(21.6347255505832,-10.7430346646081,-10.7430346646081));
#56323=CARTESIAN_POINT('Ctrl Pts',(21.6347255505832,0.,-10.7430346646081));
#56324=CARTESIAN_POINT('Ctrl Pts',(21.6347255505832,10.7430346646081,-10.7430346646081));
#56325=CARTESIAN_POINT('Ctrl Pts',(21.6347255505832,10.7430346646081,0.));
#56326=CARTESIAN_POINT('Ctrl Pts',(20.4975894383762,11.3145134298179,0.));
#56327=CARTESIAN_POINT('Ctrl Pts',(20.4975894383762,11.3145134298179,11.3145134298179));
#56328=CARTESIAN_POINT('Ctrl Pts',(20.4975894383762,0.,11.3145134298179));
#56329=CARTESIAN_POINT('Ctrl Pts',(20.4975894383762,-11.3145134298179,11.3145134298179));
#56330=CARTESIAN_POINT('Ctrl Pts',(20.4975894383762,-11.3145134298179,0.));
#56331=CARTESIAN_POINT('Ctrl Pts',(20.4975894383762,-11.3145134298179,-11.3145134298179));
#56332=CARTESIAN_POINT('Ctrl Pts',(20.4975894383762,0.,-11.3145134298179));
#56333=CARTESIAN_POINT('Ctrl Pts',(20.4975894383762,11.3145134298179,-11.3145134298179));
#56334=CARTESIAN_POINT('Ctrl Pts',(20.4975894383762,11.3145134298179,0.));
#56335=CARTESIAN_POINT('Ctrl Pts',(19.3456615791409,12.0038530129696,0.));
#56336=CARTESIAN_POINT('Ctrl Pts',(19.3456615791409,12.0038530129696,12.0038530129696));
#56337=CARTESIAN_POINT('Ctrl Pts',(19.3456615791409,0.,12.0038530129696));
#56338=CARTESIAN_POINT('Ctrl Pts',(19.3456615791409,-12.0038530129696,12.0038530129696));
#56339=CARTESIAN_POINT('Ctrl Pts',(19.3456615791409,-12.0038530129696,0.));
#56340=CARTESIAN_POINT('Ctrl Pts',(19.3456615791409,-12.0038530129696,-12.0038530129696));
#56341=CARTESIAN_POINT('Ctrl Pts',(19.3456615791409,0.,-12.0038530129696));
#56342=CARTESIAN_POINT('Ctrl Pts',(19.3456615791409,12.0038530129696,-12.0038530129696));
#56343=CARTESIAN_POINT('Ctrl Pts',(19.3456615791409,12.0038530129696,0.));
#56344=CARTESIAN_POINT('Ctrl Pts',(18.1843885347784,12.8237912132616,0.));
#56345=CARTESIAN_POINT('Ctrl Pts',(18.1843885347784,12.8237912132616,12.8237912132616));
#56346=CARTESIAN_POINT('Ctrl Pts',(18.1843885347784,0.,12.8237912132616));
#56347=CARTESIAN_POINT('Ctrl Pts',(18.1843885347784,-12.8237912132616,12.8237912132616));
#56348=CARTESIAN_POINT('Ctrl Pts',(18.1843885347784,-12.8237912132616,0.));
#56349=CARTESIAN_POINT('Ctrl Pts',(18.1843885347784,-12.8237912132616,-12.8237912132616));
#56350=CARTESIAN_POINT('Ctrl Pts',(18.1843885347784,0.,-12.8237912132616));
#56351=CARTESIAN_POINT('Ctrl Pts',(18.1843885347784,12.8237912132616,-12.8237912132616));
#56352=CARTESIAN_POINT('Ctrl Pts',(18.1843885347784,12.8237912132616,0.));
#56353=CARTESIAN_POINT('Ctrl Pts',(17.0210036637821,13.7799946040807,0.));
#56354=CARTESIAN_POINT('Ctrl Pts',(17.0210036637821,13.7799946040807,13.7799946040807));
#56355=CARTESIAN_POINT('Ctrl Pts',(17.0210036637821,0.,13.7799946040807));
#56356=CARTESIAN_POINT('Ctrl Pts',(17.0210036637821,-13.7799946040807,13.7799946040807));
#56357=CARTESIAN_POINT('Ctrl Pts',(17.0210036637821,-13.7799946040807,0.));
#56358=CARTESIAN_POINT('Ctrl Pts',(17.0210036637821,-13.7799946040807,-13.7799946040807));
#56359=CARTESIAN_POINT('Ctrl Pts',(17.0210036637821,0.,-13.7799946040807));
#56360=CARTESIAN_POINT('Ctrl Pts',(17.0210036637821,13.7799946040807,-13.7799946040807));
#56361=CARTESIAN_POINT('Ctrl Pts',(17.0210036637821,13.7799946040807,0.));
#56362=CARTESIAN_POINT('Ctrl Pts',(15.8649034353727,14.8662985491428,0.));
#56363=CARTESIAN_POINT('Ctrl Pts',(15.8649034353727,14.8662985491428,14.8662985491428));
#56364=CARTESIAN_POINT('Ctrl Pts',(15.8649034353727,0.,14.8662985491428));
#56365=CARTESIAN_POINT('Ctrl Pts',(15.8649034353727,-14.8662985491428,14.8662985491428));
#56366=CARTESIAN_POINT('Ctrl Pts',(15.8649034353727,-14.8662985491428,0.));
#56367=CARTESIAN_POINT('Ctrl Pts',(15.8649034353727,-14.8662985491428,-14.8662985491428));
#56368=CARTESIAN_POINT('Ctrl Pts',(15.8649034353727,0.,-14.8662985491428));
#56369=CARTESIAN_POINT('Ctrl Pts',(15.8649034353727,14.8662985491428,-14.8662985491428));
#56370=CARTESIAN_POINT('Ctrl Pts',(15.8649034353727,14.8662985491428,0.));
#56371=CARTESIAN_POINT('Ctrl Pts',(14.7267277676362,16.0674034956045,0.));
#56372=CARTESIAN_POINT('Ctrl Pts',(14.7267277676362,16.0674034956045,16.0674034956045));
#56373=CARTESIAN_POINT('Ctrl Pts',(14.7267277676362,0.,16.0674034956045));
#56374=CARTESIAN_POINT('Ctrl Pts',(14.7267277676362,-16.0674034956045,16.0674034956045));
#56375=CARTESIAN_POINT('Ctrl Pts',(14.7267277676362,-16.0674034956045,0.));
#56376=CARTESIAN_POINT('Ctrl Pts',(14.7267277676362,-16.0674034956045,-16.0674034956045));
#56377=CARTESIAN_POINT('Ctrl Pts',(14.7267277676362,0.,-16.0674034956045));
#56378=CARTESIAN_POINT('Ctrl Pts',(14.7267277676362,16.0674034956045,-16.0674034956045));
#56379=CARTESIAN_POINT('Ctrl Pts',(14.7267277676362,16.0674034956045,0.));
#56380=CARTESIAN_POINT('Ctrl Pts',(13.6172459538847,17.362757468191,0.));
#56381=CARTESIAN_POINT('Ctrl Pts',(13.6172459538847,17.362757468191,17.362757468191));
#56382=CARTESIAN_POINT('Ctrl Pts',(13.6172459538847,0.,17.362757468191));
#56383=CARTESIAN_POINT('Ctrl Pts',(13.6172459538847,-17.362757468191,17.362757468191));
#56384=CARTESIAN_POINT('Ctrl Pts',(13.6172459538847,-17.362757468191,0.));
#56385=CARTESIAN_POINT('Ctrl Pts',(13.6172459538847,-17.362757468191,-17.362757468191));
#56386=CARTESIAN_POINT('Ctrl Pts',(13.6172459538847,0.,-17.362757468191));
#56387=CARTESIAN_POINT('Ctrl Pts',(13.6172459538847,17.362757468191,-17.362757468191));
#56388=CARTESIAN_POINT('Ctrl Pts',(13.6172459538847,17.362757468191,0.));
#56389=CARTESIAN_POINT('Ctrl Pts',(12.5462580187496,18.7300247619529,0.));
#56390=CARTESIAN_POINT('Ctrl Pts',(12.5462580187496,18.7300247619529,18.7300247619529));
#56391=CARTESIAN_POINT('Ctrl Pts',(12.5462580187496,0.,18.7300247619529));
#56392=CARTESIAN_POINT('Ctrl Pts',(12.5462580187496,-18.7300247619529,18.7300247619529));
#56393=CARTESIAN_POINT('Ctrl Pts',(12.5462580187496,-18.7300247619529,0.));
#56394=CARTESIAN_POINT('Ctrl Pts',(12.5462580187496,-18.7300247619529,-18.7300247619529));
#56395=CARTESIAN_POINT('Ctrl Pts',(12.5462580187496,0.,-18.7300247619529));
#56396=CARTESIAN_POINT('Ctrl Pts',(12.5462580187496,18.7300247619529,-18.7300247619529));
#56397=CARTESIAN_POINT('Ctrl Pts',(12.5462580187496,18.7300247619529,0.));
#56398=CARTESIAN_POINT('Ctrl Pts',(11.5215838208076,20.1483844597128,0.));
#56399=CARTESIAN_POINT('Ctrl Pts',(11.5215838208076,20.1483844597128,20.1483844597128));
#56400=CARTESIAN_POINT('Ctrl Pts',(11.5215838208076,0.,20.1483844597128));
#56401=CARTESIAN_POINT('Ctrl Pts',(11.5215838208076,-20.1483844597128,20.1483844597128));
#56402=CARTESIAN_POINT('Ctrl Pts',(11.5215838208076,-20.1483844597128,0.));
#56403=CARTESIAN_POINT('Ctrl Pts',(11.5215838208076,-20.1483844597128,-20.1483844597128));
#56404=CARTESIAN_POINT('Ctrl Pts',(11.5215838208076,0.,-20.1483844597128));
#56405=CARTESIAN_POINT('Ctrl Pts',(11.5215838208076,20.1483844597128,-20.1483844597128));
#56406=CARTESIAN_POINT('Ctrl Pts',(11.5215838208076,20.1483844597128,0.));
#56407=CARTESIAN_POINT('Ctrl Pts',(10.5477031262524,21.602527086122,0.));
#56408=CARTESIAN_POINT('Ctrl Pts',(10.5477031262524,21.602527086122,21.602527086122));
#56409=CARTESIAN_POINT('Ctrl Pts',(10.5477031262524,0.,21.602527086122));
#56410=CARTESIAN_POINT('Ctrl Pts',(10.5477031262524,-21.602527086122,21.602527086122));
#56411=CARTESIAN_POINT('Ctrl Pts',(10.5477031262524,-21.602527086122,0.));
#56412=CARTESIAN_POINT('Ctrl Pts',(10.5477031262524,-21.602527086122,-21.602527086122));
#56413=CARTESIAN_POINT('Ctrl Pts',(10.5477031262524,0.,-21.602527086122));
#56414=CARTESIAN_POINT('Ctrl Pts',(10.5477031262524,21.602527086122,-21.602527086122));
#56415=CARTESIAN_POINT('Ctrl Pts',(10.5477031262524,21.602527086122,0.));
#56416=CARTESIAN_POINT('Ctrl Pts',(9.62553662153839,23.0838998256659,0.));
#56417=CARTESIAN_POINT('Ctrl Pts',(9.62553662153839,23.0838998256659,23.0838998256659));
#56418=CARTESIAN_POINT('Ctrl Pts',(9.62553662153839,0.,23.0838998256659));
#56419=CARTESIAN_POINT('Ctrl Pts',(9.62553662153839,-23.0838998256659,23.0838998256659));
#56420=CARTESIAN_POINT('Ctrl Pts',(9.62553662153839,-23.0838998256659,0.));
#56421=CARTESIAN_POINT('Ctrl Pts',(9.62553662153839,-23.0838998256659,-23.0838998256659));
#56422=CARTESIAN_POINT('Ctrl Pts',(9.62553662153839,0.,-23.0838998256659));
#56423=CARTESIAN_POINT('Ctrl Pts',(9.62553662153839,23.0838998256659,-23.0838998256659));
#56424=CARTESIAN_POINT('Ctrl Pts',(9.62553662153839,23.0838998256659,0.));
#56425=CARTESIAN_POINT('Ctrl Pts',(8.75359166551105,24.5886478127263,0.));
#56426=CARTESIAN_POINT('Ctrl Pts',(8.75359166551105,24.5886478127262,24.5886478127262));
#56427=CARTESIAN_POINT('Ctrl Pts',(8.75359166551105,0.,24.5886478127263));
#56428=CARTESIAN_POINT('Ctrl Pts',(8.75359166551105,-24.5886478127262,24.5886478127262));
#56429=CARTESIAN_POINT('Ctrl Pts',(8.75359166551105,-24.5886478127263,0.));
#56430=CARTESIAN_POINT('Ctrl Pts',(8.75359166551105,-24.5886478127262,-24.5886478127262));
#56431=CARTESIAN_POINT('Ctrl Pts',(8.75359166551105,0.,-24.5886478127263));
#56432=CARTESIAN_POINT('Ctrl Pts',(8.75359166551105,24.5886478127262,-24.5886478127262));
#56433=CARTESIAN_POINT('Ctrl Pts',(8.75359166551105,24.5886478127263,0.));
#56434=CARTESIAN_POINT('Ctrl Pts',(7.92870053877921,26.1164647205758,0.));
#56435=CARTESIAN_POINT('Ctrl Pts',(7.92870053877921,26.1164647205758,26.1164647205758));
#56436=CARTESIAN_POINT('Ctrl Pts',(7.92870053877921,0.,26.1164647205758));
#56437=CARTESIAN_POINT('Ctrl Pts',(7.92870053877921,-26.1164647205758,26.1164647205758));
#56438=CARTESIAN_POINT('Ctrl Pts',(7.92870053877921,-26.1164647205758,0.));
#56439=CARTESIAN_POINT('Ctrl Pts',(7.92870053877921,-26.1164647205758,-26.1164647205758));
#56440=CARTESIAN_POINT('Ctrl Pts',(7.92870053877921,0.,-26.1164647205758));
#56441=CARTESIAN_POINT('Ctrl Pts',(7.92870053877921,26.1164647205758,-26.1164647205758));
#56442=CARTESIAN_POINT('Ctrl Pts',(7.92870053877921,26.1164647205758,0.));
#56443=CARTESIAN_POINT('Ctrl Pts',(7.14689760675259,27.6690738550248,0.));
#56444=CARTESIAN_POINT('Ctrl Pts',(7.14689760675259,27.6690738550248,27.6690738550248));
#56445=CARTESIAN_POINT('Ctrl Pts',(7.1468976067526,0.,27.6690738550248));
#56446=CARTESIAN_POINT('Ctrl Pts',(7.1468976067526,-27.6690738550248,27.6690738550248));
#56447=CARTESIAN_POINT('Ctrl Pts',(7.1468976067526,-27.6690738550248,0.));
#56448=CARTESIAN_POINT('Ctrl Pts',(7.1468976067526,-27.6690738550248,-27.6690738550248));
#56449=CARTESIAN_POINT('Ctrl Pts',(7.1468976067526,0.,-27.6690738550248));
#56450=CARTESIAN_POINT('Ctrl Pts',(7.14689760675259,27.6690738550248,-27.6690738550248));
#56451=CARTESIAN_POINT('Ctrl Pts',(7.14689760675259,27.6690738550248,0.));
#56452=CARTESIAN_POINT('Ctrl Pts',(6.40416480933221,29.248955946805,0.));
#56453=CARTESIAN_POINT('Ctrl Pts',(6.40416480933221,29.248955946805,29.248955946805));
#56454=CARTESIAN_POINT('Ctrl Pts',(6.40416480933221,0.,29.248955946805));
#56455=CARTESIAN_POINT('Ctrl Pts',(6.40416480933221,-29.248955946805,29.248955946805));
#56456=CARTESIAN_POINT('Ctrl Pts',(6.40416480933221,-29.248955946805,0.));
#56457=CARTESIAN_POINT('Ctrl Pts',(6.40416480933221,-29.248955946805,-29.248955946805));
#56458=CARTESIAN_POINT('Ctrl Pts',(6.40416480933221,0.,-29.248955946805));
#56459=CARTESIAN_POINT('Ctrl Pts',(6.40416480933221,29.248955946805,-29.248955946805));
#56460=CARTESIAN_POINT('Ctrl Pts',(6.40416480933221,29.248955946805,0.));
#56461=CARTESIAN_POINT('Ctrl Pts',(5.69731071687183,30.8577859595634,0.));
#56462=CARTESIAN_POINT('Ctrl Pts',(5.69731071687183,30.8577859595634,30.8577859595634));
#56463=CARTESIAN_POINT('Ctrl Pts',(5.69731071687183,0.,30.8577859595634));
#56464=CARTESIAN_POINT('Ctrl Pts',(5.69731071687183,-30.8577859595634,30.8577859595634));
#56465=CARTESIAN_POINT('Ctrl Pts',(5.69731071687183,-30.8577859595634,0.));
#56466=CARTESIAN_POINT('Ctrl Pts',(5.69731071687183,-30.8577859595634,-30.8577859595634));
#56467=CARTESIAN_POINT('Ctrl Pts',(5.69731071687183,0.,-30.8577859595634));
#56468=CARTESIAN_POINT('Ctrl Pts',(5.69731071687183,30.8577859595634,-30.8577859595634));
#56469=CARTESIAN_POINT('Ctrl Pts',(5.69731071687183,30.8577859595634,0.));
#56470=CARTESIAN_POINT('Ctrl Pts',(5.02401496259691,32.4964011792533,0.));
#56471=CARTESIAN_POINT('Ctrl Pts',(5.02401496259691,32.4964011792533,32.4964011792533));
#56472=CARTESIAN_POINT('Ctrl Pts',(5.02401496259691,0.,32.4964011792533));
#56473=CARTESIAN_POINT('Ctrl Pts',(5.02401496259691,-32.4964011792533,32.4964011792533));
#56474=CARTESIAN_POINT('Ctrl Pts',(5.02401496259691,-32.4964011792533,0.));
#56475=CARTESIAN_POINT('Ctrl Pts',(5.02401496259691,-32.4964011792533,-32.4964011792533));
#56476=CARTESIAN_POINT('Ctrl Pts',(5.02401496259691,0.,-32.4964011792533));
#56477=CARTESIAN_POINT('Ctrl Pts',(5.02401496259691,32.4964011792533,-32.4964011792533));
#56478=CARTESIAN_POINT('Ctrl Pts',(5.02401496259691,32.4964011792533,0.));
#56479=CARTESIAN_POINT('Ctrl Pts',(4.38267277981043,34.1651137045816,0.));
#56480=CARTESIAN_POINT('Ctrl Pts',(4.38267277981043,34.1651137045815,34.1651137045815));
#56481=CARTESIAN_POINT('Ctrl Pts',(4.38267277981043,0.,34.1651137045816));
#56482=CARTESIAN_POINT('Ctrl Pts',(4.38267277981043,-34.1651137045815,34.1651137045815));
#56483=CARTESIAN_POINT('Ctrl Pts',(4.38267277981043,-34.1651137045816,0.));
#56484=CARTESIAN_POINT('Ctrl Pts',(4.38267277981043,-34.1651137045815,-34.1651137045815));
#56485=CARTESIAN_POINT('Ctrl Pts',(4.38267277981043,0.,-34.1651137045816));
#56486=CARTESIAN_POINT('Ctrl Pts',(4.38267277981043,34.1651137045815,-34.1651137045815));
#56487=CARTESIAN_POINT('Ctrl Pts',(4.38267277981043,34.1651137045816,0.));
#56488=CARTESIAN_POINT('Ctrl Pts',(3.89437496746067,35.5241326822989,0.));
#56489=CARTESIAN_POINT('Ctrl Pts',(3.89437496746067,35.5241326822989,35.5241326822989));
#56490=CARTESIAN_POINT('Ctrl Pts',(3.89437496746067,0.,35.5241326822989));
#56491=CARTESIAN_POINT('Ctrl Pts',(3.89437496746066,-35.5241326822989,35.5241326822989));
#56492=CARTESIAN_POINT('Ctrl Pts',(3.89437496746066,-35.5241326822989,0.));
#56493=CARTESIAN_POINT('Ctrl Pts',(3.89437496746066,-35.5241326822989,-35.5241326822989));
#56494=CARTESIAN_POINT('Ctrl Pts',(3.89437496746067,0.,-35.5241326822989));
#56495=CARTESIAN_POINT('Ctrl Pts',(3.89437496746067,35.5241326822989,-35.5241326822989));
#56496=CARTESIAN_POINT('Ctrl Pts',(3.89437496746067,35.5241326822989,0.));
#56497=CARTESIAN_POINT('Ctrl Pts',(3.5418673953418,36.5568488026925,0.));
#56498=CARTESIAN_POINT('Ctrl Pts',(3.5418673953418,36.5568488026925,36.5568488026925));
#56499=CARTESIAN_POINT('Ctrl Pts',(3.5418673953418,0.,36.5568488026925));
#56500=CARTESIAN_POINT('Ctrl Pts',(3.5418673953418,-36.5568488026925,36.5568488026925));
#56501=CARTESIAN_POINT('Ctrl Pts',(3.5418673953418,-36.5568488026925,0.));
#56502=CARTESIAN_POINT('Ctrl Pts',(3.5418673953418,-36.5568488026925,-36.5568488026925));
#56503=CARTESIAN_POINT('Ctrl Pts',(3.5418673953418,0.,-36.5568488026925));
#56504=CARTESIAN_POINT('Ctrl Pts',(3.5418673953418,36.5568488026925,-36.5568488026925));
#56505=CARTESIAN_POINT('Ctrl Pts',(3.5418673953418,36.5568488026925,0.));
#56506=CARTESIAN_POINT('Ctrl Pts',(3.31294245015623,37.2512891119684,0.));
#56507=CARTESIAN_POINT('Ctrl Pts',(3.31294245015623,37.2512891119684,37.2512891119684));
#56508=CARTESIAN_POINT('Ctrl Pts',(3.31294245015623,0.,37.2512891119684));
#56509=CARTESIAN_POINT('Ctrl Pts',(3.31294245015623,-37.2512891119684,37.2512891119684));
#56510=CARTESIAN_POINT('Ctrl Pts',(3.31294245015623,-37.2512891119684,0.));
#56511=CARTESIAN_POINT('Ctrl Pts',(3.31294245015623,-37.2512891119684,-37.2512891119684));
#56512=CARTESIAN_POINT('Ctrl Pts',(3.31294245015623,0.,-37.2512891119684));
#56513=CARTESIAN_POINT('Ctrl Pts',(3.31294245015623,37.2512891119684,-37.2512891119684));
#56514=CARTESIAN_POINT('Ctrl Pts',(3.31294245015623,37.2512891119684,0.));
#56515=CARTESIAN_POINT('Ctrl Pts',(3.2,37.6,0.));
#56516=CARTESIAN_POINT('Ctrl Pts',(3.2,37.6,37.6));
#56517=CARTESIAN_POINT('Ctrl Pts',(3.2,0.,37.6));
#56518=CARTESIAN_POINT('Ctrl Pts',(3.2,-37.6,37.6));
#56519=CARTESIAN_POINT('Ctrl Pts',(3.2,-37.6,0.));
#56520=CARTESIAN_POINT('Ctrl Pts',(3.2,-37.6,-37.6));
#56521=CARTESIAN_POINT('Ctrl Pts',(3.2,0.,-37.6));
#56522=CARTESIAN_POINT('Ctrl Pts',(3.2,37.6,-37.6));
#56523=CARTESIAN_POINT('Ctrl Pts',(3.2,37.6,0.));
#56524=CARTESIAN_POINT('',(27.,9.2,0.));
#56525=CARTESIAN_POINT('Ctrl Pts',(24.5,9.71413754081038,0.));
#56526=CARTESIAN_POINT('Ctrl Pts',(24.584270852469,9.69059102176396,0.));
#56527=CARTESIAN_POINT('Ctrl Pts',(24.8823684230922,9.60913381736612,0.));
#56528=CARTESIAN_POINT('Ctrl Pts',(25.3906552690265,9.48132788945834,0.));
#56529=CARTESIAN_POINT('Ctrl Pts',(25.892339495915,9.37377670323605,0.));
#56530=CARTESIAN_POINT('Ctrl Pts',(26.3874085880356,9.28597940593777,0.));
#56531=CARTESIAN_POINT('Ctrl Pts',(26.796570998452,9.22636560737002,0.));
#56532=CARTESIAN_POINT('Ctrl Pts',(27.,9.2,0.));
#56533=CARTESIAN_POINT('',(27.,-9.2,-1.12667505521557E-15));
#56534=CARTESIAN_POINT('Origin',(27.,0.,0.));
#56535=CARTESIAN_POINT('Origin',(27.,0.,0.));
#56536=CARTESIAN_POINT('',(3.2,37.5892271801377,-0.899999999999994));
#56537=CARTESIAN_POINT('Origin',(3.2,0.,0.));
#56538=CARTESIAN_POINT('',(24.5,5.24229587453786,-8.17819063886291));
#56539=CARTESIAN_POINT('Ctrl Pts',(3.2,37.5892271801377,-0.9));
#56540=CARTESIAN_POINT('Ctrl Pts',(3.45174020122667,36.8117541621245,-0.9));
#56541=CARTESIAN_POINT('Ctrl Pts',(3.71840125351367,36.0251069070192,-0.899999999999995));
#56542=CARTESIAN_POINT('Ctrl Pts',(4.,35.2340925362767,-0.899999999999995));
#56543=CARTESIAN_POINT('Ctrl Pts',(4.62816481945855,33.4695697690894,-0.900000000000002));
#56544=CARTESIAN_POINT('Ctrl Pts',(5.32582968819375,31.7073778438848,-0.839717528293596));
#56545=CARTESIAN_POINT('Ctrl Pts',(6.03866110767478,30.0825526385231,-0.844879409428011));
#56546=CARTESIAN_POINT('Ctrl Pts',(6.32798219793006,29.4230752543307,-0.846974492552523));
#56547=CARTESIAN_POINT('Ctrl Pts',(6.61604117565574,28.793782414028,-0.861009606870751));
#56548=CARTESIAN_POINT('Ctrl Pts',(6.89476148100328,28.2061545880624,-0.893825964111232));
#56549=CARTESIAN_POINT('Ctrl Pts',(7.65522892458988,26.6028561486637,-0.983362932963847));
#56550=CARTESIAN_POINT('Ctrl Pts',(8.35226708789681,25.307434370521,-1.09931216348024));
#56551=CARTESIAN_POINT('Ctrl Pts',(8.78926323543883,24.5226424560649,-1.19512255048227));
#56552=CARTESIAN_POINT('Ctrl Pts',(8.9903195843563,24.1615697146506,-1.23920368645418));
#56553=CARTESIAN_POINT('Ctrl Pts',(9.18275522864328,23.8242551291094,-1.28645191173913));
#56554=CARTESIAN_POINT('Ctrl Pts',(9.37496047156673,23.4940308964114,-1.34002181064069));
#56555=CARTESIAN_POINT('Ctrl Pts',(9.48075234026397,23.312271865623,-1.36950726912516));
#56556=CARTESIAN_POINT('Ctrl Pts',(9.58626091274252,23.1330836509346,-1.40088640835537));
#56557=CARTESIAN_POINT('Ctrl Pts',(9.69257910363365,22.9544806736799,-1.43495784272423));
#56558=CARTESIAN_POINT('Ctrl Pts',(10.0319880480858,22.3843106258459,-1.54372708981334));
#56559=CARTESIAN_POINT('Ctrl Pts',(10.3788056757338,21.8199482988106,-1.68100872063375));
#56560=CARTESIAN_POINT('Ctrl Pts',(10.7756849097841,21.1980699537259,-1.85708105784221));
#56561=CARTESIAN_POINT('Ctrl Pts',(10.8890930417026,21.0203683877436,-1.90739367974876));
#56562=CARTESIAN_POINT('Ctrl Pts',(11.0576203534459,20.7579535709124,-1.98378827882632));
#56563=CARTESIAN_POINT('Ctrl Pts',(11.2725125504481,20.4310649639431,-2.08497651593983));
#56564=CARTESIAN_POINT('Ctrl Pts',(11.5968279601822,19.9377245170328,-2.23768985331333));
#56565=CARTESIAN_POINT('Ctrl Pts',(12.025567884829,19.2993337801102,-2.44965947375353));
#56566=CARTESIAN_POINT('Ctrl Pts',(12.532035905153,18.5840189796223,-2.68594697261969));
#56567=CARTESIAN_POINT('Ctrl Pts',(13.0988763174395,17.7834366720487,-2.95040059634461));
#56568=CARTESIAN_POINT('Ctrl Pts',(13.7495416909273,16.8976545731049,-3.30146477931067));
#56569=CARTESIAN_POINT('Ctrl Pts',(14.4398764933743,16.0059407465834,-3.67134635070127));
#56570=CARTESIAN_POINT('Ctrl Pts',(14.7901814029647,15.553447651533,-3.85903981475072));
#56571=CARTESIAN_POINT('Ctrl Pts',(15.1459546146389,15.1068649503278,-4.0457097304312));
#56572=CARTESIAN_POINT('Ctrl Pts',(15.4570717747561,14.7276262420568,-4.19832359076494));
#56573=CARTESIAN_POINT('Ctrl Pts',(15.7998231422506,14.3098267680006,-4.36645513744121));
#56574=CARTESIAN_POINT('Ctrl Pts',(16.0676294526253,13.990318693849,-4.50331995895759));
#56575=CARTESIAN_POINT('Ctrl Pts',(16.3615308021931,13.6447281514167,-4.65432808429673));
#56576=CARTESIAN_POINT('Ctrl Pts',(17.0296616056386,12.859091450129,-4.99761735553682));
#56577=CARTESIAN_POINT('Ctrl Pts',(17.7084691891668,12.0886798104406,-5.35674638147456));
#56578=CARTESIAN_POINT('Ctrl Pts',(18.4207032016838,11.3350011751768,-5.68212942088499));
#56579=CARTESIAN_POINT('Ctrl Pts',(18.8298642043985,10.902031251374,-5.86905401074141));
#56580=CARTESIAN_POINT('Ctrl Pts',(19.2113759274554,10.5047768811947,-6.04970003189267));
#56581=CARTESIAN_POINT('Ctrl Pts',(19.5701113609878,10.1352032844547,-6.21809496346388));
#56582=CARTESIAN_POINT('Ctrl Pts',(20.1215476022469,9.56710697724541,-6.47694608167746));
#56583=CARTESIAN_POINT('Ctrl Pts',(20.6514912601264,9.02382054581082,-6.73117610025783));
#56584=CARTESIAN_POINT('Ctrl Pts',(21.3979544325339,8.30110396122067,-7.03003130093698));
#56585=CARTESIAN_POINT('Ctrl Pts',(21.8107631281408,7.90142759190171,-7.19530405668434));
#56586=CARTESIAN_POINT('Ctrl Pts',(22.3076315954255,7.42611128017324,-7.38765428460632));
#56587=CARTESIAN_POINT('Ctrl Pts',(22.8472772293734,6.90153052972702,-7.58806809630901));
#56588=CARTESIAN_POINT('Ctrl Pts',(23.3953136567666,6.36879322533974,-7.79159808424252));
#56589=CARTESIAN_POINT('Ctrl Pts',(23.9608264582666,5.8087958334843,-7.99400612701712));
#56590=CARTESIAN_POINT('Ctrl Pts',(24.5,5.24229587453786,-8.17819063886291));
#56591=CARTESIAN_POINT('',(24.5,7.16983932323689,-6.55422552562448));
#56592=CARTESIAN_POINT('Ctrl Pts',(24.5,5.24229587453786,-8.17819063886291));
#56593=CARTESIAN_POINT('Ctrl Pts',(24.5,5.64521806942229,-7.91991378359311));
#56594=CARTESIAN_POINT('Ctrl Pts',(24.5,6.02903768297008,-7.63187011183746));
#56595=CARTESIAN_POINT('Ctrl Pts',(24.5,6.66464379880506,-7.07668969209044));
#56596=CARTESIAN_POINT('Ctrl Pts',(24.5,6.92481388700865,-6.82226528119806));
#56597=CARTESIAN_POINT('Ctrl Pts',(24.5,7.16983932323689,-6.55422552562448));
#56598=CARTESIAN_POINT('Ctrl Pts',(24.5,7.16983932323689,-6.55422552562448));
#56599=CARTESIAN_POINT('Ctrl Pts',(23.8274939345993,7.72087585355875,-6.22993425436329));
#56600=CARTESIAN_POINT('Ctrl Pts',(23.3366347314239,8.10243836675503,-5.9971074697364));
#56601=CARTESIAN_POINT('Ctrl Pts',(22.5855494187791,8.69228987173019,-5.63439342300611));
#56602=CARTESIAN_POINT('Ctrl Pts',(22.2454144275548,8.95940884355763,-5.4701354658546));
#56603=CARTESIAN_POINT('Ctrl Pts',(21.8382660751901,9.285050095425,-5.26284147008233));
#56604=CARTESIAN_POINT('Ctrl Pts',(21.3802156960109,9.65774830624375,-5.02425880299215));
#56605=CARTESIAN_POINT('Ctrl Pts',(20.7694693299338,10.1546894468861,-4.70614205523307));
#56606=CARTESIAN_POINT('Ctrl Pts',(20.1629003036551,10.6565278673439,-4.38627069785178));
#56607=CARTESIAN_POINT('Ctrl Pts',(19.5574857571565,11.1735047521273,-4.09023617084508));
#56608=CARTESIAN_POINT('Ctrl Pts',(18.6418529423121,11.9553838843044,-3.64251166732608));
#56609=CARTESIAN_POINT('Ctrl Pts',(17.773481333357,12.7723018260926,-3.16504296577866));
#56610=CARTESIAN_POINT('Ctrl Pts',(16.9621253129276,13.5883953552262,-2.76110771822243));
#56611=CARTESIAN_POINT('Ctrl Pts',(16.8133360681893,13.7380533805297,-2.68703268963603));
#56612=CARTESIAN_POINT('Ctrl Pts',(16.6656205375718,13.8886489787092,-2.61462956901353));
#56613=CARTESIAN_POINT('Ctrl Pts',(16.5183901926363,14.0408164096359,-2.54382268324666));
#56614=CARTESIAN_POINT('Ctrl Pts',(15.7264522885453,14.8593104257425,-2.16295923601354));
#56615=CARTESIAN_POINT('Ctrl Pts',(14.9462259716364,15.7452570124731,-1.74040949812692));
#56616=CARTESIAN_POINT('Ctrl Pts',(14.2963150411565,16.5251374105151,-1.42162688464704));
#56617=CARTESIAN_POINT('Ctrl Pts',(13.9908350931921,16.8917073699346,-1.27178835814949));
#56618=CARTESIAN_POINT('Ctrl Pts',(13.7077063565862,17.2419142372062,-1.13921261589477));
#56619=CARTESIAN_POINT('Ctrl Pts',(13.4460198946299,17.5732908880439,-1.02322593212869));
#56620=CARTESIAN_POINT('Ctrl Pts',(12.8297897879206,18.3536303346477,-0.750095690771559));
#56621=CARTESIAN_POINT('Ctrl Pts',(12.341051952675,19.0193845631393,-0.520653486972896));
#56622=CARTESIAN_POINT('Ctrl Pts',(11.9631039144853,19.5480150790474,-0.35462224598778));
#56623=CARTESIAN_POINT('Ctrl Pts',(11.6627866324515,19.9680645665328,-0.222693922548958));
#56624=CARTESIAN_POINT('Ctrl Pts',(11.3909151560383,20.3600418064951,-0.108420555322461));
#56625=CARTESIAN_POINT('Ctrl Pts',(11.1111871729018,20.775057671175,1.50053580671994E-15));
#56626=CARTESIAN_POINT('Ctrl Pts',(2.09999999999999,9.70239382419368,0.9));
#56627=CARTESIAN_POINT('Ctrl Pts',(2.73333333333333,9.70239382419368,0.9));
#56628=CARTESIAN_POINT('Ctrl Pts',(3.36632387111522,9.70238311374191,0.899943572704684));
#56629=CARTESIAN_POINT('Ctrl Pts',(4.12418390810446,9.70237979485746,0.899926556305573));
#56630=CARTESIAN_POINT('Ctrl Pts',(4.36793405804848,9.70227889326302,0.901142755072256));
#56631=CARTESIAN_POINT('Ctrl Pts',(4.86516733785842,9.70182686384601,0.906703885275862));
#56632=CARTESIAN_POINT('Ctrl Pts',(5.74558933798915,9.70077369524553,0.919837119111666));
#56633=CARTESIAN_POINT('Ctrl Pts',(6.51837592843883,9.70075915441346,0.920043366739036));
#56634=CARTESIAN_POINT('Ctrl Pts',(7.1031128831408,9.70255678431008,0.896330940156011));
#56635=CARTESIAN_POINT('Ctrl Pts',(7.23026824315571,9.70301993681095,0.891007254471877));
#56636=CARTESIAN_POINT('Ctrl Pts',(7.42494888780729,9.70386111674548,0.882248192098819));
#56637=CARTESIAN_POINT('Ctrl Pts',(7.61951912013724,9.70483286951889,0.872784906947758));
#56638=CARTESIAN_POINT('Ctrl Pts',(8.01076648546345,9.70700730924683,0.852173583936991));
#56639=CARTESIAN_POINT('Ctrl Pts',(8.6008368585707,9.7109991524828,0.814319361374828));
#56640=CARTESIAN_POINT('Ctrl Pts',(9.25154787508086,9.71589427768064,0.755208645277658));
#56641=CARTESIAN_POINT('Ctrl Pts',(9.76267229657535,9.71954704831515,0.694519587021701));
#56642=CARTESIAN_POINT('Ctrl Pts',(10.014171082006,9.72118810845726,0.65910761044294));
#56643=CARTESIAN_POINT('Ctrl Pts',(10.7177517881878,9.72539449907129,0.550905934553037));
#56644=CARTESIAN_POINT('Ctrl Pts',(11.8208631668899,9.7387414708566,0.30695723782105));
#56645=CARTESIAN_POINT('Ctrl Pts',(12.8080214119101,9.74360244998835,0.00601043568995343));
#56646=CARTESIAN_POINT('Ctrl Pts',(13.5604126906717,9.73617681748438,-0.231382581987876));
#56647=CARTESIAN_POINT('Ctrl Pts',(14.1415324087999,9.72798482552665,-0.434588673886165));
#56648=CARTESIAN_POINT('Ctrl Pts',(15.2007205223741,9.70191685856208,-0.866738392578812));
#56649=CARTESIAN_POINT('Ctrl Pts',(15.9284934234743,9.66540770021948,-1.21113245671502));
#56650=CARTESIAN_POINT('Ctrl Pts',(16.6747552776732,9.60865895503553,-1.56555224791166));
#56651=CARTESIAN_POINT('Ctrl Pts',(17.2497622997617,9.55601631928308,-1.85742036071714));
#56652=CARTESIAN_POINT('Ctrl Pts',(18.2984408124205,9.42723341754466,-2.44688146345142));
#56653=CARTESIAN_POINT('Ctrl Pts',(19.023654255104,9.29844614565911,-2.89446970327295));
#56654=CARTESIAN_POINT('Ctrl Pts',(19.7681836146925,9.13779726718118,-3.34781162099393));
#56655=CARTESIAN_POINT('Ctrl Pts',(20.3331355916067,8.99879342938229,-3.70764381764044));
#56656=CARTESIAN_POINT('Ctrl Pts',(21.3722795878879,8.68312647686188,-4.41282175870863));
#56657=CARTESIAN_POINT('Ctrl Pts',(22.0962322041254,8.39994687509579,-4.92488812724573));
#56658=CARTESIAN_POINT('Ctrl Pts',(23.2302270680055,7.90257741264269,-5.69145757370445));
#56659=CARTESIAN_POINT('Ctrl Pts',(23.8854423668127,7.55670872152269,-6.13564425905366));
#56660=CARTESIAN_POINT('Ctrl Pts',(24.5000000001022,7.16983932310749,-6.55422552562591));
#56661=CARTESIAN_POINT('Ctrl Pts',(2.09999999999999,13.886302003518,0.9));
#56662=CARTESIAN_POINT('Ctrl Pts',(2.73333333333333,13.886302003518,0.9));
#56663=CARTESIAN_POINT('Ctrl Pts',(3.36613013456572,13.886293466186,0.899934636656705));
#56664=CARTESIAN_POINT('Ctrl Pts',(4.12377198935332,13.8862908337435,0.899915275189073));
#56665=CARTESIAN_POINT('Ctrl Pts',(4.36466956133672,13.8861969875265,0.901644022806547));
#56666=CARTESIAN_POINT('Ctrl Pts',(4.86001353404206,13.8857766744056,0.909581065394921));
#56667=CARTESIAN_POINT('Ctrl Pts',(5.74114344094781,13.8847964321218,0.928387766932829));
#56668=CARTESIAN_POINT('Ctrl Pts',(6.52371165318003,13.8847857317307,0.928826747414305));
#56669=CARTESIAN_POINT('Ctrl Pts',(7.12008868672732,13.8864582425445,0.894425264736249));
#56670=CARTESIAN_POINT('Ctrl Pts',(7.2473920845663,13.886908806475,0.886799179992507));
#56671=CARTESIAN_POINT('Ctrl Pts',(7.44367696450914,13.8877691576202,0.874193604263346));
#56672=CARTESIAN_POINT('Ctrl Pts',(7.63959093335125,13.8887879198323,0.860585277112663));
#56673=CARTESIAN_POINT('Ctrl Pts',(8.03420776743963,13.891091359666,0.830913205754772));
#56674=CARTESIAN_POINT('Ctrl Pts',(8.63054063110045,13.8953340247099,0.776366915874588));
#56675=CARTESIAN_POINT('Ctrl Pts',(9.29110414788195,13.9000524777747,0.690945060637293));
#56676=CARTESIAN_POINT('Ctrl Pts',(9.81209171470009,13.9029382846741,0.602989957084009));
#56677=CARTESIAN_POINT('Ctrl Pts',(10.0692653859326,13.9039233252519,0.551564607071378));
#56678=CARTESIAN_POINT('Ctrl Pts',(10.7901161263785,13.905801040616,0.394264167844574));
#56679=CARTESIAN_POINT('Ctrl Pts',(11.9164140743865,13.9153944782979,0.0402610058985021));
#56680=CARTESIAN_POINT('Ctrl Pts',(12.9133300122381,13.9101438826876,-0.392622143318933));
#56681=CARTESIAN_POINT('Ctrl Pts',(13.6697345269123,13.8898038073169,-0.732507745058096));
#56682=CARTESIAN_POINT('Ctrl Pts',(14.2631482815798,13.8697611392688,-1.0268202159191));
#56683=CARTESIAN_POINT('Ctrl Pts',(15.3329170876201,13.8143188664754,-1.64805789896314));
#56684=CARTESIAN_POINT('Ctrl Pts',(16.065400822286,13.7476864604472,-2.1401844399863));
#56685=CARTESIAN_POINT('Ctrl Pts',(16.8131024396104,13.6516057483624,-2.64427530685194));
#56686=CARTESIAN_POINT('Ctrl Pts',(17.3939205030447,13.5638317918362,-3.06247796039152));
#56687=CARTESIAN_POINT('Ctrl Pts',(18.4451570754854,13.3544577672646,-3.90129822129329));
#56688=CARTESIAN_POINT('Ctrl Pts',(19.1720430750714,13.1515971699246,-4.53544369462377));
#56689=CARTESIAN_POINT('Ctrl Pts',(19.9173987143267,12.902625551066,-5.17597857280555));
#56690=CARTESIAN_POINT('Ctrl Pts',(20.4826350906704,12.6889939496253,-5.68486006256131));
#56691=CARTESIAN_POINT('Ctrl Pts',(21.5194164976709,12.2087215604998,-6.67751869749508));
#56692=CARTESIAN_POINT('Ctrl Pts',(22.2433236988674,11.7831123238236,-7.39621420284916));
#56693=CARTESIAN_POINT('Ctrl Pts',(23.3780713364062,11.0396851260099,-8.46963766904746));
#56694=CARTESIAN_POINT('Ctrl Pts',(24.0312127056184,10.5284370227301,-9.08844396340443));
#56695=CARTESIAN_POINT('Ctrl Pts',(24.6419825553303,9.96056935923752,-9.66798043909671));
#56696=CARTESIAN_POINT('Ctrl Pts',(2.09999999999999,23.6487544219413,0.9));
#56697=CARTESIAN_POINT('Ctrl Pts',(2.73333333333333,23.6487544219413,0.9));
#56698=CARTESIAN_POINT('Ctrl Pts',(3.36565166989018,23.648723186002,0.899810674604605));
#56699=CARTESIAN_POINT('Ctrl Pts',(4.1227770961911,23.6487135356683,0.899754412481333));
#56700=CARTESIAN_POINT('Ctrl Pts',(4.35701428556174,23.6486339129901,0.902631341193944));
#56701=CARTESIAN_POINT('Ctrl Pts',(4.84795832867355,23.6482823455618,0.916015675715051));
#56702=CARTESIAN_POINT('Ctrl Pts',(5.73069615138054,23.6474648422221,0.948050758092538));
#56703=CARTESIAN_POINT('Ctrl Pts',(6.53614700405502,23.6474243933554,0.949253331942218));
#56704=CARTESIAN_POINT('Ctrl Pts',(7.15941198676745,23.6487878326115,0.888431899181333));
#56705=CARTESIAN_POINT('Ctrl Pts',(7.28705556652675,23.6492079046684,0.875410302124557));
#56706=CARTESIAN_POINT('Ctrl Pts',(7.48703947127753,23.6501100122595,0.853609697064992));
#56707=CARTESIAN_POINT('Ctrl Pts',(7.68604134768081,23.6512342606514,0.830120478181656));
#56708=CARTESIAN_POINT('Ctrl Pts',(8.08839242481482,23.6538318226179,0.778768089003677));
#56709=CARTESIAN_POINT('Ctrl Pts',(8.69896725403256,23.6586132337531,0.683967884128669));
#56710=CARTESIAN_POINT('Ctrl Pts',(9.38146799592133,23.6628388218879,0.534448529854445));
#56711=CARTESIAN_POINT('Ctrl Pts',(9.92347326694303,23.6638129580854,0.379381577922531));
#56712=CARTESIAN_POINT('Ctrl Pts',(10.1922138317613,23.663170473224,0.288268137281189));
#56713=CARTESIAN_POINT('Ctrl Pts',(10.9469984854868,23.6592100918921,0.00858085944299974));
#56714=CARTESIAN_POINT('Ctrl Pts',(12.1071835656316,23.6588244502173,-0.615249067553259));
#56715=CARTESIAN_POINT('Ctrl Pts',(13.10934181009,23.6284698279663,-1.35870373313894));
#56716=CARTESIAN_POINT('Ctrl Pts',(13.8683634030329,23.5768907059628,-1.93925931749388));
#56717=CARTESIAN_POINT('Ctrl Pts',(14.4658081522521,23.5282487607608,-2.44691660663979));
#56718=CARTESIAN_POINT('Ctrl Pts',(15.5292065922307,23.4040225569915,-3.50091787875384));
#56719=CARTESIAN_POINT('Ctrl Pts',(16.25612925985,23.2671320804502,-4.33240603899768));
#56720=CARTESIAN_POINT('Ctrl Pts',(17.0018288855248,23.0785614632775,-5.18472180987648));
#56721=CARTESIAN_POINT('Ctrl Pts',(17.5709926777516,22.9116014373373,-5.88434164318249));
#56722=CARTESIAN_POINT('Ctrl Pts',(18.6067980794747,22.520519768836,-7.28568570527198));
#56723=CARTESIAN_POINT('Ctrl Pts',(19.3243460106793,22.1491525108876,-8.34596662426811));
#56724=CARTESIAN_POINT('Ctrl Pts',(20.0666634439746,21.6959815979795,-9.42157847934581));
#56725=CARTESIAN_POINT('Ctrl Pts',(20.6167925376506,21.3177487953732,-10.2604211543252));
#56726=CARTESIAN_POINT('Ctrl Pts',(21.6393809830421,20.4677589075133,-11.9080648199959));
#56727=CARTESIAN_POINT('Ctrl Pts',(22.3554885642927,19.7185230095471,-13.1029251946305));
#56728=CARTESIAN_POINT('Ctrl Pts',(23.4867409067233,18.408630119116,-14.8934828716927));
#56729=CARTESIAN_POINT('Ctrl Pts',(24.1253373265787,17.5278847743971,-15.9063459622623));
#56730=CARTESIAN_POINT('Ctrl Pts',(24.7277571265287,16.5516187964772,-16.8576639625222));
#56731=CARTESIAN_POINT('Ctrl Pts',(2.09999999999999,33.4112068403646,0.9));
#56732=CARTESIAN_POINT('Ctrl Pts',(2.73333333333333,33.4112068403646,0.9));
#56733=CARTESIAN_POINT('Ctrl Pts',(3.36511452663434,33.4111761653147,0.899840745554594));
#56734=CARTESIAN_POINT('Ctrl Pts',(4.12170983818995,33.4111667671358,0.899796306780195));
#56735=CARTESIAN_POINT('Ctrl Pts',(4.34927019961831,33.4111030790715,0.903743099070193));
#56736=CARTESIAN_POINT('Ctrl Pts',(4.83587450315472,33.4108253785101,0.92242175897404));
#56737=CARTESIAN_POINT('Ctrl Pts',(5.72001145403567,33.4101755509066,0.967787576946441));
#56738=CARTESIAN_POINT('Ctrl Pts',(6.54876301828212,33.4101411791828,0.97075247449325));
#56739=CARTESIAN_POINT('Ctrl Pts',(7.19754212980654,33.4112032548265,0.880480590233061));
#56740=CARTESIAN_POINT('Ctrl Pts',(7.32550057368378,33.4115919397608,0.862020988728711));
#56741=CARTESIAN_POINT('Ctrl Pts',(7.52895904796954,33.4125344491362,0.830573953588618));
#56742=CARTESIAN_POINT('Ctrl Pts',(7.73081337870169,33.4137623486153,0.796794277431493));
#56743=CARTESIAN_POINT('Ctrl Pts',(8.14024610125225,33.416644671293,0.722660084039429));
#56744=CARTESIAN_POINT('Ctrl Pts',(8.76331513085336,33.4219612775907,0.585414526276326));
#56745=CARTESIAN_POINT('Ctrl Pts',(9.46278822378255,33.4256153655972,0.367459274710017));
#56746=CARTESIAN_POINT('Ctrl Pts',(10.0176548667882,33.4245339217562,0.141184776125187));
#56747=CARTESIAN_POINT('Ctrl Pts',(10.2919127083958,33.4221691705248,0.00852806418557635));
#56748=CARTESIAN_POINT('Ctrl Pts',(11.0596838975171,33.4121382406894,-0.39741540036137));
#56749=CARTESIAN_POINT('Ctrl Pts',(12.2113609303221,33.4016448516588,-1.27944658677757));
#56750=CARTESIAN_POINT('Ctrl Pts',(13.2034544750666,33.3476280317028,-2.31751121998455));
#56751=CARTESIAN_POINT('Ctrl Pts',(13.958790347696,33.2656790468827,-3.13274228974461));
#56752=CARTESIAN_POINT('Ctrl Pts',(14.542824409456,33.1913245084766,-3.83240360300729));
#56753=CARTESIAN_POINT('Ctrl Pts',(15.5915804267801,33.0041588224546,-5.29349765081425));
#56754=CARTESIAN_POINT('Ctrl Pts',(16.3123204181258,32.8020629110146,-6.45249308889002));
#56755=CARTESIAN_POINT('Ctrl Pts',(17.0563550542797,32.5245018229527,-7.64998966563405));
#56756=CARTESIAN_POINT('Ctrl Pts',(17.6162778419526,32.2852973888993,-8.61371409555214));
#56757=CARTESIAN_POINT('Ctrl Pts',(18.6451709005287,31.7226316969721,-10.5658949269178));
#56758=CARTESIAN_POINT('Ctrl Pts',(19.3594051248222,31.1901454406191,-12.0481304710539));
#56759=CARTESIAN_POINT('Ctrl Pts',(20.1008987914504,30.5386549627683,-13.5595949879592));
#56760=CARTESIAN_POINT('Ctrl Pts',(20.6466183193975,30.003280804915,-14.7231785594183));
#56761=CARTESIAN_POINT('Ctrl Pts',(21.6663807536096,28.7938945751524,-17.0275349953218));
#56762=CARTESIAN_POINT('Ctrl Pts',(22.3810364687107,27.7280363584589,-18.7018955338072));
#56763=CARTESIAN_POINT('Ctrl Pts',(23.5117483399784,25.8614793339912,-21.216829058667));
#56764=CARTESIAN_POINT('Ctrl Pts',(24.1480627906507,24.61701655753,-22.6285410064029));
#56765=CARTESIAN_POINT('Ctrl Pts',(24.7493903499091,23.2364939785392,-23.9577803684282));
#56766=CARTESIAN_POINT('Ctrl Pts',(2.09999999999999,38.9897510794637,0.9));
#56767=CARTESIAN_POINT('Ctrl Pts',(2.73333333333333,38.9897510794637,0.9));
#56768=CARTESIAN_POINT('Ctrl Pts',(3.36478879685081,38.9897220570697,0.89985896409509));
#56769=CARTESIAN_POINT('Ctrl Pts',(4.12107778498996,38.989713228803,0.899821396098744));
#56770=CARTESIAN_POINT('Ctrl Pts',(4.34481509744132,38.9896587133212,0.904351569922351));
#56771=CARTESIAN_POINT('Ctrl Pts',(4.82897515227901,38.989423652051,0.925991788001339));
#56772=CARTESIAN_POINT('Ctrl Pts',(5.71380230618561,38.9888696861857,0.979014362623941));
#56773=CARTESIAN_POINT('Ctrl Pts',(6.55610955603432,38.9888414597256,0.98318304814543));
#56774=CARTESIAN_POINT('Ctrl Pts',(7.21873857123617,38.9897305837832,0.875215691307443));
#56775=CARTESIAN_POINT('Ctrl Pts',(7.34686387089368,38.9901009601951,0.853636790127038));
#56776=CARTESIAN_POINT('Ctrl Pts',(7.55218952294518,38.991065815581,0.816553666708369));
#56777=CARTESIAN_POINT('Ctrl Pts',(7.75555264488831,38.9923519711669,0.776785625693149));
#56778=CARTESIAN_POINT('Ctrl Pts',(8.16869603838144,38.9953940636619,0.689360805961949));
#56779=CARTESIAN_POINT('Ctrl Pts',(8.79805341970188,39.0010104332016,0.527343393080334));
#56780=CARTESIAN_POINT('Ctrl Pts',(9.50502666554615,39.0043196140019,0.269763699750302));
#56781=CARTESIAN_POINT('Ctrl Pts',(10.064431266213,39.0020570255402,0.00315136578276065));
#56782=CARTESIAN_POINT('Ctrl Pts',(10.3401531790778,38.9987170953899,-0.152616667959919));
#56783=CARTESIAN_POINT('Ctrl Pts',(11.1103010543903,38.9852807309237,-0.627999100260067));
#56784=CARTESIAN_POINT('Ctrl Pts',(12.254576959855,38.9694318216162,-1.64974102780262));
#56785=CARTESIAN_POINT('Ctrl Pts',(13.2428711731431,38.9024766882624,-2.85423024818584));
#56786=CARTESIAN_POINT('Ctrl Pts',(13.9964017017256,38.8035591455185,-3.80267703087181));
#56787=CARTESIAN_POINT('Ctrl Pts',(14.5753786143845,38.7150140796801,-4.61020769734798));
#56788=CARTESIAN_POINT('Ctrl Pts',(15.6192592403265,38.492440052229,-6.30454904922076));
#56789=CARTESIAN_POINT('Ctrl Pts',(16.3373913183118,38.2535226204795,-7.65097529021429));
#56790=CARTESIAN_POINT('Ctrl Pts',(17.0806205854546,37.9256324686629,-9.04571732323448));
#56791=CARTESIAN_POINT('Ctrl Pts',(17.6370003403016,37.6452040748109,-10.1616972682833));
#56792=CARTESIAN_POINT('Ctrl Pts',(18.6627915222875,36.984538240599,-12.4306082839159));
#56793=CARTESIAN_POINT('Ctrl Pts',(19.3754523008299,36.3603136908351,-14.1544547728556));
#56794=CARTESIAN_POINT('Ctrl Pts',(20.1166123028179,35.5959813536198,-15.9150758011866));
#56795=CARTESIAN_POINT('Ctrl Pts',(20.6599948765211,34.970628879379,-17.26545899592));
#56796=CARTESIAN_POINT('Ctrl Pts',(21.6777842655078,33.5558510677647,-19.9461245033443));
#56797=CARTESIAN_POINT('Ctrl Pts',(22.391798977594,32.3094239354671,-21.8948863198921));
#56798=CARTESIAN_POINT('Ctrl Pts',(23.5225016210748,30.1253828617895,-24.8241019273224));
#56799=CARTESIAN_POINT('Ctrl Pts',(24.157514841919,28.6731789929379,-26.4644737024698));
#56800=CARTESIAN_POINT('Ctrl Pts',(24.7577717974218,27.0616688848421,-28.0099816319188));
#56801=CARTESIAN_POINT('',(24.5,19.2888993183199,-18.8928124716178));
#56802=CARTESIAN_POINT('Ctrl Pts',(24.5,19.2888993183199,-18.8928124716178));
#56803=CARTESIAN_POINT('Ctrl Pts',(24.5,18.4146674682996,-18.0152760071265));
#56804=CARTESIAN_POINT('Ctrl Pts',(24.5,17.5558967018297,-17.1519793443978));
#56805=CARTESIAN_POINT('Ctrl Pts',(24.5,14.0106747121728,-13.5812560497461));
#56806=CARTESIAN_POINT('Ctrl Pts',(24.5,10.2531955099118,-9.78418534540856));
#56807=CARTESIAN_POINT('Ctrl Pts',(24.5,7.16983932323689,-6.55422552562448));
#56808=CARTESIAN_POINT('',(10.2670750393577,34.1526563890204,0.));
#56809=CARTESIAN_POINT('Ctrl Pts',(10.2670750393577,34.1526563890204,-4.68375338513738E-16));
#56810=CARTESIAN_POINT('Ctrl Pts',(11.2293198185888,33.2721453537472,-0.465431410556517));
#56811=CARTESIAN_POINT('Ctrl Pts',(12.092802582344,32.5668339115407,-1.14700595996091));
#56812=CARTESIAN_POINT('Ctrl Pts',(14.3080979519049,30.8500805090056,-3.2126602051371));
#56813=CARTESIAN_POINT('Ctrl Pts',(14.8952017874601,30.4291106260349,-3.86523333611874));
#56814=CARTESIAN_POINT('Ctrl Pts',(17.0803363586062,28.6861024817812,-6.7160879710462));
#56815=CARTESIAN_POINT('Ctrl Pts',(17.6922811489506,28.1624534567924,-7.58672157878782));
#56816=CARTESIAN_POINT('Ctrl Pts',(19.0755427322033,26.8718943495686,-9.71692181817951));
#56817=CARTESIAN_POINT('Ctrl Pts',(20.2687424742408,25.6862391985472,-11.6130226450378));
#56818=CARTESIAN_POINT('Ctrl Pts',(22.3267279388309,22.9384152527353,-15.2120800399172));
#56819=CARTESIAN_POINT('Ctrl Pts',(23.4192562717209,21.3312428140497,-17.071137473725));
#56820=CARTESIAN_POINT('Ctrl Pts',(24.5,19.2888993183199,-18.8928124716178));
#56821=CARTESIAN_POINT('Ctrl Pts',(6.,38.9878978038234,0.971506478939046));
#56822=CARTESIAN_POINT('Ctrl Pts',(7.51604047332547,36.8303135352266,0.968297921939491));
#56823=CARTESIAN_POINT('Ctrl Pts',(9.08449301626627,35.2778821774931,0.481732853248133));
#56824=CARTESIAN_POINT('Ctrl Pts',(9.8624969752411,34.5273296915935,0.184503206613648));
#56825=CARTESIAN_POINT('Ctrl Pts',(10.0667253012217,34.3359882803962,0.0969078380449349));
#56826=CARTESIAN_POINT('Ctrl Pts',(10.2670750393577,34.1526563890204,1.64798730217797E-16));
#56827=CARTESIAN_POINT('Origin',(24.5,8.5,0.));
#56828=CARTESIAN_POINT('',(24.5,15.2746652201978,-22.2639754404033));
#56829=CARTESIAN_POINT('Ctrl Pts',(24.5,5.24229587453786,-8.17819063886291));
#56830=CARTESIAN_POINT('Ctrl Pts',(24.5,7.79421491150921,-11.6489323742096));
#56831=CARTESIAN_POINT('Ctrl Pts',(24.5,11.1172362590846,-16.3395906941412));
#56832=CARTESIAN_POINT('Ctrl Pts',(24.5,15.2746652201978,-22.2639754404033));
#56833=CARTESIAN_POINT('Origin',(24.5,0.,0.));
#56834=CARTESIAN_POINT('Ctrl Pts',(24.5,15.2746649873443,-22.2639756001573));
#56835=CARTESIAN_POINT('Ctrl Pts',(24.5,27.,-14.2195648714001));
#56836=CARTESIAN_POINT('Ctrl Pts',(24.5,27.,0.));
#56837=CARTESIAN_POINT('Ctrl Pts',(24.5,27.,27.));
#56838=CARTESIAN_POINT('Ctrl Pts',(24.5,0.,27.));
#56839=CARTESIAN_POINT('Ctrl Pts',(24.5,-27.,27.));
#56840=CARTESIAN_POINT('Ctrl Pts',(24.5,-27.,0.));
#56841=CARTESIAN_POINT('Ctrl Pts',(24.5,-27.,-27.));
#56842=CARTESIAN_POINT('Ctrl Pts',(24.5,0.,-27.));
#56843=CARTESIAN_POINT('Ctrl Pts',(24.5,8.37155243023015,-27.));
#56844=CARTESIAN_POINT('Ctrl Pts',(24.5,15.2746649873443,-22.2639756001573));
#56845=CARTESIAN_POINT('Ctrl Pts',(24.3078118955742,15.2932132103474,-22.2910110333212));
#56846=CARTESIAN_POINT('Ctrl Pts',(24.3078118955742,27.0327864487698,-14.2368318727032));
#56847=CARTESIAN_POINT('Ctrl Pts',(24.3078118955742,27.0327864487698,0.));
#56848=CARTESIAN_POINT('Ctrl Pts',(24.3078118955742,27.0327864487698,27.0327864487698));
#56849=CARTESIAN_POINT('Ctrl Pts',(24.3078118955742,0.,27.0327864487698));
#56850=CARTESIAN_POINT('Ctrl Pts',(24.3078118955742,-27.0327864487698,27.0327864487698));
#56851=CARTESIAN_POINT('Ctrl Pts',(24.3078118955742,-27.0327864487698,0.));
#56852=CARTESIAN_POINT('Ctrl Pts',(24.3078118955742,-27.0327864487698,-27.0327864487698));
#56853=CARTESIAN_POINT('Ctrl Pts',(24.3078118955742,0.,-27.0327864487698));
#56854=CARTESIAN_POINT('Ctrl Pts',(24.3078118955742,8.38171811448488,-27.0327864487698));
#56855=CARTESIAN_POINT('Ctrl Pts',(24.3078118955742,15.2932132103474,-22.2910110333212));
#56856=CARTESIAN_POINT('Ctrl Pts',(23.9225830034177,15.3326657652955,-22.348516106032));
#56857=CARTESIAN_POINT('Ctrl Pts',(23.9225830034177,27.1025240819344,-14.2735592356203));
#56858=CARTESIAN_POINT('Ctrl Pts',(23.9225830034177,27.1025240819344,0.));
#56859=CARTESIAN_POINT('Ctrl Pts',(23.9225830034177,27.1025240819344,27.1025240819344));
#56860=CARTESIAN_POINT('Ctrl Pts',(23.9225830034177,0.,27.1025240819344));
#56861=CARTESIAN_POINT('Ctrl Pts',(23.9225830034177,-27.1025240819344,27.1025240819344));
#56862=CARTESIAN_POINT('Ctrl Pts',(23.9225830034177,-27.1025240819344,0.));
#56863=CARTESIAN_POINT('Ctrl Pts',(23.9225830034177,-27.1025240819344,-27.1025240819344));
#56864=CARTESIAN_POINT('Ctrl Pts',(23.9225830034177,0.,-27.1025240819344));
#56865=CARTESIAN_POINT('Ctrl Pts',(23.9225830034177,8.40334079049961,-27.1025240819344));
#56866=CARTESIAN_POINT('Ctrl Pts',(23.9225830034177,15.3326657652955,-22.348516106032));
#56867=CARTESIAN_POINT('Ctrl Pts',(23.3421815947946,15.3989129006907,-22.4450762994792));
#56868=CARTESIAN_POINT('Ctrl Pts',(23.3421815947946,27.2196246963933,-14.3352303387232));
#56869=CARTESIAN_POINT('Ctrl Pts',(23.3421815947946,27.2196246963933,0.));
#56870=CARTESIAN_POINT('Ctrl Pts',(23.3421815947946,27.2196246963933,27.2196246963933));
#56871=CARTESIAN_POINT('Ctrl Pts',(23.3421815947946,0.,27.2196246963933));
#56872=CARTESIAN_POINT('Ctrl Pts',(23.3421815947946,-27.2196246963933,27.2196246963933));
#56873=CARTESIAN_POINT('Ctrl Pts',(23.3421815947946,-27.2196246963933,0.));
#56874=CARTESIAN_POINT('Ctrl Pts',(23.3421815947946,-27.2196246963933,-27.2196246963933));
#56875=CARTESIAN_POINT('Ctrl Pts',(23.3421815947946,0.,-27.2196246963933));
#56876=CARTESIAN_POINT('Ctrl Pts',(23.3421815947946,8.43964871396458,-27.2196246963933));
#56877=CARTESIAN_POINT('Ctrl Pts',(23.3421815947946,15.3989129006907,-22.4450762994792));
#56878=CARTESIAN_POINT('Ctrl Pts',(22.5631762070947,15.5014369037694,-22.5945127620704));
#56879=CARTESIAN_POINT('Ctrl Pts',(22.5631762070947,27.4008494948041,-14.4306724786236));
#56880=CARTESIAN_POINT('Ctrl Pts',(22.5631762070947,27.4008494948041,0.));
#56881=CARTESIAN_POINT('Ctrl Pts',(22.5631762070947,27.4008494948041,27.4008494948041));
#56882=CARTESIAN_POINT('Ctrl Pts',(22.5631762070947,0.,27.4008494948041));
#56883=CARTESIAN_POINT('Ctrl Pts',(22.5631762070947,-27.4008494948041,27.4008494948041));
#56884=CARTESIAN_POINT('Ctrl Pts',(22.5631762070947,-27.4008494948041,0.));
#56885=CARTESIAN_POINT('Ctrl Pts',(22.5631762070947,-27.4008494948041,-27.4008494948041));
#56886=CARTESIAN_POINT('Ctrl Pts',(22.5631762070947,0.,-27.4008494948041));
#56887=CARTESIAN_POINT('Ctrl Pts',(22.5631762070947,8.49583882142956,-27.4008494948041));
#56888=CARTESIAN_POINT('Ctrl Pts',(22.5631762070947,15.5014369037694,-22.5945127620704));
#56889=CARTESIAN_POINT('Ctrl Pts',(21.5808622776984,15.6536636723535,-22.8163947519049));
#56890=CARTESIAN_POINT('Ctrl Pts',(21.5808622776984,27.6699305355455,-14.5723841569379));
#56891=CARTESIAN_POINT('Ctrl Pts',(21.5808622776984,27.6699305355455,0.));
#56892=CARTESIAN_POINT('Ctrl Pts',(21.5808622776984,27.6699305355455,27.6699305355455));
#56893=CARTESIAN_POINT('Ctrl Pts',(21.5808622776984,0.,27.6699305355455));
#56894=CARTESIAN_POINT('Ctrl Pts',(21.5808622776984,-27.6699305355455,27.6699305355455));
#56895=CARTESIAN_POINT('Ctrl Pts',(21.5808622776984,-27.6699305355455,0.));
#56896=CARTESIAN_POINT('Ctrl Pts',(21.5808622776984,-27.6699305355455,-27.6699305355455));
#56897=CARTESIAN_POINT('Ctrl Pts',(21.5808622776984,0.,-27.6699305355455));
#56898=CARTESIAN_POINT('Ctrl Pts',(21.5808622776984,8.57926941552391,-27.6699305355455));
#56899=CARTESIAN_POINT('Ctrl Pts',(21.5808622776984,15.6536636723535,-22.8163947519049));
#56900=CARTESIAN_POINT('Ctrl Pts',(20.5902243197586,15.8306138323376,-23.0743129483166));
#56901=CARTESIAN_POINT('Ctrl Pts',(20.5902243197586,27.9827134557292,-14.7371114541311));
#56902=CARTESIAN_POINT('Ctrl Pts',(20.5902243197586,27.9827134557292,0.));
#56903=CARTESIAN_POINT('Ctrl Pts',(20.5902243197586,27.9827134557292,27.9827134557292));
#56904=CARTESIAN_POINT('Ctrl Pts',(20.5902243197586,0.,27.9827134557292));
#56905=CARTESIAN_POINT('Ctrl Pts',(20.5902243197586,-27.9827134557292,27.9827134557292));
#56906=CARTESIAN_POINT('Ctrl Pts',(20.5902243197586,-27.9827134557292,0.));
#56907=CARTESIAN_POINT('Ctrl Pts',(20.5902243197586,-27.9827134557292,-27.9827134557292));
#56908=CARTESIAN_POINT('Ctrl Pts',(20.5902243197586,0.,-27.9827134557292));
#56909=CARTESIAN_POINT('Ctrl Pts',(20.5902243197586,8.6762501049905,-27.9827134557292));
#56910=CARTESIAN_POINT('Ctrl Pts',(20.5902243197586,15.8306138323376,-23.0743129483166));
#56911=CARTESIAN_POINT('Ctrl Pts',(19.591895069338,16.0331232490547,-23.3694856880348));
#56912=CARTESIAN_POINT('Ctrl Pts',(19.591895069338,28.3406757583979,-14.9256324979946));
#56913=CARTESIAN_POINT('Ctrl Pts',(19.591895069338,28.3406757583979,0.));
#56914=CARTESIAN_POINT('Ctrl Pts',(19.591895069338,28.3406757583979,28.3406757583979));
#56915=CARTESIAN_POINT('Ctrl Pts',(19.591895069338,0.,28.3406757583979));
#56916=CARTESIAN_POINT('Ctrl Pts',(19.591895069338,-28.3406757583979,28.3406757583979));
#56917=CARTESIAN_POINT('Ctrl Pts',(19.591895069338,-28.3406757583979,0.));
#56918=CARTESIAN_POINT('Ctrl Pts',(19.591895069338,-28.3406757583979,-28.3406757583979));
#56919=CARTESIAN_POINT('Ctrl Pts',(19.591895069338,0.,-28.3406757583979));
#56920=CARTESIAN_POINT('Ctrl Pts',(19.591895069338,8.78723900072521,-28.3406757583979));
#56921=CARTESIAN_POINT('Ctrl Pts',(19.591895069338,16.0331232490547,-23.3694856880348));
#56922=CARTESIAN_POINT('Ctrl Pts',(18.5871162949016,16.2621527784708,-23.7033134910576));
#56923=CARTESIAN_POINT('Ctrl Pts',(18.5871162949016,28.7455158841458,-15.1388417732027));
#56924=CARTESIAN_POINT('Ctrl Pts',(18.5871162949016,28.7455158841458,0.));
#56925=CARTESIAN_POINT('Ctrl Pts',(18.5871162949016,28.7455158841458,28.7455158841458));
#56926=CARTESIAN_POINT('Ctrl Pts',(18.5871162949016,0.,28.7455158841458));
#56927=CARTESIAN_POINT('Ctrl Pts',(18.5871162949016,-28.7455158841458,28.7455158841458));
#56928=CARTESIAN_POINT('Ctrl Pts',(18.5871162949016,-28.7455158841458,0.));
#56929=CARTESIAN_POINT('Ctrl Pts',(18.5871162949016,-28.7455158841458,-28.7455158841458));
#56930=CARTESIAN_POINT('Ctrl Pts',(18.5871162949016,0.,-28.7455158841458));
#56931=CARTESIAN_POINT('Ctrl Pts',(18.5871162949016,8.91276271696817,-28.7455158841458));
#56932=CARTESIAN_POINT('Ctrl Pts',(18.5871162949016,16.2621527784708,-23.7033134910576));
#56933=CARTESIAN_POINT('Ctrl Pts',(17.577868433379,16.5186756279781,-24.0772148805183));
#56934=CARTESIAN_POINT('Ctrl Pts',(17.577868433379,29.1989541063548,-15.3776452626794));
#56935=CARTESIAN_POINT('Ctrl Pts',(17.577868433379,29.1989541063548,0.));
#56936=CARTESIAN_POINT('Ctrl Pts',(17.577868433379,29.1989541063548,29.1989541063548));
#56937=CARTESIAN_POINT('Ctrl Pts',(17.577868433379,0.,29.1989541063548));
#56938=CARTESIAN_POINT('Ctrl Pts',(17.577868433379,-29.1989541063548,29.1989541063548));
#56939=CARTESIAN_POINT('Ctrl Pts',(17.577868433379,-29.1989541063548,0.));
#56940=CARTESIAN_POINT('Ctrl Pts',(17.577868433379,-29.1989541063548,-29.1989541063548));
#56941=CARTESIAN_POINT('Ctrl Pts',(17.577868433379,0.,-29.1989541063548));
#56942=CARTESIAN_POINT('Ctrl Pts',(17.577868433379,9.053354637379,-29.1989541063548));
#56943=CARTESIAN_POINT('Ctrl Pts',(17.577868433379,16.5186756279781,-24.0772148805183));
#56944=CARTESIAN_POINT('Ctrl Pts',(16.5668667015923,16.8035054746331,-24.4923758520602));
#56945=CARTESIAN_POINT('Ctrl Pts',(16.5668667015923,29.7024287073398,-15.6428004385983));
#56946=CARTESIAN_POINT('Ctrl Pts',(16.5668667015923,29.7024287073398,0.));
#56947=CARTESIAN_POINT('Ctrl Pts',(16.5668667015923,29.7024287073398,29.7024287073398));
#56948=CARTESIAN_POINT('Ctrl Pts',(16.5668667015923,0.,29.7024287073398));
#56949=CARTESIAN_POINT('Ctrl Pts',(16.5668667015923,-29.7024287073398,29.7024287073398));
#56950=CARTESIAN_POINT('Ctrl Pts',(16.5668667015923,-29.7024287073398,0.));
#56951=CARTESIAN_POINT('Ctrl Pts',(16.5668667015923,-29.7024287073398,-29.7024287073398));
#56952=CARTESIAN_POINT('Ctrl Pts',(16.5668667015923,0.,-29.7024287073398));
#56953=CARTESIAN_POINT('Ctrl Pts',(16.5668667015923,9.20946071217291,-29.7024287073398));
#56954=CARTESIAN_POINT('Ctrl Pts',(16.5668667015923,16.8035054746331,-24.4923758520602));
#56955=CARTESIAN_POINT('Ctrl Pts',(15.5576189940876,17.1170945776568,-24.9494556075887));
#56956=CARTESIAN_POINT('Ctrl Pts',(15.5576189940876,30.2567391153688,-15.9347283202968));
#56957=CARTESIAN_POINT('Ctrl Pts',(15.5576189940876,30.2567391153688,0.));
#56958=CARTESIAN_POINT('Ctrl Pts',(15.5576189940876,30.2567391153687,30.2567391153687));
#56959=CARTESIAN_POINT('Ctrl Pts',(15.5576189940876,0.,30.2567391153688));
#56960=CARTESIAN_POINT('Ctrl Pts',(15.5576189940876,-30.2567391153687,30.2567391153687));
#56961=CARTESIAN_POINT('Ctrl Pts',(15.5576189940876,-30.2567391153688,0.));
#56962=CARTESIAN_POINT('Ctrl Pts',(15.5576189940876,-30.2567391153687,-30.2567391153687));
#56963=CARTESIAN_POINT('Ctrl Pts',(15.5576189940876,0.,-30.2567391153688));
#56964=CARTESIAN_POINT('Ctrl Pts',(15.5576189940876,9.38132881007796,-30.2567391153688));
#56965=CARTESIAN_POINT('Ctrl Pts',(15.5576189940876,17.1170945776568,-24.9494556075887));
#56966=CARTESIAN_POINT('Ctrl Pts',(14.5544447688713,17.4593421723157,-25.4483072749091));
#56967=CARTESIAN_POINT('Ctrl Pts',(14.5544447688713,30.8617072153858,-16.2533351033827));
#56968=CARTESIAN_POINT('Ctrl Pts',(14.5544447688713,30.8617072153858,0.));
#56969=CARTESIAN_POINT('Ctrl Pts',(14.5544447688713,30.8617072153858,30.8617072153858));
#56970=CARTESIAN_POINT('Ctrl Pts',(14.5544447688713,0.,30.8617072153858));
#56971=CARTESIAN_POINT('Ctrl Pts',(14.5544447688713,-30.8617072153858,30.8617072153858));
#56972=CARTESIAN_POINT('Ctrl Pts',(14.5544447688713,-30.8617072153858,0.));
#56973=CARTESIAN_POINT('Ctrl Pts',(14.5544447688713,-30.8617072153858,-30.8617072153858));
#56974=CARTESIAN_POINT('Ctrl Pts',(14.5544447688713,0.,-30.8617072153858));
#56975=CARTESIAN_POINT('Ctrl Pts',(14.5544447688713,9.56890370518571,-30.8617072153858));
#56976=CARTESIAN_POINT('Ctrl Pts',(14.5544447688713,17.4593421723157,-25.4483072749091));
#56977=CARTESIAN_POINT('Ctrl Pts',(13.5625963827217,17.8292752645412,-25.9875126418238));
#56978=CARTESIAN_POINT('Ctrl Pts',(13.5625963827217,31.5156131110873,-16.5977150035204));
#56979=CARTESIAN_POINT('Ctrl Pts',(13.5625963827217,31.5156131110873,0.));
#56980=CARTESIAN_POINT('Ctrl Pts',(13.5625963827217,31.5156131110873,31.5156131110873));
#56981=CARTESIAN_POINT('Ctrl Pts',(13.5625963827217,0.,31.5156131110873));
#56982=CARTESIAN_POINT('Ctrl Pts',(13.5625963827217,-31.5156131110873,31.5156131110873));
#56983=CARTESIAN_POINT('Ctrl Pts',(13.5625963827217,-31.5156131110873,0.));
#56984=CARTESIAN_POINT('Ctrl Pts',(13.5625963827217,-31.5156131110873,-31.5156131110873));
#56985=CARTESIAN_POINT('Ctrl Pts',(13.5625963827217,0.,-31.5156131110873));
#56986=CARTESIAN_POINT('Ctrl Pts',(13.5625963827217,9.77165213075244,-31.5156131110873));
#56987=CARTESIAN_POINT('Ctrl Pts',(13.5625963827217,17.8292752645412,-25.9875126418238));
#56988=CARTESIAN_POINT('Ctrl Pts',(12.5880795783847,18.2250438427861,-26.5643751770515));
#56989=CARTESIAN_POINT('Ctrl Pts',(12.5880795783847,32.2151866612413,-16.966145799029));
#56990=CARTESIAN_POINT('Ctrl Pts',(12.5880795783847,32.2151866612413,0.));
#56991=CARTESIAN_POINT('Ctrl Pts',(12.5880795783847,32.2151866612413,32.2151866612413));
#56992=CARTESIAN_POINT('Ctrl Pts',(12.5880795783847,0.,32.2151866612413));
#56993=CARTESIAN_POINT('Ctrl Pts',(12.5880795783847,-32.2151866612413,32.2151866612413));
#56994=CARTESIAN_POINT('Ctrl Pts',(12.5880795783847,-32.2151866612413,0.));
#56995=CARTESIAN_POINT('Ctrl Pts',(12.5880795783847,-32.2151866612413,-32.2151866612413));
#56996=CARTESIAN_POINT('Ctrl Pts',(12.5880795783847,0.,-32.2151866612413));
#56997=CARTESIAN_POINT('Ctrl Pts',(12.5880795783847,9.98856015497159,-32.2151866612413));
#56998=CARTESIAN_POINT('Ctrl Pts',(12.5880795783847,18.2250438427861,-26.5643751770515));
#56999=CARTESIAN_POINT('Ctrl Pts',(11.6370973936883,18.6443245145603,-27.1755083609041));
#57000=CARTESIAN_POINT('Ctrl Pts',(11.6370973936883,32.9563209608992,-17.3564645861551));
#57001=CARTESIAN_POINT('Ctrl Pts',(11.6370973936883,32.9563209608992,0.));
#57002=CARTESIAN_POINT('Ctrl Pts',(11.6370973936883,32.9563209608992,32.9563209608992));
#57003=CARTESIAN_POINT('Ctrl Pts',(11.6370973936883,0.,32.9563209608992));
#57004=CARTESIAN_POINT('Ctrl Pts',(11.6370973936883,-32.9563209608992,32.9563209608992));
#57005=CARTESIAN_POINT('Ctrl Pts',(11.6370973936883,-32.9563209608992,0.));
#57006=CARTESIAN_POINT('Ctrl Pts',(11.6370973936883,-32.9563209608992,-32.9563209608992));
#57007=CARTESIAN_POINT('Ctrl Pts',(11.6370973936883,0.,-32.9563209608992));
#57008=CARTESIAN_POINT('Ctrl Pts',(11.6370973936883,10.2183544011726,-32.9563209608992));
#57009=CARTESIAN_POINT('Ctrl Pts',(11.6370973936883,18.6443245145603,-27.1755083609041));
#57010=CARTESIAN_POINT('Ctrl Pts',(10.7155646400367,19.084590376709,-27.8172290415595));
#57011=CARTESIAN_POINT('Ctrl Pts',(10.7155646400367,33.7345493729701,-17.7663190080147));
#57012=CARTESIAN_POINT('Ctrl Pts',(10.7155646400367,33.7345493729701,0.));
#57013=CARTESIAN_POINT('Ctrl Pts',(10.7155646400367,33.7345493729701,33.7345493729701));
#57014=CARTESIAN_POINT('Ctrl Pts',(10.7155646400367,0.,33.7345493729701));
#57015=CARTESIAN_POINT('Ctrl Pts',(10.7155646400367,-33.7345493729701,33.7345493729701));
#57016=CARTESIAN_POINT('Ctrl Pts',(10.7155646400367,-33.7345493729701,0.));
#57017=CARTESIAN_POINT('Ctrl Pts',(10.7155646400367,-33.7345493729701,-33.7345493729701));
#57018=CARTESIAN_POINT('Ctrl Pts',(10.7155646400367,0.,-33.7345493729701));
#57019=CARTESIAN_POINT('Ctrl Pts',(10.7155646400367,10.4596499550373,-33.7345493729701));
#57020=CARTESIAN_POINT('Ctrl Pts',(10.7155646400367,19.084590376709,-27.8172290415595));
#57021=CARTESIAN_POINT('Ctrl Pts',(9.82859575068344,19.5433963611581,-28.485973347994));
#57022=CARTESIAN_POINT('Ctrl Pts',(9.82859575068344,34.5455499147423,-18.1934328900321));
#57023=CARTESIAN_POINT('Ctrl Pts',(9.82859575068344,34.5455499147423,0.));
#57024=CARTESIAN_POINT('Ctrl Pts',(9.82859575068344,34.5455499147423,34.5455499147423));
#57025=CARTESIAN_POINT('Ctrl Pts',(9.82859575068344,0.,34.5455499147423));
#57026=CARTESIAN_POINT('Ctrl Pts',(9.82859575068344,-34.5455499147423,34.5455499147423));
#57027=CARTESIAN_POINT('Ctrl Pts',(9.82859575068344,-34.5455499147423,0.));
#57028=CARTESIAN_POINT('Ctrl Pts',(9.82859575068344,-34.5455499147423,-34.5455499147423));
#57029=CARTESIAN_POINT('Ctrl Pts',(9.82859575068344,0.,-34.5455499147423));
#57030=CARTESIAN_POINT('Ctrl Pts',(9.82859575068344,10.7111067534221,-34.5455499147423));
#57031=CARTESIAN_POINT('Ctrl Pts',(9.82859575068344,19.5433963611581,-28.485973347994));
#57032=CARTESIAN_POINT('Ctrl Pts',(8.97989469943246,20.0186512506371,-29.1786931734031));
#57033=CARTESIAN_POINT('Ctrl Pts',(8.97989469943246,35.3856260818179,-18.6358594661302));
#57034=CARTESIAN_POINT('Ctrl Pts',(8.97989469943246,35.3856260818179,0.));
#57035=CARTESIAN_POINT('Ctrl Pts',(8.97989469943246,35.3856260818179,35.3856260818179));
#57036=CARTESIAN_POINT('Ctrl Pts',(8.97989469943246,0.,35.3856260818179));
#57037=CARTESIAN_POINT('Ctrl Pts',(8.97989469943246,-35.3856260818179,35.3856260818179));
#57038=CARTESIAN_POINT('Ctrl Pts',(8.97989469943246,-35.3856260818179,0.));
#57039=CARTESIAN_POINT('Ctrl Pts',(8.97989469943246,-35.3856260818179,-35.3856260818179));
#57040=CARTESIAN_POINT('Ctrl Pts',(8.97989469943246,0.,-35.3856260818179));
#57041=CARTESIAN_POINT('Ctrl Pts',(8.97989469943246,10.9715786674244,-35.3856260818179));
#57042=CARTESIAN_POINT('Ctrl Pts',(8.97989469943246,20.0186512506371,-29.1786931734031));
#57043=CARTESIAN_POINT('Ctrl Pts',(8.1713316609345,20.5088253880975,-29.8931589273354));
#57044=CARTESIAN_POINT('Ctrl Pts',(8.1713316609345,36.2520740021093,-19.0921747405847));
#57045=CARTESIAN_POINT('Ctrl Pts',(8.1713316609345,36.2520740021093,0.));
#57046=CARTESIAN_POINT('Ctrl Pts',(8.1713316609345,36.2520740021093,36.2520740021093));
#57047=CARTESIAN_POINT('Ctrl Pts',(8.1713316609345,0.,36.2520740021093));
#57048=CARTESIAN_POINT('Ctrl Pts',(8.1713316609345,-36.2520740021093,36.2520740021093));
#57049=CARTESIAN_POINT('Ctrl Pts',(8.1713316609345,-36.2520740021093,0.));
#57050=CARTESIAN_POINT('Ctrl Pts',(8.1713316609345,-36.2520740021093,-36.2520740021093));
#57051=CARTESIAN_POINT('Ctrl Pts',(8.1713316609345,0.,-36.2520740021093));
#57052=CARTESIAN_POINT('Ctrl Pts',(8.1713316609345,11.2402273412312,-36.2520740021093));
#57053=CARTESIAN_POINT('Ctrl Pts',(8.1713316609345,20.5088253880975,-29.8931589273354));
#57054=CARTESIAN_POINT('Ctrl Pts',(7.40358438374929,21.0128566018474,-30.6278224144852));
#57055=CARTESIAN_POINT('Ctrl Pts',(7.40358438374929,37.1430161460138,-19.5613899113964));
#57056=CARTESIAN_POINT('Ctrl Pts',(7.40358438374929,37.1430161460139,0.));
#57057=CARTESIAN_POINT('Ctrl Pts',(7.40358438374929,37.1430161460138,37.1430161460138));
#57058=CARTESIAN_POINT('Ctrl Pts',(7.40358438374929,0.,37.1430161460139));
#57059=CARTESIAN_POINT('Ctrl Pts',(7.40358438374929,-37.1430161460138,37.1430161460138));
#57060=CARTESIAN_POINT('Ctrl Pts',(7.40358438374929,-37.1430161460139,0.));
#57061=CARTESIAN_POINT('Ctrl Pts',(7.40358438374929,-37.1430161460138,-37.1430161460138));
#57062=CARTESIAN_POINT('Ctrl Pts',(7.40358438374929,0.,-37.1430161460139));
#57063=CARTESIAN_POINT('Ctrl Pts',(7.40358438374929,11.5164706327126,-37.1430161460138));
#57064=CARTESIAN_POINT('Ctrl Pts',(7.40358438374929,21.0128566018474,-30.6278224144852));
#57065=CARTESIAN_POINT('Ctrl Pts',(6.82198164612729,21.426644412938,-31.2309493398479));
#57066=CARTESIAN_POINT('Ctrl Pts',(6.82198164612729,37.8744410845445,-19.946595258137));
#57067=CARTESIAN_POINT('Ctrl Pts',(6.82198164612729,37.8744410845445,0.));
#57068=CARTESIAN_POINT('Ctrl Pts',(6.82198164612729,37.8744410845445,37.8744410845445));
#57069=CARTESIAN_POINT('Ctrl Pts',(6.82198164612729,0.,37.8744410845445));
#57070=CARTESIAN_POINT('Ctrl Pts',(6.82198164612729,-37.8744410845445,37.8744410845445));
#57071=CARTESIAN_POINT('Ctrl Pts',(6.82198164612729,-37.8744410845445,0.));
#57072=CARTESIAN_POINT('Ctrl Pts',(6.82198164612729,-37.8744410845445,-37.8744410845445));
#57073=CARTESIAN_POINT('Ctrl Pts',(6.82198164612729,0.,-37.8744410845445));
#57074=CARTESIAN_POINT('Ctrl Pts',(6.82198164612729,11.743254418701,-37.8744410845445));
#57075=CARTESIAN_POINT('Ctrl Pts',(6.82198164612729,21.426644412938,-31.2309493398479));
#57076=CARTESIAN_POINT('Ctrl Pts',(6.40395249919757,21.7427802361891,-31.6917411320757));
#57077=CARTESIAN_POINT('Ctrl Pts',(6.40395249919757,38.433253158973,-20.2408939449244));
#57078=CARTESIAN_POINT('Ctrl Pts',(6.40395249919757,38.433253158973,0.));
#57079=CARTESIAN_POINT('Ctrl Pts',(6.40395249919757,38.433253158973,38.433253158973));
#57080=CARTESIAN_POINT('Ctrl Pts',(6.40395249919757,0.,38.433253158973));
#57081=CARTESIAN_POINT('Ctrl Pts',(6.40395249919757,-38.433253158973,38.433253158973));
#57082=CARTESIAN_POINT('Ctrl Pts',(6.40395249919757,-38.433253158973,0.));
#57083=CARTESIAN_POINT('Ctrl Pts',(6.40395249919757,-38.433253158973,-38.433253158973));
#57084=CARTESIAN_POINT('Ctrl Pts',(6.40395249919757,0.,-38.433253158973));
#57085=CARTESIAN_POINT('Ctrl Pts',(6.40395249919757,11.9165182920241,-38.433253158973));
#57086=CARTESIAN_POINT('Ctrl Pts',(6.40395249919757,21.7427802361891,-31.6917411320757));
#57087=CARTESIAN_POINT('Ctrl Pts',(6.13331019225912,21.9561025509032,-32.0026744856845));
#57088=CARTESIAN_POINT('Ctrl Pts',(6.13331019225912,38.8103286956251,-20.4394809839926));
#57089=CARTESIAN_POINT('Ctrl Pts',(6.13331019225912,38.8103286956251,0.));
#57090=CARTESIAN_POINT('Ctrl Pts',(6.13331019225912,38.8103286956251,38.8103286956251));
#57091=CARTESIAN_POINT('Ctrl Pts',(6.13331019225912,0.,38.8103286956251));
#57092=CARTESIAN_POINT('Ctrl Pts',(6.13331019225912,-38.8103286956251,38.8103286956251));
#57093=CARTESIAN_POINT('Ctrl Pts',(6.13331019225912,-38.8103286956251,0.));
#57094=CARTESIAN_POINT('Ctrl Pts',(6.13331019225912,-38.8103286956251,-38.8103286956251));
#57095=CARTESIAN_POINT('Ctrl Pts',(6.13331019225912,0.,-38.8103286956251));
#57096=CARTESIAN_POINT('Ctrl Pts',(6.13331019225912,12.0334333892552,-38.8103286956251));
#57097=CARTESIAN_POINT('Ctrl Pts',(6.13331019225912,21.9561025509032,-32.0026744856845));
#57098=CARTESIAN_POINT('Ctrl Pts',(6.,22.0634049817195,-32.1590758668939));
#57099=CARTESIAN_POINT('Ctrl Pts',(6.,39.,-20.5393714809112));
#57100=CARTESIAN_POINT('Ctrl Pts',(6.,39.,0.));
#57101=CARTESIAN_POINT('Ctrl Pts',(6.,39.,39.));
#57102=CARTESIAN_POINT('Ctrl Pts',(6.,0.,39.));
#57103=CARTESIAN_POINT('Ctrl Pts',(6.,-39.,39.));
#57104=CARTESIAN_POINT('Ctrl Pts',(6.,-39.,0.));
#57105=CARTESIAN_POINT('Ctrl Pts',(6.,-39.,-39.));
#57106=CARTESIAN_POINT('Ctrl Pts',(6.,0.,-39.));
#57107=CARTESIAN_POINT('Ctrl Pts',(6.,12.0922423992213,-39.));
#57108=CARTESIAN_POINT('Ctrl Pts',(6.,22.0634049817195,-32.1590758668939));
#57109=CARTESIAN_POINT('Ctrl Pts',(24.5,15.2746652201978,-22.2639754404033));
#57110=CARTESIAN_POINT('Ctrl Pts',(23.5178991898112,17.7900297317948,-20.7414389863023));
#57111=CARTESIAN_POINT('Ctrl Pts',(22.3947886245986,20.0495645305202,-18.9195767222114));
#57112=CARTESIAN_POINT('Ctrl Pts',(21.1743874927566,22.0660835472267,-16.915405191777));
#57113=CARTESIAN_POINT('Ctrl Pts',(20.5031871793432,23.1751354488541,-15.8131442021206));
#57114=CARTESIAN_POINT('Ctrl Pts',(19.8411792966403,24.2071629062566,-14.6351278759304));
#57115=CARTESIAN_POINT('Ctrl Pts',(19.1295827650253,25.1714380797582,-13.4354459468032));
#57116=CARTESIAN_POINT('Ctrl Pts',(18.8261415870907,25.5826272600038,-12.9238738950185));
#57117=CARTESIAN_POINT('Ctrl Pts',(18.5104994276268,25.9850411393693,-12.404332641861));
#57118=CARTESIAN_POINT('Ctrl Pts',(18.2016639423759,26.3553711077349,-11.9183617880446));
#57119=CARTESIAN_POINT('Ctrl Pts',(17.6747132403628,26.987246802486,-11.0891737743408));
#57120=CARTESIAN_POINT('Ctrl Pts',(17.2016343370984,27.5228289338585,-10.3269493110331));
#57121=CARTESIAN_POINT('Ctrl Pts',(16.8729352926451,27.8805533220886,-9.81400929094393));
#57122=CARTESIAN_POINT('Ctrl Pts',(16.6342454025473,28.1403204140616,-9.44152996954687));
#57123=CARTESIAN_POINT('Ctrl Pts',(16.5014949770662,28.2793135182913,-9.23929506825468));
#57124=CARTESIAN_POINT('Ctrl Pts',(16.3424569562978,28.4442683427237,-9.00014216371263));
#57125=CARTESIAN_POINT('Ctrl Pts',(15.993118510103,28.8066034735382,-8.47482561568167));
#57126=CARTESIAN_POINT('Ctrl Pts',(15.6312480487537,29.1643380375821,-7.95419476716189));
#57127=CARTESIAN_POINT('Ctrl Pts',(15.2503296894305,29.5245094879835,-7.44978258413541));
#57128=CARTESIAN_POINT('Ctrl Pts',(14.7484414179076,29.9990621638247,-6.78518201428077));
#57129=CARTESIAN_POINT('Ctrl Pts',(14.2669345517206,30.4475318788827,-6.13744034835409));
#57130=CARTESIAN_POINT('Ctrl Pts',(13.7912435751455,30.8800117840353,-5.54611601085555));
#57131=CARTESIAN_POINT('Ctrl Pts',(13.5533980868579,31.0962517366116,-5.25045384210628));
#57132=CARTESIAN_POINT('Ctrl Pts',(13.3161115657262,31.3096390113264,-4.9671616086599));
#57133=CARTESIAN_POINT('Ctrl Pts',(13.0766514227367,31.5235559498616,-4.69823014337086));
#57134=CARTESIAN_POINT('Ctrl Pts',(12.9188702359555,31.6645066233779,-4.52103019173643));
#57135=CARTESIAN_POINT('Ctrl Pts',(12.7601526360409,31.8056928422568,-4.35006042750501));
#57136=CARTESIAN_POINT('Ctrl Pts',(12.5997389313808,31.9481916423883,-4.1859403999119));
#57137=CARTESIAN_POINT('Ctrl Pts',(12.5166971934814,32.0219593297351,-4.10098000114603));
#57138=CARTESIAN_POINT('Ctrl Pts',(12.4397215765388,32.0902904057789,-4.02412719470386));
#57139=CARTESIAN_POINT('Ctrl Pts',(12.3478597934844,32.1718560071766,-3.93542897845831));
#57140=CARTESIAN_POINT('Ctrl Pts',(11.9116121727781,32.5592075080742,-3.51420499922096));
#57141=CARTESIAN_POINT('Ctrl Pts',(10.7144663992386,33.6238209182471,-2.28350062373506));
#57142=CARTESIAN_POINT('Ctrl Pts',(9.56604185022483,34.7743191636545,-1.6807321648514));
#57143=CARTESIAN_POINT('Ctrl Pts',(9.07284645450772,35.2684051163649,-1.42187090238518));
#57144=CARTESIAN_POINT('Ctrl Pts',(8.57333454992768,35.7900679626755,-1.25277516408929));
#57145=CARTESIAN_POINT('Ctrl Pts',(8.00348148263049,36.4414959462974,-1.11294819927946));
#57146=CARTESIAN_POINT('Ctrl Pts',(7.63919428965959,36.8579311384459,-1.02356169697667));
#57147=CARTESIAN_POINT('Ctrl Pts',(7.2438864438469,37.3374667334074,-0.951049621039589));
#57148=CARTESIAN_POINT('Ctrl Pts',(6.94254646282579,37.7220011048021,-0.902244736766912));
#57149=CARTESIAN_POINT('Ctrl Pts',(6.91433564865295,37.7580004025312,-0.897675726321375));
#57150=CARTESIAN_POINT('Ctrl Pts',(6.88669635040567,37.7934387743179,-0.89325998801799));
#57151=CARTESIAN_POINT('Ctrl Pts',(6.85962514029878,37.8283036072989,-0.888985319768479));
#57152=CARTESIAN_POINT('Ctrl Pts',(6.44000062073739,38.368735258912,-0.822724683343163));
#57153=CARTESIAN_POINT('Ctrl Pts',(6.15412442492902,38.7718575486186,-0.828800771638793));
#57154=CARTESIAN_POINT('Ctrl Pts',(6.,38.9911990462069,-0.828490759799982));
#57155=CARTESIAN_POINT('Ctrl Pts',(2.09999999999999,9.70057967382468,-0.9));
#57156=CARTESIAN_POINT('Ctrl Pts',(2.73333333333332,9.70057967382468,-0.9));
#57157=CARTESIAN_POINT('Ctrl Pts',(3.36699574607395,9.70059005321194,-0.899942825180981));
#57158=CARTESIAN_POINT('Ctrl Pts',(4.12579817395472,9.70059327517204,-0.899925538426819));
#57159=CARTESIAN_POINT('Ctrl Pts',(4.38275749788984,9.7007262380907,-0.898639486126413));
#57160=CARTESIAN_POINT('Ctrl Pts',(4.88872023230434,9.7013226080202,-0.892940393354486));
#57161=CARTESIAN_POINT('Ctrl Pts',(5.76576815117897,9.7027126091003,-0.879800331845227));
#57162=CARTESIAN_POINT('Ctrl Pts',(6.49294800367276,9.70272682384117,-0.880004039269183));
#57163=CARTESIAN_POINT('Ctrl Pts',(7.02334978980851,9.7003499446892,-0.901450813685861));
#57164=CARTESIAN_POINT('Ctrl Pts',(7.14973151012377,9.69983015215563,-0.906734178368804));
#57165=CARTESIAN_POINT('Ctrl Pts',(7.39956059419753,9.69883105549345,-0.917970126739818));
#57166=CARTESIAN_POINT('Ctrl Pts',(7.71335439531399,9.69758466503641,-0.933748103679502));
#57167=CARTESIAN_POINT('Ctrl Pts',(8.08760778694771,9.69583752317872,-0.956004462473258));
#57168=CARTESIAN_POINT('Ctrl Pts',(8.58202753816148,9.69285898041634,-0.99085924708594));
#57169=CARTESIAN_POINT('Ctrl Pts',(9.18585213220259,9.68729348127799,-1.04563537764413));
#57170=CARTESIAN_POINT('Ctrl Pts',(9.64252060159779,9.67961272832539,-1.10407520282726));
#57171=CARTESIAN_POINT('Ctrl Pts',(10.3691727925248,9.66316415892935,-1.21502210418074));
#57172=CARTESIAN_POINT('Ctrl Pts',(11.1023934939471,9.64291586397951,-1.37505182297649));
#57173=CARTESIAN_POINT('Ctrl Pts',(12.0425471796807,9.60260179231032,-1.63666268571367));
#57174=CARTESIAN_POINT('Ctrl Pts',(12.4995913073701,9.57670316757122,-1.77585592157297));
#57175=CARTESIAN_POINT('Ctrl Pts',(13.0011491477499,9.54392598331016,-1.93113784163963));
#57176=CARTESIAN_POINT('Ctrl Pts',(13.5006102383397,9.50612955297879,-2.1025105735227));
#57177=CARTESIAN_POINT('Ctrl Pts',(14.4710708057365,9.41550916749915,-2.48724983034416));
#57178=CARTESIAN_POINT('Ctrl Pts',(15.1518257104396,9.32856897303256,-2.79923279354156));
#57179=CARTESIAN_POINT('Ctrl Pts',(15.8845791715993,9.2156036499786,-3.13372913998994));
#57180=CARTESIAN_POINT('Ctrl Pts',(16.3870096096401,9.12766425587705,-3.3785113296341));
#57181=CARTESIAN_POINT('Ctrl Pts',(17.3639693983226,8.92220955647037,-3.90025233998292));
#57182=CARTESIAN_POINT('Ctrl Pts',(18.0500449337391,8.73620009317483,-4.29999527322685));
#57183=CARTESIAN_POINT('Ctrl Pts',(18.7841974918272,8.5100601990801,-4.71761880736));
#57184=CARTESIAN_POINT('Ctrl Pts',(19.2877316715229,8.33770758255159,-5.01626902913314));
#57185=CARTESIAN_POINT('Ctrl Pts',(20.270830255076,7.94468607642615,-5.63097621657333));
#57186=CARTESIAN_POINT('Ctrl Pts',(20.9685752777043,7.60361048672244,-6.08039129179283));
#57187=CARTESIAN_POINT('Ctrl Pts',(22.6570444653075,6.7053439134869,-7.10435307734314));
#57188=CARTESIAN_POINT('Ctrl Pts',(23.7241254823866,5.94930970418605,-7.73257301523402));
#57189=CARTESIAN_POINT('Ctrl Pts',(24.6950729185821,5.06818763168846,-8.29049117070007));
#57190=CARTESIAN_POINT('Ctrl Pts',(2.09999999999999,12.4900227849924,-0.9));
#57191=CARTESIAN_POINT('Ctrl Pts',(2.73333333333333,12.4900227849924,-0.9));
#57192=CARTESIAN_POINT('Ctrl Pts',(3.36711593286258,12.4900350732685,-0.899923338257865));
#57193=CARTESIAN_POINT('Ctrl Pts',(4.12606108559101,12.4900388828623,-0.899900267382887));
#57194=CARTESIAN_POINT('Ctrl Pts',(4.38492166674737,12.4901766322851,-0.898235423402214));
#57195=CARTESIAN_POINT('Ctrl Pts',(4.89214186044569,12.4907940394702,-0.890880104482316));
#57196=CARTESIAN_POINT('Ctrl Pts',(5.76871669674148,12.4922331404629,-0.873964960821528));
#57197=CARTESIAN_POINT('Ctrl Pts',(6.48935737656207,12.4922496348677,-0.874303891764717));
#57198=CARTESIAN_POINT('Ctrl Pts',(7.01200280711183,12.4897914851075,-0.901601722722426));
#57199=CARTESIAN_POINT('Ctrl Pts',(7.13826357206355,12.4892638554664,-0.908398677788786));
#57200=CARTESIAN_POINT('Ctrl Pts',(7.38673691586477,12.4882832497312,-0.922805797286931));
#57201=CARTESIAN_POINT('Ctrl Pts',(7.69892824648965,12.4871080942582,-0.943038576261421));
#57202=CARTESIAN_POINT('Ctrl Pts',(8.0705664804814,12.4854686042712,-0.971544342930977));
#57203=CARTESIAN_POINT('Ctrl Pts',(8.56088758368331,12.4825959523084,-1.01613710264616));
#57204=CARTESIAN_POINT('Ctrl Pts',(9.15814513041246,12.4769595906258,-1.08610160656213));
#57205=CARTESIAN_POINT('Ctrl Pts',(9.60777554034275,12.468746296037,-1.16049917233183));
#57206=CARTESIAN_POINT('Ctrl Pts',(10.3209062172087,12.4508324485273,-1.30136035149208));
#57207=CARTESIAN_POINT('Ctrl Pts',(11.0425437394732,12.4295262892971,-1.50493234803139));
#57208=CARTESIAN_POINT('Ctrl Pts',(11.9742896318204,12.3853339611956,-1.8399228903873));
#57209=CARTESIAN_POINT('Ctrl Pts',(12.4288761309409,12.3560398614547,-2.01876820477874));
#57210=CARTESIAN_POINT('Ctrl Pts',(12.9286708179861,12.3183165430442,-2.21862458063622));
#57211=CARTESIAN_POINT('Ctrl Pts',(13.4199962589649,12.2751874773222,-2.43712366209172));
#57212=CARTESIAN_POINT('Ctrl Pts',(14.3833021834327,12.1705259624137,-2.9310172387322));
#57213=CARTESIAN_POINT('Ctrl Pts',(15.0609069806317,12.0681822043469,-3.33319508099636));
#57214=CARTESIAN_POINT('Ctrl Pts',(15.7927902555254,11.932649685131,-3.76590395503156));
#57215=CARTESIAN_POINT('Ctrl Pts',(16.2911579735696,11.8276689824143,-4.0808892056978));
#57216=CARTESIAN_POINT('Ctrl Pts',(17.2659787139141,11.5797551229758,-4.75590720934297));
#57217=CARTESIAN_POINT('Ctrl Pts',(17.9510813915698,11.352641285026,-5.27484524120805));
#57218=CARTESIAN_POINT('Ctrl Pts',(18.6848997382068,11.074158593171,-5.81807378002929));
#57219=CARTESIAN_POINT('Ctrl Pts',(19.1880319937622,10.8620643305274,-6.20661118455775));
#57220=CARTESIAN_POINT('Ctrl Pts',(20.172357775901,10.3750481164233,-7.00893220254037));
#57221=CARTESIAN_POINT('Ctrl Pts',(20.8704864843064,9.94949961190826,-7.59709821983438));
#57222=CARTESIAN_POINT('Ctrl Pts',(22.5588413378293,8.82437146010007,-8.93943031422903));
#57223=CARTESIAN_POINT('Ctrl Pts',(23.6292145427077,7.87024728938886,-9.77160798313874));
#57224=CARTESIAN_POINT('Ctrl Pts',(24.6070641578141,6.74729640798646,-10.5188587391465));
#57225=CARTESIAN_POINT('Ctrl Pts',(2.09999999999999,18.0689090073278,-0.9));
#57226=CARTESIAN_POINT('Ctrl Pts',(2.73333333333332,18.0689090073278,-0.9));
#57227=CARTESIAN_POINT('Ctrl Pts',(3.36736559419821,18.0689314789609,-0.899865425636373));
#57228=CARTESIAN_POINT('Ctrl Pts',(4.12659875622228,18.0689384409667,-0.899825122261498));
#57229=CARTESIAN_POINT('Ctrl Pts',(4.38926345438438,18.0690862846866,-0.897386117530702));
#57230=CARTESIAN_POINT('Ctrl Pts',(4.89899520603675,18.069746945452,-0.886685515381575));
#57231=CARTESIAN_POINT('Ctrl Pts',(5.77464038746463,18.071286009881,-0.86222188815569));
#57232=CARTESIAN_POINT('Ctrl Pts',(6.48217933907112,18.0713158624184,-0.862943428769206));
#57233=CARTESIAN_POINT('Ctrl Pts',(6.98941530816473,18.0686994298788,-0.901392822899508));
#57234=CARTESIAN_POINT('Ctrl Pts',(7.11543652137778,18.0681565331617,-0.911206755481794));
#57235=CARTESIAN_POINT('Ctrl Pts',(7.36121956286345,18.0672138729335,-0.93185221447469));
#57236=CARTESIAN_POINT('Ctrl Pts',(7.67024245563845,18.0661849478685,-0.960846457117527));
#57237=CARTESIAN_POINT('Ctrl Pts',(8.03672088388777,18.0647641042642,-1.00158789539943));
#57238=CARTESIAN_POINT('Ctrl Pts',(8.51901276891291,18.0621154200779,-1.06515019836488));
#57239=CARTESIAN_POINT('Ctrl Pts',(9.10353634573336,18.0563613895553,-1.16450313421632));
#57240=CARTESIAN_POINT('Ctrl Pts',(9.53996031439373,18.0471397487516,-1.26934809663657));
#57241=CARTESIAN_POINT('Ctrl Pts',(10.2286868726423,18.0264576771242,-1.4667114867886));
#57242=CARTESIAN_POINT('Ctrl Pts',(10.9322529814026,18.0033848030989,-1.75351833023026));
#57243=CARTESIAN_POINT('Ctrl Pts',(11.8534175309074,17.9519701461305,-2.23291342512525));
#57244=CARTESIAN_POINT('Ctrl Pts',(12.3052433854515,17.9161742014927,-2.49039272798436));
#57245=CARTESIAN_POINT('Ctrl Pts',(12.8031166247441,17.8688536207807,-2.77894324840396));
#57246=CARTESIAN_POINT('Ctrl Pts',(13.2871795523955,17.8155736163136,-3.09023041616086));
#57247=CARTESIAN_POINT('Ctrl Pts',(14.2486094030008,17.6833109363502,-3.80395063248038));
#57248=CARTESIAN_POINT('Ctrl Pts',(14.9265925530568,17.5504089048378,-4.38797919240388));
#57249=CARTESIAN_POINT('Ctrl Pts',(15.6587039975819,17.3701999174313,-5.01739464023764));
#57250=CARTESIAN_POINT('Ctrl Pts',(16.159865983277,17.2304652392218,-5.47692008190156));
#57251=CARTESIAN_POINT('Ctrl Pts',(17.1407994058435,16.8957016774365,-6.46562803933544));
#57252=CARTESIAN_POINT('Ctrl Pts',(17.8296343470588,16.5850049496136,-7.22640249819829));
#57253=CARTESIAN_POINT('Ctrl Pts',(18.56460273973,16.2014274362579,-8.0214716671563));
#57254=CARTESIAN_POINT('Ctrl Pts',(19.0748031274678,15.9062727033236,-8.59692120486745));
#57255=CARTESIAN_POINT('Ctrl Pts',(20.0668883298028,15.2256796563853,-9.78160896677002));
#57256=CARTESIAN_POINT('Ctrl Pts',(20.7688293710982,14.6278203429455,-10.649754812288));
#57257=CARTESIAN_POINT('Ctrl Pts',(22.4601426409202,13.0448722721453,-12.628814335545));
#57258=CARTESIAN_POINT('Ctrl Pts',(23.5475123664675,11.6790030585503,-13.8811542175352));
#57259=CARTESIAN_POINT('Ctrl Pts',(24.5367146907742,10.0590378761085,-15.0082084052888));
#57260=CARTESIAN_POINT('Ctrl Pts',(2.09999999999999,27.8319598964147,-0.9));
#57261=CARTESIAN_POINT('Ctrl Pts',(2.73333333333333,27.8319598964147,-0.9));
#57262=CARTESIAN_POINT('Ctrl Pts',(3.36789044795187,27.8319876241424,-0.89982221409351));
#57263=CARTESIAN_POINT('Ctrl Pts',(4.12765289629168,27.831996167011,-0.89977046921849));
#57264=CARTESIAN_POINT('Ctrl Pts',(4.39698725464062,27.8321607554124,-0.895929159974803));
#57265=CARTESIAN_POINT('Ctrl Pts',(4.91109827079468,27.8328943097031,-0.879282199143232));
#57266=CARTESIAN_POINT('Ctrl Pts',(5.78522928181945,27.8346056768937,-0.84165461313598));
#57267=CARTESIAN_POINT('Ctrl Pts',(6.46973294865984,27.8346392832047,-0.843590781671977));
#57268=CARTESIAN_POINT('Ctrl Pts',(6.95067651024836,27.8317418569026,-0.899765981581546));
#57269=CARTESIAN_POINT('Ctrl Pts',(7.07629429939615,27.8311726695747,-0.914829100774546));
#57270=CARTESIAN_POINT('Ctrl Pts',(7.31750539815411,27.830297898526,-0.946050159135031));
#57271=CARTESIAN_POINT('Ctrl Pts',(7.62122509886065,27.8295244439959,-0.9899356060868));
#57272=CARTESIAN_POINT('Ctrl Pts',(7.97911623757604,27.8284951948722,-1.05124515340815));
#57273=CARTESIAN_POINT('Ctrl Pts',(8.44841085954398,27.8262539604227,-1.14651171885001));
#57274=CARTESIAN_POINT('Ctrl Pts',(9.01306407988194,27.8203481205507,-1.29445151760389));
#57275=CARTESIAN_POINT('Ctrl Pts',(9.43128909448383,27.8094728330774,-1.44915600718223));
#57276=CARTESIAN_POINT('Ctrl Pts',(10.0907382943461,27.7842139649744,-1.73964108221529));
#57277=CARTESIAN_POINT('Ctrl Pts',(10.7834515141013,27.7583882260773,-2.17179722470656));
#57278=CARTESIAN_POINT('Ctrl Pts',(11.7033986544081,27.6943968923929,-2.90904596552635));
#57279=CARTESIAN_POINT('Ctrl Pts',(12.1558218967572,27.647130029751,-3.30641843400165));
#57280=CARTESIAN_POINT('Ctrl Pts',(12.6542280666759,27.582969575709,-3.75198469320058));
#57281=CARTESIAN_POINT('Ctrl Pts',(13.1437548116734,27.5107186176355,-4.23653406986742));
#57282=CARTESIAN_POINT('Ctrl Pts',(14.1171239439967,27.3271714868175,-5.3520099831172));
#57283=CARTESIAN_POINT('Ctrl Pts',(14.8016839612719,27.1377343463863,-6.26369910268171));
#57284=CARTESIAN_POINT('Ctrl Pts',(15.5358005468912,26.8775022985013,-7.24012140721596));
#57285=CARTESIAN_POINT('Ctrl Pts',(16.0483854251272,26.6719324304959,-7.96755301690588));
#57286=CARTESIAN_POINT('Ctrl Pts',(17.0412489733341,26.1774693343013,-9.51866802157106));
#57287=CARTESIAN_POINT('Ctrl Pts',(17.7361882741502,25.7144627748922,-10.708934017746));
#57288=CARTESIAN_POINT('Ctrl Pts',(18.4727311807247,25.1427927030562,-11.9454322770708));
#57289=CARTESIAN_POINT('Ctrl Pts',(18.9926681482578,24.6948244944429,-12.856984892699));
#57290=CARTESIAN_POINT('Ctrl Pts',(19.993215775242,23.6653897614789,-14.7147792886911));
#57291=CARTESIAN_POINT('Ctrl Pts',(20.6988619738766,22.7591841007288,-16.0727729514956));
#57292=CARTESIAN_POINT('Ctrl Pts',(22.3925074251532,20.3625954625553,-19.1600243068367));
#57293=CARTESIAN_POINT('Ctrl Pts',(23.4934455914502,18.2609587529817,-21.14616843884));
#57294=CARTESIAN_POINT('Ctrl Pts',(24.4910863782171,15.7630437648442,-22.9288095711654));
#57295=CARTESIAN_POINT('Ctrl Pts',(2.09999999999999,34.805567674334,-0.9));
#57296=CARTESIAN_POINT('Ctrl Pts',(2.73333333333332,34.805567674334,-0.9));
#57297=CARTESIAN_POINT('Ctrl Pts',(3.36826743871256,34.8055967346523,-0.899835915143074));
#57298=CARTESIAN_POINT('Ctrl Pts',(4.12840588772228,34.8056056335578,-0.899790127261619));
#57299=CARTESIAN_POINT('Ctrl Pts',(4.4025114583892,34.8057820526053,-0.89490507727122));
#57300=CARTESIAN_POINT('Ctrl Pts',(4.91970796594585,34.8065669258982,-0.873924471880327));
#57301=CARTESIAN_POINT('Ctrl Pts',(5.79287353555174,34.8084012267811,-0.826944415738466));
#57302=CARTESIAN_POINT('Ctrl Pts',(6.46062808939426,34.8084327574831,-0.83018802637527));
#57303=CARTESIAN_POINT('Ctrl Pts',(6.92359088308148,34.8053357383561,-0.897514817877851));
#57304=CARTESIAN_POINT('Ctrl Pts',(7.04893740326678,34.804748375931,-0.916302103864695));
#57305=CARTESIAN_POINT('Ctrl Pts',(7.28704977969169,34.8039238169991,-0.954792702397151));
#57306=CARTESIAN_POINT('Ctrl Pts',(7.58724291600503,34.8033356004416,-1.00895581405421));
#57307=CARTESIAN_POINT('Ctrl Pts',(7.93954383598411,34.8025940050698,-1.08429063224267));
#57308=CARTESIAN_POINT('Ctrl Pts',(8.40075586732036,34.8006611522329,-1.20110613516639));
#57309=CARTESIAN_POINT('Ctrl Pts',(8.95399273182333,34.7946914626677,-1.38186135819649));
#57310=CARTESIAN_POINT('Ctrl Pts',(9.36427840538061,34.7827044460818,-1.57081212048793));
#57311=CARTESIAN_POINT('Ctrl Pts',(10.0148313303383,34.7542662135578,-1.92761296467034));
#57312=CARTESIAN_POINT('Ctrl Pts',(10.7126997709799,34.7263529856802,-2.47021587913641));
#57313=CARTESIAN_POINT('Ctrl Pts',(11.6386950163915,34.6527282846468,-3.39910531888624));
#57314=CARTESIAN_POINT('Ctrl Pts',(12.0933422150127,34.5969186241691,-3.89880693180439));
#57315=CARTESIAN_POINT('Ctrl Pts',(12.5933047205618,34.5203928739712,-4.45827819796938));
#57316=CARTESIAN_POINT('Ctrl Pts',(13.0908921604143,34.4332799259541,-5.07548512276185));
#57317=CARTESIAN_POINT('Ctrl Pts',(14.0727432149392,34.210693104137,-6.48656916810702));
#57318=CARTESIAN_POINT('Ctrl Pts',(14.7612503503968,33.9790719957191,-7.63560214898364));
#57319=CARTESIAN_POINT('Ctrl Pts',(15.4965030323713,33.6603033480339,-8.8605088817018));
#57320=CARTESIAN_POINT('Ctrl Pts',(16.014881454427,33.4054890971074,-9.78386054397124));
#57321=CARTESIAN_POINT('Ctrl Pts',(17.0125123260485,32.7936491966452,-11.7388593147722));
#57322=CARTESIAN_POINT('Ctrl Pts',(17.7100146172093,32.2196145267863,-13.2363029872184));
#57323=CARTESIAN_POINT('Ctrl Pts',(18.4472695543676,31.5115805969217,-14.7874452578874));
#57324=CARTESIAN_POINT('Ctrl Pts',(18.9707548965599,30.9524459159778,-15.9395047263215));
#57325=CARTESIAN_POINT('Ctrl Pts',(19.9740264837229,29.6706590049061,-18.2765031600774));
#57326=CARTESIAN_POINT('Ctrl Pts',(20.6810539289866,28.54203233395,-19.9829624932166));
#57327=CARTESIAN_POINT('Ctrl Pts',(22.3757767447239,25.5592752325617,-23.8579947070288));
#57328=CARTESIAN_POINT('Ctrl Pts',(23.4815899075194,22.9294129237493,-26.364359275229));
#57329=CARTESIAN_POINT('Ctrl Pts',(24.4815088739376,19.8034651938544,-28.6101490004946));
#57330=CARTESIAN_POINT('Ctrl Pts',(2.09999999999999,38.9897323410855,-0.9));
#57331=CARTESIAN_POINT('Ctrl Pts',(2.73333333333332,38.9897323410855,-0.9));
#57332=CARTESIAN_POINT('Ctrl Pts',(3.36849615379698,38.9897610649469,-0.899852059213593));
#57333=CARTESIAN_POINT('Ctrl Pts',(4.12885962395895,38.9897698170468,-0.899812187521165));
#57334=CARTESIAN_POINT('Ctrl Pts',(4.40583159898798,38.9899532662553,-0.894285767756435));
#57335=CARTESIAN_POINT('Ctrl Pts',(4.92485788889799,38.990768611501,-0.870670475322903));
#57336=CARTESIAN_POINT('Ctrl Pts',(5.79750326314279,38.9926765482163,-0.818103220835964));
#57337=CARTESIAN_POINT('Ctrl Pts',(6.45506243282504,38.992704760601,-0.822251386235662));
#57338=CARTESIAN_POINT('Ctrl Pts',(6.90763991463113,38.9894881916481,-0.895788682720272));
#57339=CARTESIAN_POINT('Ctrl Pts',(7.03283207401276,38.9888901159876,-0.91680271827912));
#57340=CARTESIAN_POINT('Ctrl Pts',(7.26916860321449,38.9880962384994,-0.959567402413746));
#57341=CARTESIAN_POINT('Ctrl Pts',(7.56737377775836,38.987619882036,-1.01979141838418));
#57342=CARTESIAN_POINT('Ctrl Pts',(7.91658095958571,38.9870532799917,-1.10336261682834));
#57343=CARTESIAN_POINT('Ctrl Pts',(8.37348791722709,38.9853096166242,-1.23286279651375));
#57344=CARTESIAN_POINT('Ctrl Pts',(8.92106444762905,38.9793115853919,-1.43302666782297));
#57345=CARTESIAN_POINT('Ctrl Pts',(9.32831366869251,38.9666594263059,-1.64284783605233));
#57346=CARTESIAN_POINT('Ctrl Pts',(9.97666156258205,38.936276009937,-2.04106314828367));
#57347=CARTESIAN_POINT('Ctrl Pts',(10.6788383765048,38.9069541794025,-2.65284302971923));
#57348=CARTESIAN_POINT('Ctrl Pts',(11.6082277531202,38.8272954085081,-3.69828340078152));
#57349=CARTESIAN_POINT('Ctrl Pts',(12.0641250472752,38.7662333808051,-4.25984491669686));
#57350=CARTESIAN_POINT('Ctrl Pts',(12.5649316129707,38.6821599570872,-4.88795818367918));
#57351=CARTESIAN_POINT('Ctrl Pts',(13.0665677015588,38.5858647600716,-5.58586750635022));
#57352=CARTESIAN_POINT('Ctrl Pts',(14.0523411482935,38.3394863474703,-7.17457852304705));
#57353=CARTESIAN_POINT('Ctrl Pts',(14.7427818946082,38.0822528719035,-8.4661717831259));
#57354=CARTESIAN_POINT('Ctrl Pts',(15.4785956174119,37.7280642874556,-9.84020415159883));
#57355=CARTESIAN_POINT('Ctrl Pts',(15.9996744207587,37.4434946991277,-10.8810259511239));
#57356=CARTESIAN_POINT('Ctrl Pts',(16.9995248066819,36.7608899240757,-13.0779693240867));
#57357=CARTESIAN_POINT('Ctrl Pts',(17.698187626898,36.1199220991796,-14.7595819219367));
#57358=CARTESIAN_POINT('Ctrl Pts',(18.4357383815742,35.3297290385984,-16.4993988315544));
#57359=CARTESIAN_POINT('Ctrl Pts',(18.9608457759147,34.7037521257359,-17.795429156587));
#57360=CARTESIAN_POINT('Ctrl Pts',(19.9653654503623,33.2702491455335,-20.4194610099597));
#57361=CARTESIAN_POINT('Ctrl Pts',(20.6729596776041,32.0078971340288,-22.3346914855994));
#57362=CARTESIAN_POINT('Ctrl Pts',(22.3680456304984,28.6727183627523,-26.6817849852975));
#57363=CARTESIAN_POINT('Ctrl Pts',(23.4757593035169,25.7258503646778,-29.4992019611683));
#57364=CARTESIAN_POINT('Ctrl Pts',(24.4767076204831,22.2231379796722,-32.0221667171178));
#57365=CARTESIAN_POINT('Ctrl Pts',(2.79759256767181,38.5299267367737,-0.89995268342482));
#57366=CARTESIAN_POINT('Ctrl Pts',(2.93204017151055,38.2166454242421,-0.899936609237971));
#57367=CARTESIAN_POINT('Ctrl Pts',(3.06669302905926,37.9029839075505,-0.899917784182059));
#57368=CARTESIAN_POINT('Ctrl Pts',(3.20139918604663,37.5892463829854,-0.899898741184433));
#57369=CARTESIAN_POINT('Origin',(0.249999999999999,0.,0.));
#57370=CARTESIAN_POINT('',(0.249999999999999,-38.75,-4.74550634669599E-15));
#57371=CARTESIAN_POINT('Origin',(2.9,0.,0.));
#57372=CARTESIAN_POINT('Origin',(27.1,0.,0.));
#57373=CARTESIAN_POINT('',(27.2,-8.7,-1.0654427152582E-15));
#57374=CARTESIAN_POINT('Origin',(27.2,0.,0.));
#57375=CARTESIAN_POINT('',(27.1,-8.95,-1.09605888523688E-15));
#57376=CARTESIAN_POINT('Origin',(28.8,0.,0.));
#57377=CARTESIAN_POINT('',(30.4,-8.7,-1.0654427152582E-15));
#57378=CARTESIAN_POINT('Origin',(30.4,0.,0.));
#57379=CARTESIAN_POINT('',(28.8,-8.7,-1.0654427152582E-15));
#57380=CARTESIAN_POINT('Origin',(30.7,0.,0.));
#57381=CARTESIAN_POINT('',(30.7,-8.4,-1.02870331128378E-15));
#60349=UNCERTAINTY_MEASURE_WITH_UNIT(LENGTH_MEASURE(0.01),#60366,
'DISTANCE_ACCURACY_VALUE',
'Maximum model space distance between geometric entities at asserted c
onnectivities');
#60353=UNCERTAINTY_MEASURE_WITH_UNIT(LENGTH_MEASURE(0.01),#60366,
'DISTANCE_ACCURACY_VALUE',
'Maximum model space distance between geometric entities at asserted c
onnectivities');
#60361=(
GEOMETRIC_REPRESENTATION_CONTEXT(3)
GLOBAL_UNCERTAINTY_ASSIGNED_CONTEXT((#60349))
GLOBAL_UNIT_ASSIGNED_CONTEXT((#60366,#60368,#60369))
REPRESENTATION_CONTEXT('','3D')
);
#60365=(
GEOMETRIC_REPRESENTATION_CONTEXT(3)
GLOBAL_UNCERTAINTY_ASSIGNED_CONTEXT((#60353))
GLOBAL_UNIT_ASSIGNED_CONTEXT((#60366,#60368,#60369))
REPRESENTATION_CONTEXT('','3D')
);
#60366=(
LENGTH_UNIT()
NAMED_UNIT(*)
SI_UNIT(.MILLI.,.METRE.)
);
#60368=(
NAMED_UNIT(*)
PLANE_ANGLE_UNIT()
SI_UNIT($,.RADIAN.)
);
#60369=(
NAMED_UNIT(*)
SI_UNIT($,.STERADIAN.)
SOLID_ANGLE_UNIT()
);
#60377=SHAPE_DEFINITION_REPRESENTATION(#60388,#60413);
#60388=PRODUCT_DEFINITION_SHAPE('',$,#60425);
#60413=SHAPE_REPRESENTATION('',(#19231),#60361);
#60417=PRODUCT_DEFINITION_CONTEXT('part definition',#60452,'design');
#60425=PRODUCT_DEFINITION('2026-10-25-00-06-36-701',
'09_Compressor_Wheel_54x78_7plus7',#60436,#60417);
#60436=PRODUCT_DEFINITION_FORMATION('',$,#60461);
#60452=APPLICATION_CONTEXT(
'Core Data for Automotive Mechanical Design Process');
#60453=PRODUCT_CONTEXT('part definition',#60452,'mechanical');
#60461=PRODUCT('2026-10-25-00-06-36-701',
'09_Compressor_Wheel_54x78_7plus7',$,(#60453));
#60514=COLOUR_RGB('Sky Blue',0.24,0.69,0.87);
#60515=FILL_AREA_STYLE_COLOUR('',#60514);
#60516=FILL_AREA_STYLE('',(#60515));
#60517=SURFACE_STYLE_FILL_AREA(#60516);
#60518=SURFACE_SIDE_STYLE('',(#60517));
#60519=SURFACE_STYLE_USAGE(.BOTH.,#60518);
#60520=PRESENTATION_STYLE_ASSIGNMENT((#60519));
ENDSEC;
END-ISO-10303-21;
